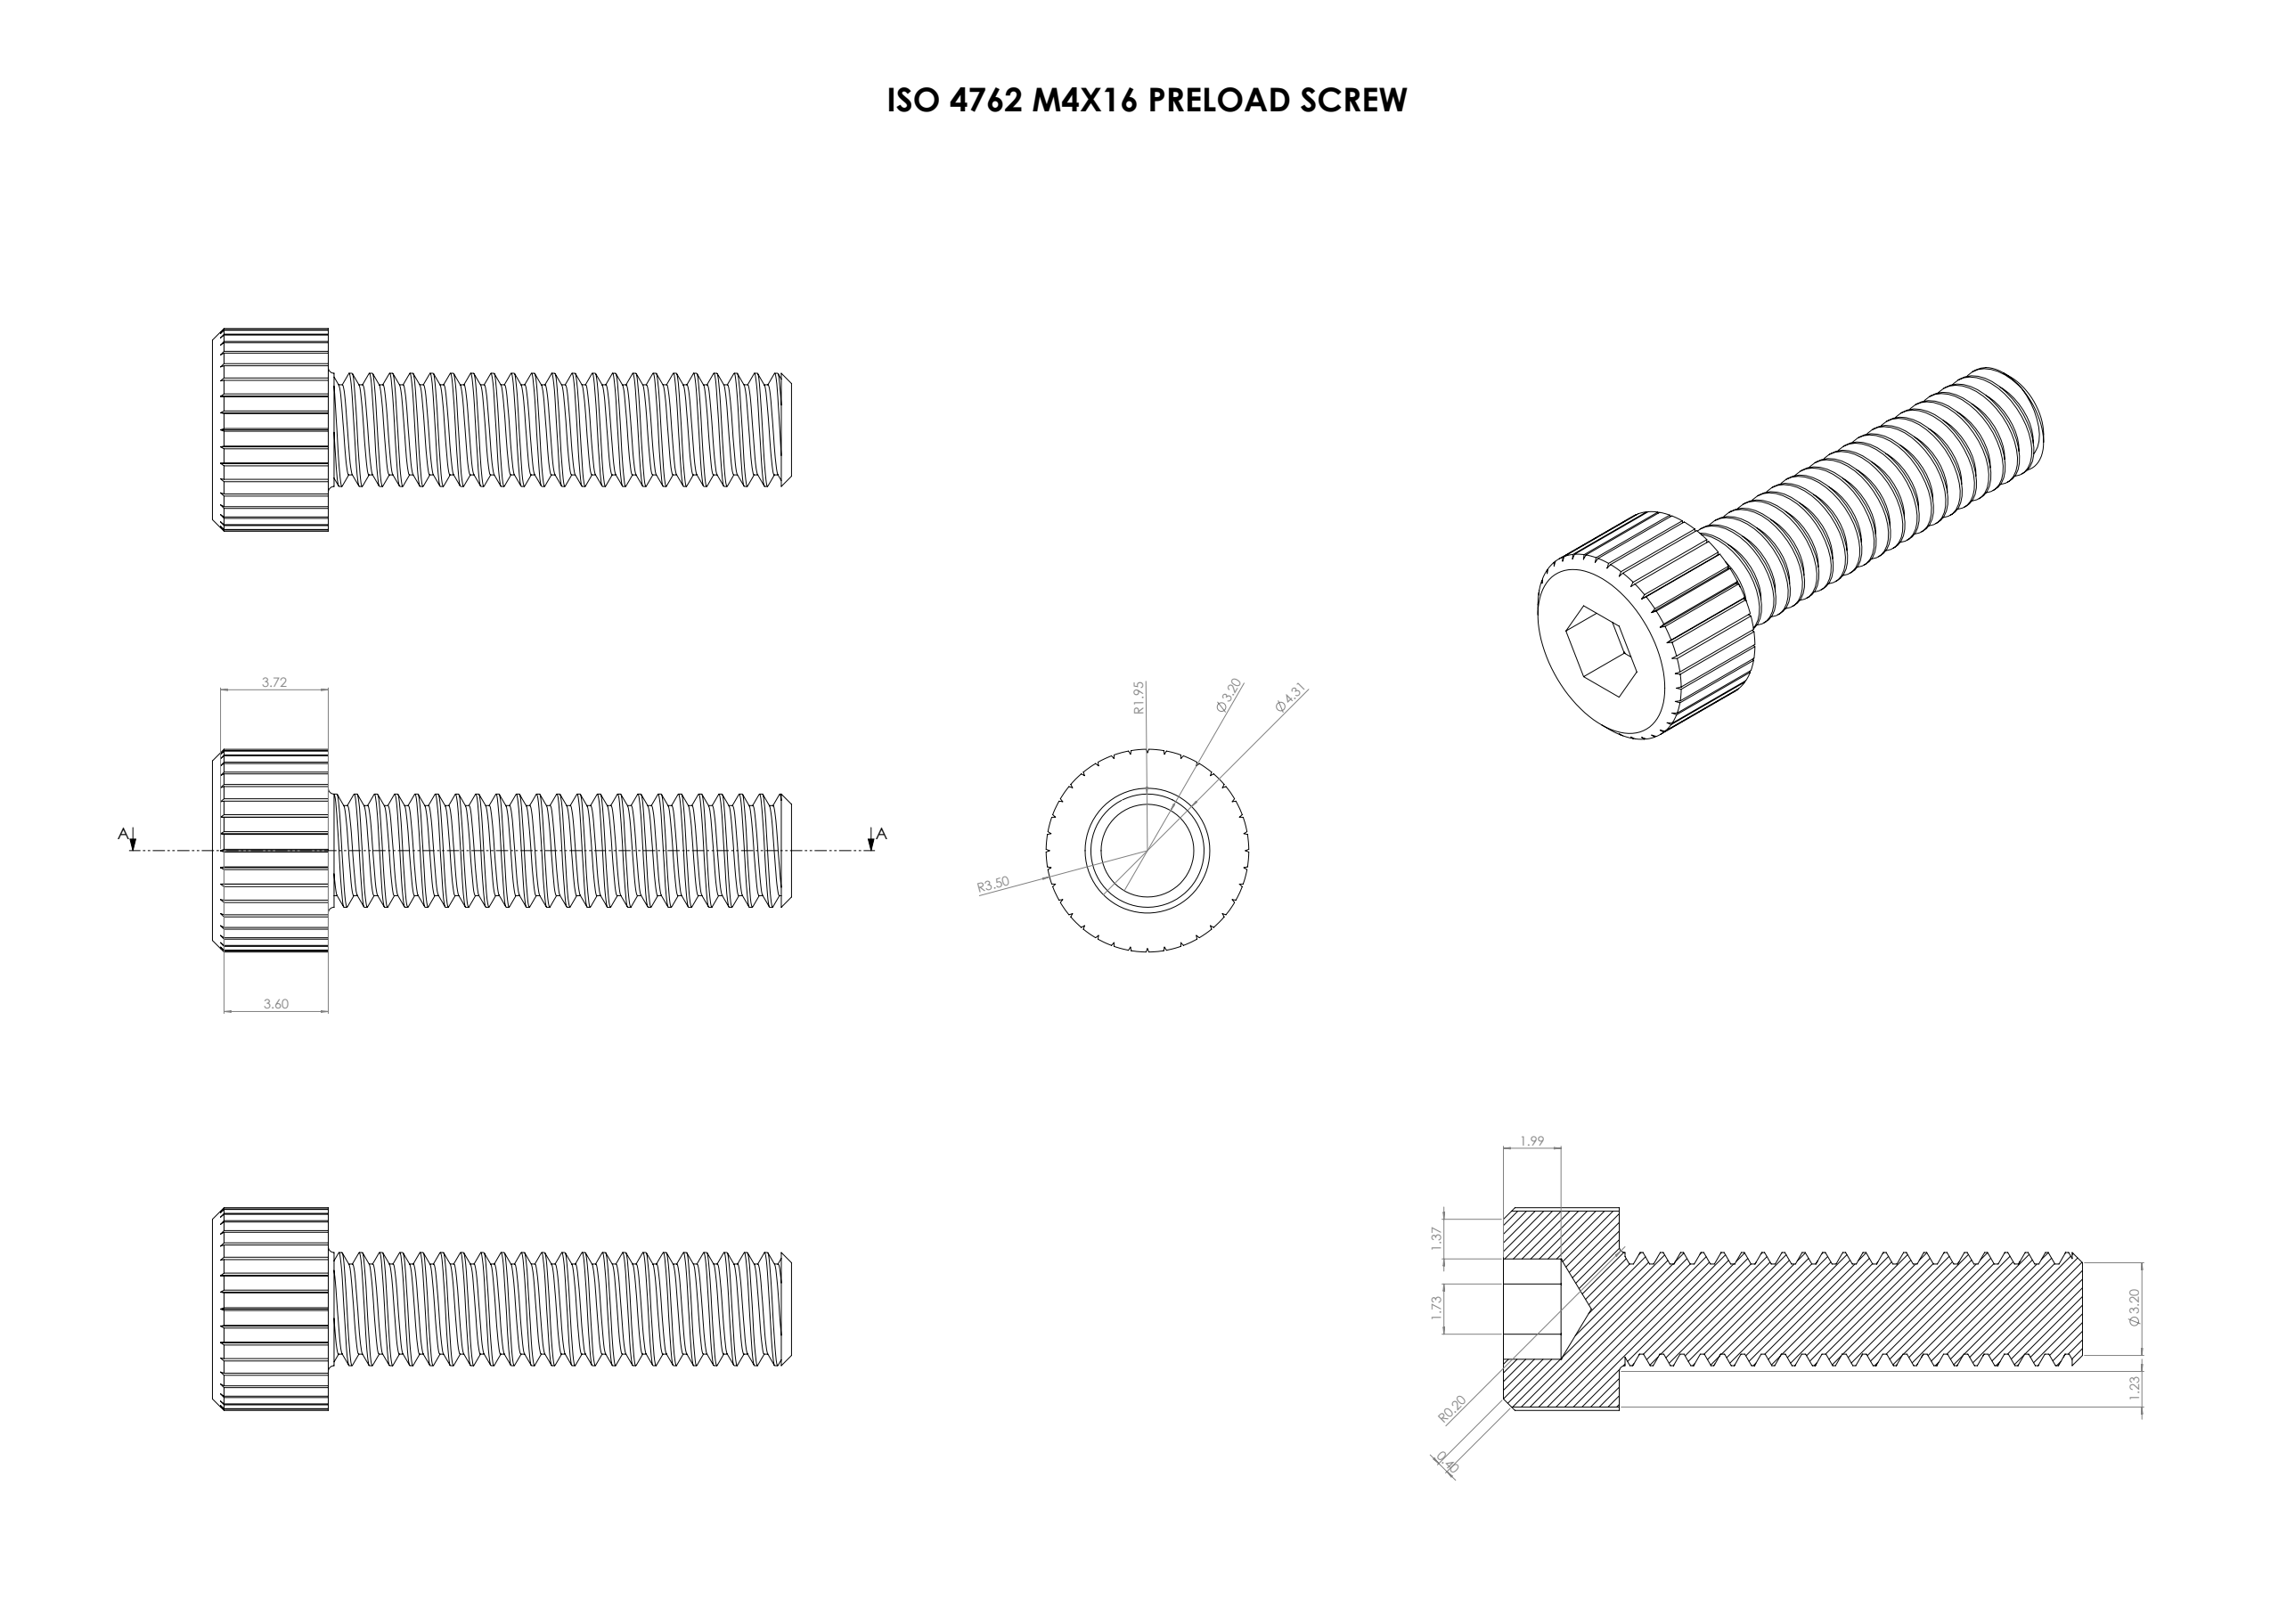
ISO-10303-21;
HEADER;
/* Generated by software containing ST-Developer
 * from STEP Tools, Inc. (www.steptools.com) 
 */

FILE_DESCRIPTION(
/* description */ (''),
/* implementation_level */ '2;1');

FILE_NAME(
/* name */ 
'11_ISO_4762_M4x16_Preload_Screw.step',
/* time_stamp */ '2026-10-20T10:06:23-07:00',
/* author */ (''),
/* organization */ (''),
/* preprocessor_version */ 'ST-DEVELOPER v20.2',
/* originating_system */ 'Autodesk Translation Framework v15.15.0.0',
/* authorisation */ '');

FILE_SCHEMA (('AUTOMOTIVE_DESIGN { 1 0 10303 214 3 1 1 }'));
ENDSEC;

DATA;
#10=MECHANICAL_DESIGN_GEOMETRIC_PRESENTATION_REPRESENTATION('',(#472),#38611);
#252=(
BOUNDED_CURVE()
B_SPLINE_CURVE(2,(#35550,#35551,#35552),.UNSPECIFIED.,.F.,.F.)
B_SPLINE_CURVE_WITH_KNOTS((3,3),(0.,0.00349669843186121),.UNSPECIFIED.)
CURVE()
GEOMETRIC_REPRESENTATION_ITEM()
RATIONAL_B_SPLINE_CURVE((1.,1.00004723091695,1.))
REPRESENTATION_ITEM('')
);
#253=(
BOUNDED_CURVE()
B_SPLINE_CURVE(2,(#35554,#35555,#35556),.UNSPECIFIED.,.F.,.F.)
B_SPLINE_CURVE_WITH_KNOTS((3,3),(0.,0.00349669843186122),.UNSPECIFIED.)
CURVE()
GEOMETRIC_REPRESENTATION_ITEM()
RATIONAL_B_SPLINE_CURVE((1.,1.00004723094136,1.))
REPRESENTATION_ITEM('')
);
#254=(
BOUNDED_CURVE()
B_SPLINE_CURVE(2,(#35559,#35560,#35561),.UNSPECIFIED.,.F.,.F.)
B_SPLINE_CURVE_WITH_KNOTS((3,3),(0.,0.00349669843186136),.UNSPECIFIED.)
CURVE()
GEOMETRIC_REPRESENTATION_ITEM()
RATIONAL_B_SPLINE_CURVE((1.,1.00004723092143,1.))
REPRESENTATION_ITEM('')
);
#255=(
BOUNDED_CURVE()
B_SPLINE_CURVE(2,(#35563,#35564,#35565),.UNSPECIFIED.,.F.,.F.)
B_SPLINE_CURVE_WITH_KNOTS((3,3),(0.,0.00349669843186135),.UNSPECIFIED.)
CURVE()
GEOMETRIC_REPRESENTATION_ITEM()
RATIONAL_B_SPLINE_CURVE((1.,1.00004723092493,1.))
REPRESENTATION_ITEM('')
);
#256=(
BOUNDED_CURVE()
B_SPLINE_CURVE(2,(#35568,#35569,#35570),.UNSPECIFIED.,.F.,.F.)
B_SPLINE_CURVE_WITH_KNOTS((3,3),(0.,0.00349669843186138),.UNSPECIFIED.)
CURVE()
GEOMETRIC_REPRESENTATION_ITEM()
RATIONAL_B_SPLINE_CURVE((1.,1.00004723092744,1.))
REPRESENTATION_ITEM('')
);
#257=(
BOUNDED_CURVE()
B_SPLINE_CURVE(2,(#35572,#35573,#35574),.UNSPECIFIED.,.F.,.F.)
B_SPLINE_CURVE_WITH_KNOTS((3,3),(0.,0.00349669843186141),.UNSPECIFIED.)
CURVE()
GEOMETRIC_REPRESENTATION_ITEM()
RATIONAL_B_SPLINE_CURVE((1.,1.00004723090855,1.))
REPRESENTATION_ITEM('')
);
#258=(
BOUNDED_CURVE()
B_SPLINE_CURVE(2,(#35577,#35578,#35579),.UNSPECIFIED.,.F.,.F.)
B_SPLINE_CURVE_WITH_KNOTS((3,3),(0.,0.0034966984318615),.UNSPECIFIED.)
CURVE()
GEOMETRIC_REPRESENTATION_ITEM()
RATIONAL_B_SPLINE_CURVE((1.,1.00004723094741,1.))
REPRESENTATION_ITEM('')
);
#259=(
BOUNDED_CURVE()
B_SPLINE_CURVE(2,(#35581,#35582,#35583),.UNSPECIFIED.,.F.,.F.)
B_SPLINE_CURVE_WITH_KNOTS((3,3),(0.,0.00349669843186142),.UNSPECIFIED.)
CURVE()
GEOMETRIC_REPRESENTATION_ITEM()
RATIONAL_B_SPLINE_CURVE((1.,1.00004723090666,1.))
REPRESENTATION_ITEM('')
);
#260=(
BOUNDED_CURVE()
B_SPLINE_CURVE(2,(#35586,#35587,#35588),.UNSPECIFIED.,.F.,.F.)
B_SPLINE_CURVE_WITH_KNOTS((3,3),(0.,0.00349669843186135),.UNSPECIFIED.)
CURVE()
GEOMETRIC_REPRESENTATION_ITEM()
RATIONAL_B_SPLINE_CURVE((1.,1.0000472309119,1.))
REPRESENTATION_ITEM('')
);
#261=(
BOUNDED_CURVE()
B_SPLINE_CURVE(2,(#35590,#35591,#35592),.UNSPECIFIED.,.F.,.F.)
B_SPLINE_CURVE_WITH_KNOTS((3,3),(0.,0.00349669843186137),.UNSPECIFIED.)
CURVE()
GEOMETRIC_REPRESENTATION_ITEM()
RATIONAL_B_SPLINE_CURVE((1.,1.00004723093721,1.))
REPRESENTATION_ITEM('')
);
#262=(
BOUNDED_CURVE()
B_SPLINE_CURVE(2,(#35595,#35596,#35597),.UNSPECIFIED.,.F.,.F.)
B_SPLINE_CURVE_WITH_KNOTS((3,3),(0.,0.00349669843186128),.UNSPECIFIED.)
CURVE()
GEOMETRIC_REPRESENTATION_ITEM()
RATIONAL_B_SPLINE_CURVE((1.,1.00004723093599,1.))
REPRESENTATION_ITEM('')
);
#263=(
BOUNDED_CURVE()
B_SPLINE_CURVE(2,(#35599,#35600,#35601),.UNSPECIFIED.,.F.,.F.)
B_SPLINE_CURVE_WITH_KNOTS((3,3),(0.,0.00349669843186128),.UNSPECIFIED.)
CURVE()
GEOMETRIC_REPRESENTATION_ITEM()
RATIONAL_B_SPLINE_CURVE((1.,1.00004723092625,1.))
REPRESENTATION_ITEM('')
);
#264=(
BOUNDED_CURVE()
B_SPLINE_CURVE(2,(#35672,#35673,#35674),.UNSPECIFIED.,.F.,.F.)
B_SPLINE_CURVE_WITH_KNOTS((3,3),(0.0420809670913651,0.0588848364681992),
 .UNSPECIFIED.)
CURVE()
GEOMETRIC_REPRESENTATION_ITEM()
RATIONAL_B_SPLINE_CURVE((1.00087707567824,1.00061365578614,1.))
REPRESENTATION_ITEM('')
);
#265=(
BOUNDED_CURVE()
B_SPLINE_CURVE(2,(#35679,#35680,#35681),.UNSPECIFIED.,.F.,.F.)
B_SPLINE_CURVE_WITH_KNOTS((3,3),(0.,0.0168038693768593),.UNSPECIFIED.)
CURVE()
GEOMETRIC_REPRESENTATION_ITEM()
RATIONAL_B_SPLINE_CURVE((1.,1.00061365578593,1.00087707567795))
REPRESENTATION_ITEM('')
);
#266=(
BOUNDED_CURVE()
B_SPLINE_CURVE(2,(#35686,#35687,#35688),.UNSPECIFIED.,.F.,.F.)
B_SPLINE_CURVE_WITH_KNOTS((3,3),(0.0420809670913399,0.0588848364681993),
 .UNSPECIFIED.)
CURVE()
GEOMETRIC_REPRESENTATION_ITEM()
RATIONAL_B_SPLINE_CURVE((1.00087707567746,1.00061365578559,1.))
REPRESENTATION_ITEM('')
);
#267=(
BOUNDED_CURVE()
B_SPLINE_CURVE(2,(#35693,#35694,#35695),.UNSPECIFIED.,.F.,.F.)
B_SPLINE_CURVE_WITH_KNOTS((3,3),(0.,0.0168038693768394),.UNSPECIFIED.)
CURVE()
GEOMETRIC_REPRESENTATION_ITEM()
RATIONAL_B_SPLINE_CURVE((1.,1.00061365578594,1.00087707567797))
REPRESENTATION_ITEM('')
);
#268=(
BOUNDED_CURVE()
B_SPLINE_CURVE(2,(#35700,#35701,#35702),.UNSPECIFIED.,.F.,.F.)
B_SPLINE_CURVE_WITH_KNOTS((3,3),(0.0420809670913626,0.0588848364681992),
 .UNSPECIFIED.)
CURVE()
GEOMETRIC_REPRESENTATION_ITEM()
RATIONAL_B_SPLINE_CURVE((1.00087707567775,1.00061365578579,1.))
REPRESENTATION_ITEM('')
);
#269=(
BOUNDED_CURVE()
B_SPLINE_CURVE(2,(#35707,#35708,#35709),.UNSPECIFIED.,.F.,.F.)
B_SPLINE_CURVE_WITH_KNOTS((3,3),(0.,0.0168038693768627),.UNSPECIFIED.)
CURVE()
GEOMETRIC_REPRESENTATION_ITEM()
RATIONAL_B_SPLINE_CURVE((1.,1.00061365578587,1.00087707567786))
REPRESENTATION_ITEM('')
);
#270=(
BOUNDED_CURVE()
B_SPLINE_CURVE(2,(#35714,#35715,#35716),.UNSPECIFIED.,.F.,.F.)
B_SPLINE_CURVE_WITH_KNOTS((3,3),(0.042080967091394,0.0588848364681993),
 .UNSPECIFIED.)
CURVE()
GEOMETRIC_REPRESENTATION_ITEM()
RATIONAL_B_SPLINE_CURVE((1.00087707567792,1.00061365578591,1.))
REPRESENTATION_ITEM('')
);
#271=(
BOUNDED_CURVE()
B_SPLINE_CURVE(2,(#35721,#35722,#35723),.UNSPECIFIED.,.F.,.F.)
B_SPLINE_CURVE_WITH_KNOTS((3,3),(0.,0.0168038693768566),.UNSPECIFIED.)
CURVE()
GEOMETRIC_REPRESENTATION_ITEM()
RATIONAL_B_SPLINE_CURVE((1.,1.00061365578555,1.0008770756774))
REPRESENTATION_ITEM('')
);
#272=(
BOUNDED_CURVE()
B_SPLINE_CURVE(2,(#35728,#35729,#35730),.UNSPECIFIED.,.F.,.F.)
B_SPLINE_CURVE_WITH_KNOTS((3,3),(0.0420809670913884,0.0588848364681993),
 .UNSPECIFIED.)
CURVE()
GEOMETRIC_REPRESENTATION_ITEM()
RATIONAL_B_SPLINE_CURVE((1.00087707567863,1.0006136557864,1.))
REPRESENTATION_ITEM('')
);
#273=(
BOUNDED_CURVE()
B_SPLINE_CURVE(2,(#35735,#35736,#35737),.UNSPECIFIED.,.F.,.F.)
B_SPLINE_CURVE_WITH_KNOTS((3,3),(0.,0.0168038693768499),.UNSPECIFIED.)
CURVE()
GEOMETRIC_REPRESENTATION_ITEM()
RATIONAL_B_SPLINE_CURVE((1.,1.00061365578631,1.00087707567849))
REPRESENTATION_ITEM('')
);
#274=(
BOUNDED_CURVE()
B_SPLINE_CURVE(2,(#35742,#35743,#35744),.UNSPECIFIED.,.F.,.F.)
B_SPLINE_CURVE_WITH_KNOTS((3,3),(0.0420809670913347,0.0588848364681992),
 .UNSPECIFIED.)
CURVE()
GEOMETRIC_REPRESENTATION_ITEM()
RATIONAL_B_SPLINE_CURVE((1.00087707567759,1.00061365578568,1.))
REPRESENTATION_ITEM('')
);
#275=(
BOUNDED_CURVE()
B_SPLINE_CURVE(2,(#35749,#35750,#35751),.UNSPECIFIED.,.F.,.F.)
B_SPLINE_CURVE_WITH_KNOTS((3,3),(0.,0.0168038693768258),.UNSPECIFIED.)
CURVE()
GEOMETRIC_REPRESENTATION_ITEM()
RATIONAL_B_SPLINE_CURVE((1.,1.00061365578592,1.00087707567793))
REPRESENTATION_ITEM('')
);
#276=(
BOUNDED_CURVE()
B_SPLINE_CURVE(2,(#35756,#35757,#35758),.UNSPECIFIED.,.F.,.F.)
B_SPLINE_CURVE_WITH_KNOTS((3,3),(0.0420809670913505,0.0588848364681993),
 .UNSPECIFIED.)
CURVE()
GEOMETRIC_REPRESENTATION_ITEM()
RATIONAL_B_SPLINE_CURVE((1.00087707567804,1.00061365578599,1.))
REPRESENTATION_ITEM('')
);
#277=(
BOUNDED_CURVE()
B_SPLINE_CURVE(2,(#35763,#35764,#35765),.UNSPECIFIED.,.F.,.F.)
B_SPLINE_CURVE_WITH_KNOTS((3,3),(0.,0.0168038693768362),.UNSPECIFIED.)
CURVE()
GEOMETRIC_REPRESENTATION_ITEM()
RATIONAL_B_SPLINE_CURVE((1.,1.00061365578568,1.00087707567759))
REPRESENTATION_ITEM('')
);
#278=(
BOUNDED_CURVE()
B_SPLINE_CURVE(2,(#35770,#35771,#35772),.UNSPECIFIED.,.F.,.F.)
B_SPLINE_CURVE_WITH_KNOTS((3,3),(0.0420809670913562,0.0588848364681992),
 .UNSPECIFIED.)
CURVE()
GEOMETRIC_REPRESENTATION_ITEM()
RATIONAL_B_SPLINE_CURVE((1.00087707567804,1.00061365578599,1.))
REPRESENTATION_ITEM('')
);
#279=(
BOUNDED_CURVE()
B_SPLINE_CURVE(2,(#35777,#35778,#35779),.UNSPECIFIED.,.F.,.F.)
B_SPLINE_CURVE_WITH_KNOTS((3,3),(0.,0.016803869376823),.UNSPECIFIED.)
CURVE()
GEOMETRIC_REPRESENTATION_ITEM()
RATIONAL_B_SPLINE_CURVE((1.,1.00061365578592,1.00087707567794))
REPRESENTATION_ITEM('')
);
#280=(
BOUNDED_CURVE()
B_SPLINE_CURVE(2,(#35784,#35785,#35786),.UNSPECIFIED.,.F.,.F.)
B_SPLINE_CURVE_WITH_KNOTS((3,3),(0.04208096709136,0.0588848364681992),
 .UNSPECIFIED.)
CURVE()
GEOMETRIC_REPRESENTATION_ITEM()
RATIONAL_B_SPLINE_CURVE((1.00087707567819,1.0006136557861,1.))
REPRESENTATION_ITEM('')
);
#281=(
BOUNDED_CURVE()
B_SPLINE_CURVE(2,(#35791,#35792,#35793),.UNSPECIFIED.,.F.,.F.)
B_SPLINE_CURVE_WITH_KNOTS((3,3),(0.,0.0168038693767949),.UNSPECIFIED.)
CURVE()
GEOMETRIC_REPRESENTATION_ITEM()
RATIONAL_B_SPLINE_CURVE((1.,1.00061365578653,1.00087707567881))
REPRESENTATION_ITEM('')
);
#282=(
BOUNDED_CURVE()
B_SPLINE_CURVE(2,(#35798,#35799,#35800),.UNSPECIFIED.,.F.,.F.)
B_SPLINE_CURVE_WITH_KNOTS((3,3),(0.0420809670913836,0.0588848364681992),
 .UNSPECIFIED.)
CURVE()
GEOMETRIC_REPRESENTATION_ITEM()
RATIONAL_B_SPLINE_CURVE((1.00087707567816,1.00061365578608,1.))
REPRESENTATION_ITEM('')
);
#283=(
BOUNDED_CURVE()
B_SPLINE_CURVE(2,(#35805,#35806,#35807),.UNSPECIFIED.,.F.,.F.)
B_SPLINE_CURVE_WITH_KNOTS((3,3),(0.,0.0168038693768179),.UNSPECIFIED.)
CURVE()
GEOMETRIC_REPRESENTATION_ITEM()
RATIONAL_B_SPLINE_CURVE((1.,1.00061365578613,1.00087707567823))
REPRESENTATION_ITEM('')
);
#284=(
BOUNDED_CURVE()
B_SPLINE_CURVE(2,(#35812,#35813,#35814),.UNSPECIFIED.,.F.,.F.)
B_SPLINE_CURVE_WITH_KNOTS((3,3),(0.0420809670913823,0.0588848364681992),
 .UNSPECIFIED.)
CURVE()
GEOMETRIC_REPRESENTATION_ITEM()
RATIONAL_B_SPLINE_CURVE((1.00087707567815,1.00061365578607,1.))
REPRESENTATION_ITEM('')
);
#285=(
BOUNDED_CURVE()
B_SPLINE_CURVE(2,(#35819,#35820,#35821),.UNSPECIFIED.,.F.,.F.)
B_SPLINE_CURVE_WITH_KNOTS((3,3),(0.,0.0168038693768011),.UNSPECIFIED.)
CURVE()
GEOMETRIC_REPRESENTATION_ITEM()
RATIONAL_B_SPLINE_CURVE((1.,1.00061365578643,1.00087707567867))
REPRESENTATION_ITEM('')
);
#286=(
BOUNDED_CURVE()
B_SPLINE_CURVE(2,(#35826,#35827,#35828),.UNSPECIFIED.,.F.,.F.)
B_SPLINE_CURVE_WITH_KNOTS((3,3),(0.0420809670914,0.0588848364681992),
 .UNSPECIFIED.)
CURVE()
GEOMETRIC_REPRESENTATION_ITEM()
RATIONAL_B_SPLINE_CURVE((1.00087707567851,1.00061365578632,1.))
REPRESENTATION_ITEM('')
);
#287=(
BOUNDED_CURVE()
B_SPLINE_CURVE(2,(#35833,#35834,#35835),.UNSPECIFIED.,.F.,.F.)
B_SPLINE_CURVE_WITH_KNOTS((3,3),(0.,0.016803869376813),.UNSPECIFIED.)
CURVE()
GEOMETRIC_REPRESENTATION_ITEM()
RATIONAL_B_SPLINE_CURVE((1.,1.00061365578622,1.00087707567836))
REPRESENTATION_ITEM('')
);
#288=(
BOUNDED_CURVE()
B_SPLINE_CURVE(2,(#35840,#35841,#35842),.UNSPECIFIED.,.F.,.F.)
B_SPLINE_CURVE_WITH_KNOTS((3,3),(0.0420809670913641,0.0588848364681993),
 .UNSPECIFIED.)
CURVE()
GEOMETRIC_REPRESENTATION_ITEM()
RATIONAL_B_SPLINE_CURVE((1.0008770756778,1.00061365578582,1.))
REPRESENTATION_ITEM('')
);
#289=(
BOUNDED_CURVE()
B_SPLINE_CURVE(2,(#35847,#35848,#35849),.UNSPECIFIED.,.F.,.F.)
B_SPLINE_CURVE_WITH_KNOTS((3,3),(0.,0.0168038693768258),.UNSPECIFIED.)
CURVE()
GEOMETRIC_REPRESENTATION_ITEM()
RATIONAL_B_SPLINE_CURVE((1.,1.00061365578608,1.00087707567816))
REPRESENTATION_ITEM('')
);
#290=(
BOUNDED_CURVE()
B_SPLINE_CURVE(2,(#35854,#35855,#35856),.UNSPECIFIED.,.F.,.F.)
B_SPLINE_CURVE_WITH_KNOTS((3,3),(0.0420809670913328,0.0588848364681992),
 .UNSPECIFIED.)
CURVE()
GEOMETRIC_REPRESENTATION_ITEM()
RATIONAL_B_SPLINE_CURVE((1.00087707567803,1.00061365578599,1.))
REPRESENTATION_ITEM('')
);
#291=(
BOUNDED_CURVE()
B_SPLINE_CURVE(2,(#35861,#35862,#35863),.UNSPECIFIED.,.F.,.F.)
B_SPLINE_CURVE_WITH_KNOTS((3,3),(0.,0.016803869376812),.UNSPECIFIED.)
CURVE()
GEOMETRIC_REPRESENTATION_ITEM()
RATIONAL_B_SPLINE_CURVE((1.,1.00061365578602,1.00087707567807))
REPRESENTATION_ITEM('')
);
#292=(
BOUNDED_CURVE()
B_SPLINE_CURVE(2,(#35868,#35869,#35870),.UNSPECIFIED.,.F.,.F.)
B_SPLINE_CURVE_WITH_KNOTS((3,3),(0.0420809670913778,0.0588848364681992),
 .UNSPECIFIED.)
CURVE()
GEOMETRIC_REPRESENTATION_ITEM()
RATIONAL_B_SPLINE_CURVE((1.0008770756785,1.00061365578631,1.))
REPRESENTATION_ITEM('')
);
#293=(
BOUNDED_CURVE()
B_SPLINE_CURVE(2,(#35875,#35876,#35877),.UNSPECIFIED.,.F.,.F.)
B_SPLINE_CURVE_WITH_KNOTS((3,3),(0.,0.0168038693768374),.UNSPECIFIED.)
CURVE()
GEOMETRIC_REPRESENTATION_ITEM()
RATIONAL_B_SPLINE_CURVE((1.,1.00061365578616,1.00087707567828))
REPRESENTATION_ITEM('')
);
#294=(
BOUNDED_CURVE()
B_SPLINE_CURVE(2,(#35882,#35883,#35884),.UNSPECIFIED.,.F.,.F.)
B_SPLINE_CURVE_WITH_KNOTS((3,3),(0.0420809670913638,0.0588848364681993),
 .UNSPECIFIED.)
CURVE()
GEOMETRIC_REPRESENTATION_ITEM()
RATIONAL_B_SPLINE_CURVE((1.00087707567787,1.00061365578588,1.))
REPRESENTATION_ITEM('')
);
#295=(
BOUNDED_CURVE()
B_SPLINE_CURVE(2,(#35889,#35890,#35891),.UNSPECIFIED.,.F.,.F.)
B_SPLINE_CURVE_WITH_KNOTS((3,3),(0.,0.0168038693768215),.UNSPECIFIED.)
CURVE()
GEOMETRIC_REPRESENTATION_ITEM()
RATIONAL_B_SPLINE_CURVE((1.,1.00061365578602,1.00087707567808))
REPRESENTATION_ITEM('')
);
#296=(
BOUNDED_CURVE()
B_SPLINE_CURVE(2,(#35896,#35897,#35898),.UNSPECIFIED.,.F.,.F.)
B_SPLINE_CURVE_WITH_KNOTS((3,3),(0.0420809670913305,0.0588848364681993),
 .UNSPECIFIED.)
CURVE()
GEOMETRIC_REPRESENTATION_ITEM()
RATIONAL_B_SPLINE_CURVE((1.00087707567765,1.00061365578572,1.))
REPRESENTATION_ITEM('')
);
#297=(
BOUNDED_CURVE()
B_SPLINE_CURVE(2,(#35903,#35904,#35905),.UNSPECIFIED.,.F.,.F.)
B_SPLINE_CURVE_WITH_KNOTS((3,3),(0.,0.0168038693768224),.UNSPECIFIED.)
CURVE()
GEOMETRIC_REPRESENTATION_ITEM()
RATIONAL_B_SPLINE_CURVE((1.,1.00061365578599,1.00087707567803))
REPRESENTATION_ITEM('')
);
#298=(
BOUNDED_CURVE()
B_SPLINE_CURVE(2,(#35910,#35911,#35912),.UNSPECIFIED.,.F.,.F.)
B_SPLINE_CURVE_WITH_KNOTS((3,3),(0.0420809670913736,0.0588848364681993),
 .UNSPECIFIED.)
CURVE()
GEOMETRIC_REPRESENTATION_ITEM()
RATIONAL_B_SPLINE_CURVE((1.00087707567727,1.00061365578546,1.))
REPRESENTATION_ITEM('')
);
#299=(
BOUNDED_CURVE()
B_SPLINE_CURVE(2,(#35917,#35918,#35919),.UNSPECIFIED.,.F.,.F.)
B_SPLINE_CURVE_WITH_KNOTS((3,3),(0.,0.0168038693768305),.UNSPECIFIED.)
CURVE()
GEOMETRIC_REPRESENTATION_ITEM()
RATIONAL_B_SPLINE_CURVE((1.,1.00061365578611,1.00087707567821))
REPRESENTATION_ITEM('')
);
#300=(
BOUNDED_CURVE()
B_SPLINE_CURVE(2,(#35924,#35925,#35926),.UNSPECIFIED.,.F.,.F.)
B_SPLINE_CURVE_WITH_KNOTS((3,3),(0.042080967091357,0.0588848364681993),
 .UNSPECIFIED.)
CURVE()
GEOMETRIC_REPRESENTATION_ITEM()
RATIONAL_B_SPLINE_CURVE((1.00087707567817,1.00061365578609,1.))
REPRESENTATION_ITEM('')
);
#301=(
BOUNDED_CURVE()
B_SPLINE_CURVE(2,(#35931,#35932,#35933),.UNSPECIFIED.,.F.,.F.)
B_SPLINE_CURVE_WITH_KNOTS((3,3),(0.,0.0168038693768215),.UNSPECIFIED.)
CURVE()
GEOMETRIC_REPRESENTATION_ITEM()
RATIONAL_B_SPLINE_CURVE((1.,1.00061365578616,1.00087707567828))
REPRESENTATION_ITEM('')
);
#302=(
BOUNDED_CURVE()
B_SPLINE_CURVE(2,(#35938,#35939,#35940),.UNSPECIFIED.,.F.,.F.)
B_SPLINE_CURVE_WITH_KNOTS((3,3),(0.04208096709137,0.0588848364681993),
 .UNSPECIFIED.)
CURVE()
GEOMETRIC_REPRESENTATION_ITEM()
RATIONAL_B_SPLINE_CURVE((1.00087707567792,1.00061365578591,1.))
REPRESENTATION_ITEM('')
);
#303=(
BOUNDED_CURVE()
B_SPLINE_CURVE(2,(#35945,#35946,#35947),.UNSPECIFIED.,.F.,.F.)
B_SPLINE_CURVE_WITH_KNOTS((3,3),(0.,0.0168038693768075),.UNSPECIFIED.)
CURVE()
GEOMETRIC_REPRESENTATION_ITEM()
RATIONAL_B_SPLINE_CURVE((1.,1.00061365578628,1.00087707567845))
REPRESENTATION_ITEM('')
);
#304=(
BOUNDED_CURVE()
B_SPLINE_CURVE(2,(#35952,#35953,#35954),.UNSPECIFIED.,.F.,.F.)
B_SPLINE_CURVE_WITH_KNOTS((3,3),(0.0420809670913788,0.0588848364681993),
 .UNSPECIFIED.)
CURVE()
GEOMETRIC_REPRESENTATION_ITEM()
RATIONAL_B_SPLINE_CURVE((1.00087707567806,1.00061365578601,1.))
REPRESENTATION_ITEM('')
);
#305=(
BOUNDED_CURVE()
B_SPLINE_CURVE(2,(#35959,#35960,#35961),.UNSPECIFIED.,.F.,.F.)
B_SPLINE_CURVE_WITH_KNOTS((3,3),(0.,0.0168038693768069),.UNSPECIFIED.)
CURVE()
GEOMETRIC_REPRESENTATION_ITEM()
RATIONAL_B_SPLINE_CURVE((1.,1.00061365578667,1.000877075679))
REPRESENTATION_ITEM('')
);
#306=(
BOUNDED_CURVE()
B_SPLINE_CURVE(2,(#35966,#35967,#35968),.UNSPECIFIED.,.F.,.F.)
B_SPLINE_CURVE_WITH_KNOTS((3,3),(0.0420809670913639,0.0588848364681993),
 .UNSPECIFIED.)
CURVE()
GEOMETRIC_REPRESENTATION_ITEM()
RATIONAL_B_SPLINE_CURVE((1.00087707567811,1.00061365578604,1.))
REPRESENTATION_ITEM('')
);
#307=(
BOUNDED_CURVE()
B_SPLINE_CURVE(2,(#35973,#35974,#35975),.UNSPECIFIED.,.F.,.F.)
B_SPLINE_CURVE_WITH_KNOTS((3,3),(0.,0.0168038693768441),.UNSPECIFIED.)
CURVE()
GEOMETRIC_REPRESENTATION_ITEM()
RATIONAL_B_SPLINE_CURVE((1.,1.00061365578625,1.0008770756784))
REPRESENTATION_ITEM('')
);
#308=(
BOUNDED_CURVE()
B_SPLINE_CURVE(2,(#35980,#35981,#35982),.UNSPECIFIED.,.F.,.F.)
B_SPLINE_CURVE_WITH_KNOTS((3,3),(0.0420809670913765,0.0588848364681993),
 .UNSPECIFIED.)
CURVE()
GEOMETRIC_REPRESENTATION_ITEM()
RATIONAL_B_SPLINE_CURVE((1.00087707567789,1.00061365578589,1.))
REPRESENTATION_ITEM('')
);
#309=(
BOUNDED_CURVE()
B_SPLINE_CURVE(2,(#35987,#35988,#35989),.UNSPECIFIED.,.F.,.F.)
B_SPLINE_CURVE_WITH_KNOTS((3,3),(0.,0.016803869376822),.UNSPECIFIED.)
CURVE()
GEOMETRIC_REPRESENTATION_ITEM()
RATIONAL_B_SPLINE_CURVE((1.,1.00061365578656,1.00087707567884))
REPRESENTATION_ITEM('')
);
#310=(
BOUNDED_CURVE()
B_SPLINE_CURVE(2,(#35994,#35995,#35996),.UNSPECIFIED.,.F.,.F.)
B_SPLINE_CURVE_WITH_KNOTS((3,3),(0.0420809670913437,0.0588848364681993),
 .UNSPECIFIED.)
CURVE()
GEOMETRIC_REPRESENTATION_ITEM()
RATIONAL_B_SPLINE_CURVE((1.00087707567775,1.00061365578579,1.))
REPRESENTATION_ITEM('')
);
#311=(
BOUNDED_CURVE()
B_SPLINE_CURVE(2,(#36001,#36002,#36003),.UNSPECIFIED.,.F.,.F.)
B_SPLINE_CURVE_WITH_KNOTS((3,3),(0.,0.0168038693768237),.UNSPECIFIED.)
CURVE()
GEOMETRIC_REPRESENTATION_ITEM()
RATIONAL_B_SPLINE_CURVE((1.,1.00061365578586,1.00087707567785))
REPRESENTATION_ITEM('')
);
#312=(
BOUNDED_CURVE()
B_SPLINE_CURVE(2,(#36008,#36009,#36010),.UNSPECIFIED.,.F.,.F.)
B_SPLINE_CURVE_WITH_KNOTS((3,3),(0.0420809670913633,0.0588848364681993),
 .UNSPECIFIED.)
CURVE()
GEOMETRIC_REPRESENTATION_ITEM()
RATIONAL_B_SPLINE_CURVE((1.00087707567797,1.00061365578594,1.))
REPRESENTATION_ITEM('')
);
#313=(
BOUNDED_CURVE()
B_SPLINE_CURVE(2,(#36015,#36016,#36017),.UNSPECIFIED.,.F.,.F.)
B_SPLINE_CURVE_WITH_KNOTS((3,3),(0.,0.0168038693768391),.UNSPECIFIED.)
CURVE()
GEOMETRIC_REPRESENTATION_ITEM()
RATIONAL_B_SPLINE_CURVE((1.,1.00061365578625,1.0008770756784))
REPRESENTATION_ITEM('')
);
#314=(
BOUNDED_CURVE()
B_SPLINE_CURVE(2,(#36022,#36023,#36024),.UNSPECIFIED.,.F.,.F.)
B_SPLINE_CURVE_WITH_KNOTS((3,3),(0.0420809670913792,0.0588848364681992),
 .UNSPECIFIED.)
CURVE()
GEOMETRIC_REPRESENTATION_ITEM()
RATIONAL_B_SPLINE_CURVE((1.00087707567848,1.0006136557863,1.))
REPRESENTATION_ITEM('')
);
#315=(
BOUNDED_CURVE()
B_SPLINE_CURVE(2,(#36029,#36030,#36031),.UNSPECIFIED.,.F.,.F.)
B_SPLINE_CURVE_WITH_KNOTS((3,3),(0.,0.0168038693768203),.UNSPECIFIED.)
CURVE()
GEOMETRIC_REPRESENTATION_ITEM()
RATIONAL_B_SPLINE_CURVE((1.,1.00061365578598,1.00087707567802))
REPRESENTATION_ITEM('')
);
#316=(
BOUNDED_CURVE()
B_SPLINE_CURVE(2,(#36036,#36037,#36038),.UNSPECIFIED.,.F.,.F.)
B_SPLINE_CURVE_WITH_KNOTS((3,3),(0.0420809670913809,0.0588848364681992),
 .UNSPECIFIED.)
CURVE()
GEOMETRIC_REPRESENTATION_ITEM()
RATIONAL_B_SPLINE_CURVE((1.00087707567876,1.0006136557865,1.))
REPRESENTATION_ITEM('')
);
#317=(
BOUNDED_CURVE()
B_SPLINE_CURVE(2,(#36043,#36044,#36045),.UNSPECIFIED.,.F.,.F.)
B_SPLINE_CURVE_WITH_KNOTS((3,3),(0.,0.016803869376822),.UNSPECIFIED.)
CURVE()
GEOMETRIC_REPRESENTATION_ITEM()
RATIONAL_B_SPLINE_CURVE((1.,1.00061365578629,1.00087707567847))
REPRESENTATION_ITEM('')
);
#318=(
BOUNDED_CURVE()
B_SPLINE_CURVE(2,(#36050,#36051,#36052),.UNSPECIFIED.,.F.,.F.)
B_SPLINE_CURVE_WITH_KNOTS((3,3),(0.0420809670913693,0.0588848364681992),
 .UNSPECIFIED.)
CURVE()
GEOMETRIC_REPRESENTATION_ITEM()
RATIONAL_B_SPLINE_CURVE((1.00087707567787,1.00061365578588,1.))
REPRESENTATION_ITEM('')
);
#319=(
BOUNDED_CURVE()
B_SPLINE_CURVE(2,(#36057,#36058,#36059),.UNSPECIFIED.,.F.,.F.)
B_SPLINE_CURVE_WITH_KNOTS((3,3),(0.,0.0168038693768241),.UNSPECIFIED.)
CURVE()
GEOMETRIC_REPRESENTATION_ITEM()
RATIONAL_B_SPLINE_CURVE((1.,1.00061365578674,1.00087707567911))
REPRESENTATION_ITEM('')
);
#320=(
BOUNDED_CURVE()
B_SPLINE_CURVE(2,(#36064,#36065,#36066),.UNSPECIFIED.,.F.,.F.)
B_SPLINE_CURVE_WITH_KNOTS((3,3),(0.0420809670913706,0.0588848364681992),
 .UNSPECIFIED.)
CURVE()
GEOMETRIC_REPRESENTATION_ITEM()
RATIONAL_B_SPLINE_CURVE((1.00087707567803,1.00061365578598,1.))
REPRESENTATION_ITEM('')
);
#321=(
BOUNDED_CURVE()
B_SPLINE_CURVE(2,(#36071,#36072,#36073),.UNSPECIFIED.,.F.,.F.)
B_SPLINE_CURVE_WITH_KNOTS((3,3),(0.,0.0168038693768352),.UNSPECIFIED.)
CURVE()
GEOMETRIC_REPRESENTATION_ITEM()
RATIONAL_B_SPLINE_CURVE((1.,1.00061365578544,1.00087707567725))
REPRESENTATION_ITEM('')
);
#322=(
BOUNDED_CURVE()
B_SPLINE_CURVE(2,(#36078,#36079,#36080),.UNSPECIFIED.,.F.,.F.)
B_SPLINE_CURVE_WITH_KNOTS((3,3),(0.0420809670913822,0.0588848364681993),
 .UNSPECIFIED.)
CURVE()
GEOMETRIC_REPRESENTATION_ITEM()
RATIONAL_B_SPLINE_CURVE((1.00087707567791,1.00061365578591,1.))
REPRESENTATION_ITEM('')
);
#323=(
BOUNDED_CURVE()
B_SPLINE_CURVE(2,(#36085,#36086,#36087),.UNSPECIFIED.,.F.,.F.)
B_SPLINE_CURVE_WITH_KNOTS((3,3),(0.,0.0168038693768391),.UNSPECIFIED.)
CURVE()
GEOMETRIC_REPRESENTATION_ITEM()
RATIONAL_B_SPLINE_CURVE((1.,1.00061365578625,1.0008770756784))
REPRESENTATION_ITEM('')
);
#324=(
BOUNDED_CURVE()
B_SPLINE_CURVE(2,(#36092,#36093,#36094),.UNSPECIFIED.,.F.,.F.)
B_SPLINE_CURVE_WITH_KNOTS((3,3),(0.0420809670913788,0.0588848364681992),
 .UNSPECIFIED.)
CURVE()
GEOMETRIC_REPRESENTATION_ITEM()
RATIONAL_B_SPLINE_CURVE((1.00087707567811,1.00061365578604,1.))
REPRESENTATION_ITEM('')
);
#325=(
BOUNDED_CURVE()
B_SPLINE_CURVE(2,(#36099,#36100,#36101),.UNSPECIFIED.,.F.,.F.)
B_SPLINE_CURVE_WITH_KNOTS((3,3),(0.,0.0168038693768716),.UNSPECIFIED.)
CURVE()
GEOMETRIC_REPRESENTATION_ITEM()
RATIONAL_B_SPLINE_CURVE((1.,1.00061365578607,1.00087707567815))
REPRESENTATION_ITEM('')
);
#326=(
BOUNDED_CURVE()
B_SPLINE_CURVE(2,(#36106,#36107,#36108),.UNSPECIFIED.,.F.,.F.)
B_SPLINE_CURVE_WITH_KNOTS((3,3),(0.0420809670913493,0.0588848364681993),
 .UNSPECIFIED.)
CURVE()
GEOMETRIC_REPRESENTATION_ITEM()
RATIONAL_B_SPLINE_CURVE((1.00087707567838,1.00061365578623,1.))
REPRESENTATION_ITEM('')
);
#327=(
BOUNDED_CURVE()
B_SPLINE_CURVE(2,(#36113,#36114,#36115),.UNSPECIFIED.,.F.,.F.)
B_SPLINE_CURVE_WITH_KNOTS((3,3),(0.,0.0168038693768289),.UNSPECIFIED.)
CURVE()
GEOMETRIC_REPRESENTATION_ITEM()
RATIONAL_B_SPLINE_CURVE((1.,1.00061365578616,1.00087707567828))
REPRESENTATION_ITEM('')
);
#328=(
BOUNDED_CURVE()
B_SPLINE_CURVE(2,(#36120,#36121,#36122),.UNSPECIFIED.,.F.,.F.)
B_SPLINE_CURVE_WITH_KNOTS((3,3),(0.0420809670913749,0.0588848364681992),
 .UNSPECIFIED.)
CURVE()
GEOMETRIC_REPRESENTATION_ITEM()
RATIONAL_B_SPLINE_CURVE((1.00087707567811,1.00061365578604,1.))
REPRESENTATION_ITEM('')
);
#329=(
BOUNDED_CURVE()
B_SPLINE_CURVE(2,(#36127,#36128,#36129),.UNSPECIFIED.,.F.,.F.)
B_SPLINE_CURVE_WITH_KNOTS((3,3),(0.,0.0168038693768264),.UNSPECIFIED.)
CURVE()
GEOMETRIC_REPRESENTATION_ITEM()
RATIONAL_B_SPLINE_CURVE((1.,1.00061365578613,1.00087707567823))
REPRESENTATION_ITEM('')
);
#330=(
BOUNDED_CURVE()
B_SPLINE_CURVE(2,(#36134,#36135,#36136),.UNSPECIFIED.,.F.,.F.)
B_SPLINE_CURVE_WITH_KNOTS((3,3),(0.0420809670913744,0.0588848364681992),
 .UNSPECIFIED.)
CURVE()
GEOMETRIC_REPRESENTATION_ITEM()
RATIONAL_B_SPLINE_CURVE((1.00087707567875,1.00061365578649,1.))
REPRESENTATION_ITEM('')
);
#331=(
BOUNDED_CURVE()
B_SPLINE_CURVE(2,(#36141,#36142,#36143),.UNSPECIFIED.,.F.,.F.)
B_SPLINE_CURVE_WITH_KNOTS((3,3),(0.,0.0168038693768507),.UNSPECIFIED.)
CURVE()
GEOMETRIC_REPRESENTATION_ITEM()
RATIONAL_B_SPLINE_CURVE((1.,1.00061365578591,1.00087707567792))
REPRESENTATION_ITEM('')
);
#332=(
BOUNDED_CURVE()
B_SPLINE_CURVE(2,(#36148,#36149,#36150),.UNSPECIFIED.,.F.,.F.)
B_SPLINE_CURVE_WITH_KNOTS((3,3),(0.0420809670913786,0.0588848364681993),
 .UNSPECIFIED.)
CURVE()
GEOMETRIC_REPRESENTATION_ITEM()
RATIONAL_B_SPLINE_CURVE((1.00087707567801,1.00061365578597,1.))
REPRESENTATION_ITEM('')
);
#333=(
BOUNDED_CURVE()
B_SPLINE_CURVE(2,(#36155,#36156,#36157),.UNSPECIFIED.,.F.,.F.)
B_SPLINE_CURVE_WITH_KNOTS((3,3),(0.,0.0168038693768258),.UNSPECIFIED.)
CURVE()
GEOMETRIC_REPRESENTATION_ITEM()
RATIONAL_B_SPLINE_CURVE((1.,1.00061365578592,1.00087707567793))
REPRESENTATION_ITEM('')
);
#334=(
BOUNDED_CURVE()
B_SPLINE_CURVE(2,(#36162,#36163,#36164),.UNSPECIFIED.,.F.,.F.)
B_SPLINE_CURVE_WITH_KNOTS((3,3),(0.0420809670913652,0.0588848364681993),
 .UNSPECIFIED.)
CURVE()
GEOMETRIC_REPRESENTATION_ITEM()
RATIONAL_B_SPLINE_CURVE((1.00087707567844,1.00061365578627,1.))
REPRESENTATION_ITEM('')
);
#335=(
BOUNDED_CURVE()
B_SPLINE_CURVE(2,(#36169,#36170,#36171),.UNSPECIFIED.,.F.,.F.)
B_SPLINE_CURVE_WITH_KNOTS((3,3),(0.,0.0168038693768152),.UNSPECIFIED.)
CURVE()
GEOMETRIC_REPRESENTATION_ITEM()
RATIONAL_B_SPLINE_CURVE((1.,1.00061365578615,1.00087707567826))
REPRESENTATION_ITEM('')
);
#444=SHAPE_REPRESENTATION_RELATIONSHIP('SRR','None',#38680,#458);
#458=ADVANCED_BREP_SHAPE_REPRESENTATION('',(#486),#38609);
#472=STYLED_ITEM('',(#38885),#486);
#486=MANIFOLD_SOLID_BREP('Screw',#16246);
#489=TOROIDAL_SURFACE('',#17387,0.2154,0.02);
#506=B_SPLINE_SURFACE_WITH_KNOTS('',3,3,((#33981,#33982,#33983,#33984,#33985,
#33986,#33987,#33988,#33989,#33990,#33991,#33992,#33993,#33994,#33995,#33996,
#33997,#33998,#33999,#34000,#34001,#34002,#34003,#34004,#34005,#34006,#34007,
#34008,#34009,#34010,#34011,#34012,#34013,#34014,#34015,#34016,#34017,#34018,
#34019,#34020,#34021,#34022,#34023,#34024,#34025,#34026,#34027,#34028,#34029,
#34030,#34031,#34032,#34033,#34034,#34035,#34036,#34037,#34038,#34039,#34040,
#34041,#34042,#34043,#34044,#34045,#34046,#34047,#34048,#34049,#34050,#34051,
#34052,#34053,#34054,#34055,#34056,#34057,#34058,#34059,#34060,#34061,#34062,
#34063,#34064,#34065,#34066,#34067,#34068,#34069,#34070,#34071,#34072,#34073,
#34074,#34075,#34076,#34077,#34078,#34079,#34080,#34081,#34082,#34083,#34084,
#34085,#34086,#34087,#34088,#34089,#34090,#34091,#34092,#34093,#34094,#34095,
#34096,#34097,#34098,#34099,#34100,#34101,#34102,#34103,#34104,#34105,#34106,
#34107,#34108,#34109,#34110,#34111,#34112,#34113,#34114,#34115,#34116,#34117,
#34118,#34119,#34120,#34121,#34122,#34123,#34124),(#34125,#34126,#34127,
#34128,#34129,#34130,#34131,#34132,#34133,#34134,#34135,#34136,#34137,#34138,
#34139,#34140,#34141,#34142,#34143,#34144,#34145,#34146,#34147,#34148,#34149,
#34150,#34151,#34152,#34153,#34154,#34155,#34156,#34157,#34158,#34159,#34160,
#34161,#34162,#34163,#34164,#34165,#34166,#34167,#34168,#34169,#34170,#34171,
#34172,#34173,#34174,#34175,#34176,#34177,#34178,#34179,#34180,#34181,#34182,
#34183,#34184,#34185,#34186,#34187,#34188,#34189,#34190,#34191,#34192,#34193,
#34194,#34195,#34196,#34197,#34198,#34199,#34200,#34201,#34202,#34203,#34204,
#34205,#34206,#34207,#34208,#34209,#34210,#34211,#34212,#34213,#34214,#34215,
#34216,#34217,#34218,#34219,#34220,#34221,#34222,#34223,#34224,#34225,#34226,
#34227,#34228,#34229,#34230,#34231,#34232,#34233,#34234,#34235,#34236,#34237,
#34238,#34239,#34240,#34241,#34242,#34243,#34244,#34245,#34246,#34247,#34248,
#34249,#34250,#34251,#34252,#34253,#34254,#34255,#34256,#34257,#34258,#34259,
#34260,#34261,#34262,#34263,#34264,#34265,#34266,#34267,#34268),(#34269,
#34270,#34271,#34272,#34273,#34274,#34275,#34276,#34277,#34278,#34279,#34280,
#34281,#34282,#34283,#34284,#34285,#34286,#34287,#34288,#34289,#34290,#34291,
#34292,#34293,#34294,#34295,#34296,#34297,#34298,#34299,#34300,#34301,#34302,
#34303,#34304,#34305,#34306,#34307,#34308,#34309,#34310,#34311,#34312,#34313,
#34314,#34315,#34316,#34317,#34318,#34319,#34320,#34321,#34322,#34323,#34324,
#34325,#34326,#34327,#34328,#34329,#34330,#34331,#34332,#34333,#34334,#34335,
#34336,#34337,#34338,#34339,#34340,#34341,#34342,#34343,#34344,#34345,#34346,
#34347,#34348,#34349,#34350,#34351,#34352,#34353,#34354,#34355,#34356,#34357,
#34358,#34359,#34360,#34361,#34362,#34363,#34364,#34365,#34366,#34367,#34368,
#34369,#34370,#34371,#34372,#34373,#34374,#34375,#34376,#34377,#34378,#34379,
#34380,#34381,#34382,#34383,#34384,#34385,#34386,#34387,#34388,#34389,#34390,
#34391,#34392,#34393,#34394,#34395,#34396,#34397,#34398,#34399,#34400,#34401,
#34402,#34403,#34404,#34405,#34406,#34407,#34408,#34409,#34410,#34411,#34412),
(#34413,#34414,#34415,#34416,#34417,#34418,#34419,#34420,#34421,#34422,
#34423,#34424,#34425,#34426,#34427,#34428,#34429,#34430,#34431,#34432,#34433,
#34434,#34435,#34436,#34437,#34438,#34439,#34440,#34441,#34442,#34443,#34444,
#34445,#34446,#34447,#34448,#34449,#34450,#34451,#34452,#34453,#34454,#34455,
#34456,#34457,#34458,#34459,#34460,#34461,#34462,#34463,#34464,#34465,#34466,
#34467,#34468,#34469,#34470,#34471,#34472,#34473,#34474,#34475,#34476,#34477,
#34478,#34479,#34480,#34481,#34482,#34483,#34484,#34485,#34486,#34487,#34488,
#34489,#34490,#34491,#34492,#34493,#34494,#34495,#34496,#34497,#34498,#34499,
#34500,#34501,#34502,#34503,#34504,#34505,#34506,#34507,#34508,#34509,#34510,
#34511,#34512,#34513,#34514,#34515,#34516,#34517,#34518,#34519,#34520,#34521,
#34522,#34523,#34524,#34525,#34526,#34527,#34528,#34529,#34530,#34531,#34532,
#34533,#34534,#34535,#34536,#34537,#34538,#34539,#34540,#34541,#34542,#34543,
#34544,#34545,#34546,#34547,#34548,#34549,#34550,#34551,#34552,#34553,#34554,
#34555,#34556)),.UNSPECIFIED.,.F.,.F.,.F.,(4,4),(4,1,1,1,1,1,1,1,1,1,1,
1,1,1,1,1,1,1,1,1,1,1,1,1,1,1,1,1,1,1,1,1,1,1,1,1,1,1,1,1,1,1,1,1,1,1,1,
1,1,1,1,1,1,1,1,1,1,1,1,1,1,1,1,1,1,1,1,1,1,1,1,1,1,1,1,1,1,1,1,1,1,1,1,
1,1,1,1,1,1,1,1,1,1,1,1,1,1,1,1,1,1,1,1,1,1,1,1,1,1,1,1,1,1,1,1,1,1,1,1,
1,1,1,1,1,1,1,1,1,1,1,1,1,1,1,1,1,1,1,1,1,1,4),(0.,0.0460148164544131),
(8.31058692273977,9.30851679455325,10.3064466663667,11.3043765381802,12.3023064099937,
13.3002362818072,14.2981661536207,15.2960960254341,16.2940258972476,17.2919557690611,
18.2898856408746,19.2878155126881,20.2857453845015,21.283675256315,22.2816051281285,
23.279534999942,24.2774648717555,25.2753947435689,26.2733246153824,27.2712544871959,
28.2691843590094,29.2671142308229,30.2650441026364,31.2629739744498,32.2609038462633,
33.2588337180768,34.2567635898903,35.2546934617038,36.2526233335172,37.2505532053307,
38.2484830771442,39.2464129489577,40.2443428207712,41.2422726925846,42.2402025643981,
43.2381324362116,44.2360623080251,45.2339921798386,46.231922051652,47.2298519234655,
48.227781795279,49.2257116670925,50.223641538906,51.2215714107194,52.2195012825329,
53.2174311543464,54.2153610261599,55.2132908979734,56.2112207697869,57.2091506416003,
58.2070805134138,59.2050103852273,60.2029402570408,61.2008701288543,62.1988000006677,
63.1967298724812,64.1946597442947,65.1925896161082,66.1905194879217,67.1884493597351,
68.1863792315486,69.1843091033621,70.1822389751756,71.1801688469891,72.1780987188026,
73.176028590616,74.1739584624295,75.171888334243,76.1698182060565,77.16774807787,
78.1656779496834,79.1636078214969,80.1615376933104,81.1594675651239,82.1573974369374,
83.1553273087509,84.1532571805643,85.1511870523778,86.1491169241913,87.1470467960048,
88.1449766678183,89.1429065396317,90.1408364114452,91.1387662832587,92.1366961550722,
93.1346260268857,94.1325558986991,95.1304857705126,96.1284156423261,97.1263455141396,
98.1242753859531,99.1222052577666,100.12013512958,101.118065001394,102.115994873207,
103.11392474502,104.111854616834,105.109784488647,106.107714360461,107.105644232274,
108.103574104088,109.101503975901,110.099433847715,111.097363719528,112.095293591342,
113.093223463155,114.091153334969,115.089083206782,116.087013078596,117.084942950409,
118.082872822223,119.080802694036,120.07873256585,121.076662437663,122.074592309477,
123.07252218129,124.070452053104,125.068381924917,126.066311796731,127.064241668544,
128.062171540357,129.060101412171,130.058031283984,131.055961155798,132.053891027611,
133.051820899425,134.049750771238,135.047680643052,136.045610514865,137.043540386679,
138.041470258492,139.039400130306,140.037330002119,141.035259873933,142.033189745746,
143.03111961756,144.029049489373,145.026979361187,146.024909233,147.022839104814,
148.020768976627,149.018698848441),.UNSPECIFIED.);
#507=B_SPLINE_SURFACE_WITH_KNOTS('',3,3,((#34705,#34706,#34707,#34708,#34709,
#34710,#34711,#34712,#34713,#34714,#34715,#34716,#34717,#34718,#34719,#34720,
#34721,#34722,#34723,#34724,#34725,#34726,#34727,#34728,#34729,#34730,#34731,
#34732,#34733,#34734,#34735,#34736,#34737,#34738,#34739,#34740,#34741,#34742,
#34743,#34744,#34745,#34746,#34747,#34748,#34749,#34750,#34751,#34752,#34753,
#34754,#34755,#34756,#34757,#34758,#34759,#34760,#34761,#34762,#34763,#34764,
#34765,#34766,#34767,#34768,#34769,#34770,#34771,#34772,#34773,#34774,#34775,
#34776,#34777,#34778,#34779,#34780,#34781,#34782,#34783,#34784,#34785,#34786,
#34787,#34788,#34789,#34790,#34791,#34792,#34793,#34794,#34795,#34796,#34797,
#34798,#34799,#34800,#34801,#34802,#34803,#34804,#34805,#34806,#34807,#34808,
#34809,#34810,#34811,#34812,#34813,#34814,#34815,#34816,#34817,#34818,#34819,
#34820,#34821,#34822,#34823,#34824,#34825,#34826,#34827,#34828,#34829,#34830,
#34831,#34832,#34833,#34834,#34835,#34836,#34837,#34838,#34839,#34840,#34841,
#34842,#34843,#34844,#34845,#34846,#34847,#34848),(#34849,#34850,#34851,
#34852,#34853,#34854,#34855,#34856,#34857,#34858,#34859,#34860,#34861,#34862,
#34863,#34864,#34865,#34866,#34867,#34868,#34869,#34870,#34871,#34872,#34873,
#34874,#34875,#34876,#34877,#34878,#34879,#34880,#34881,#34882,#34883,#34884,
#34885,#34886,#34887,#34888,#34889,#34890,#34891,#34892,#34893,#34894,#34895,
#34896,#34897,#34898,#34899,#34900,#34901,#34902,#34903,#34904,#34905,#34906,
#34907,#34908,#34909,#34910,#34911,#34912,#34913,#34914,#34915,#34916,#34917,
#34918,#34919,#34920,#34921,#34922,#34923,#34924,#34925,#34926,#34927,#34928,
#34929,#34930,#34931,#34932,#34933,#34934,#34935,#34936,#34937,#34938,#34939,
#34940,#34941,#34942,#34943,#34944,#34945,#34946,#34947,#34948,#34949,#34950,
#34951,#34952,#34953,#34954,#34955,#34956,#34957,#34958,#34959,#34960,#34961,
#34962,#34963,#34964,#34965,#34966,#34967,#34968,#34969,#34970,#34971,#34972,
#34973,#34974,#34975,#34976,#34977,#34978,#34979,#34980,#34981,#34982,#34983,
#34984,#34985,#34986,#34987,#34988,#34989,#34990,#34991,#34992),(#34993,
#34994,#34995,#34996,#34997,#34998,#34999,#35000,#35001,#35002,#35003,#35004,
#35005,#35006,#35007,#35008,#35009,#35010,#35011,#35012,#35013,#35014,#35015,
#35016,#35017,#35018,#35019,#35020,#35021,#35022,#35023,#35024,#35025,#35026,
#35027,#35028,#35029,#35030,#35031,#35032,#35033,#35034,#35035,#35036,#35037,
#35038,#35039,#35040,#35041,#35042,#35043,#35044,#35045,#35046,#35047,#35048,
#35049,#35050,#35051,#35052,#35053,#35054,#35055,#35056,#35057,#35058,#35059,
#35060,#35061,#35062,#35063,#35064,#35065,#35066,#35067,#35068,#35069,#35070,
#35071,#35072,#35073,#35074,#35075,#35076,#35077,#35078,#35079,#35080,#35081,
#35082,#35083,#35084,#35085,#35086,#35087,#35088,#35089,#35090,#35091,#35092,
#35093,#35094,#35095,#35096,#35097,#35098,#35099,#35100,#35101,#35102,#35103,
#35104,#35105,#35106,#35107,#35108,#35109,#35110,#35111,#35112,#35113,#35114,
#35115,#35116,#35117,#35118,#35119,#35120,#35121,#35122,#35123,#35124,#35125,
#35126,#35127,#35128,#35129,#35130,#35131,#35132,#35133,#35134,#35135,#35136),
(#35137,#35138,#35139,#35140,#35141,#35142,#35143,#35144,#35145,#35146,
#35147,#35148,#35149,#35150,#35151,#35152,#35153,#35154,#35155,#35156,#35157,
#35158,#35159,#35160,#35161,#35162,#35163,#35164,#35165,#35166,#35167,#35168,
#35169,#35170,#35171,#35172,#35173,#35174,#35175,#35176,#35177,#35178,#35179,
#35180,#35181,#35182,#35183,#35184,#35185,#35186,#35187,#35188,#35189,#35190,
#35191,#35192,#35193,#35194,#35195,#35196,#35197,#35198,#35199,#35200,#35201,
#35202,#35203,#35204,#35205,#35206,#35207,#35208,#35209,#35210,#35211,#35212,
#35213,#35214,#35215,#35216,#35217,#35218,#35219,#35220,#35221,#35222,#35223,
#35224,#35225,#35226,#35227,#35228,#35229,#35230,#35231,#35232,#35233,#35234,
#35235,#35236,#35237,#35238,#35239,#35240,#35241,#35242,#35243,#35244,#35245,
#35246,#35247,#35248,#35249,#35250,#35251,#35252,#35253,#35254,#35255,#35256,
#35257,#35258,#35259,#35260,#35261,#35262,#35263,#35264,#35265,#35266,#35267,
#35268,#35269,#35270,#35271,#35272,#35273,#35274,#35275,#35276,#35277,#35278,
#35279,#35280)),.UNSPECIFIED.,.F.,.F.,.F.,(4,4),(4,1,1,1,1,1,1,1,1,1,1,
1,1,1,1,1,1,1,1,1,1,1,1,1,1,1,1,1,1,1,1,1,1,1,1,1,1,1,1,1,1,1,1,1,1,1,1,
1,1,1,1,1,1,1,1,1,1,1,1,1,1,1,1,1,1,1,1,1,1,1,1,1,1,1,1,1,1,1,1,1,1,1,1,
1,1,1,1,1,1,1,1,1,1,1,1,1,1,1,1,1,1,1,1,1,1,1,1,1,1,1,1,1,1,1,1,1,1,1,1,
1,1,1,1,1,1,1,1,1,1,1,1,1,1,1,1,1,1,1,1,1,1,4),(0.,0.0460148164544131),
(11.6154215191106,12.6133513909241,13.6112812627376,14.6092111345511,15.6071410063646,
16.605070878178,17.6030007499915,18.600930621805,19.5988604936185,20.596790365432,
21.5947202372454,22.5926501090589,23.5905799808724,24.5885098526859,25.5864397244994,
26.5843695963128,27.5822994681263,28.5802293399398,29.5781592117533,30.5760890835668,
31.5740189553803,32.5719488271937,33.5698786990072,34.5678085708207,35.5657384426342,
36.5636683144477,37.5615981862611,38.5595280580746,39.5574579298881,40.5553878017016,
41.5533176735151,42.5512475453285,43.549177417142,44.5471072889555,45.545037160769,
46.5429670325825,47.540896904396,48.5388267762094,49.5367566480229,50.5346865198364,
51.5326163916499,52.5305462634634,53.5284761352768,54.5264060070903,55.5243358789038,
56.5222657507173,57.5201956225308,58.5181254943442,59.5160553661577,60.5139852379712,
61.5119151097847,62.5098449815982,63.5077748534116,64.5057047252251,65.5036345970386,
66.5015644688521,67.4994943406656,68.497424212479,69.4953540842925,70.493283956106,
71.4912138279195,72.489143699733,73.4870735715464,74.4850034433599,75.4829333151734,
76.4808631869869,77.4787930588004,78.4767229306139,79.4746528024273,80.4725826742408,
81.4705125460543,82.4684424178678,83.4663722896813,84.4643021614947,85.4622320333082,
86.4601619051217,87.4580917769352,88.4560216487487,89.4539515205621,90.4518813923756,
91.4498112641891,92.4477411360026,93.4456710078161,94.4436008796296,95.441530751443,
96.4394606232565,97.43739049507,98.4353203668835,99.433250238697,100.43118011051,
101.429109982324,102.427039854137,103.424969725951,104.422899597764,105.420829469578,
106.418759341391,107.416689213205,108.414619085018,109.412548956832,110.410478828645,
111.408408700459,112.406338572272,113.404268444086,114.402198315899,115.400128187713,
116.398058059526,117.39598793134,118.393917803153,119.391847674967,120.38977754678,
121.387707418594,122.385637290407,123.383567162221,124.381497034034,125.379426905847,
126.377356777661,127.375286649474,128.373216521288,129.371146393101,130.369076264915,
131.367006136728,132.364936008542,133.362865880355,134.360795752169,135.358725623982,
136.356655495796,137.354585367609,138.352515239423,139.350445111236,140.34837498305,
141.346304854863,142.344234726677,143.34216459849,144.340094470304,145.338024342117,
146.335954213931,147.333884085744,148.331813957558,149.329743829371,150.327673701184,
151.325603572998,152.323533444811),.UNSPECIFIED.);
#729=B_SPLINE_CURVE_WITH_KNOTS('',3,(#32274,#32275,#32276,#32277,#32278,
#32279,#32280,#32281,#32282,#32283),.UNSPECIFIED.,.F.,.F.,(4,3,3,4),(-4.09254174883829,
-3.99171948725392,-2.99378961544044,-2.06514013327807),.UNSPECIFIED.);
#730=B_SPLINE_CURVE_WITH_KNOTS('',3,(#32286,#32287,#32288,#32289,#32290,
#32291,#32292),.UNSPECIFIED.,.F.,.F.,(4,3,4),(0.,0.997929871813473,1.11419103802947),
 .UNSPECIFIED.);
#731=B_SPLINE_CURVE_WITH_KNOTS('',3,(#32297,#32298,#32299,#32300,#32301,
#32302,#32303,#32304,#32305,#32306,#32307,#32308,#32309,#32310,#32311,#32312,
#32313,#32314,#32315,#32316,#32317,#32318),.UNSPECIFIED.,.F.,.F.,(4,3,3,
3,3,3,3,4),(-10.3757270560179,-9.97929871813481,-8.98136884632133,-7.98343897450785,
-6.98550910269437,-5.98757923088089,-4.98964935906741,-4.09254174883829),
 .UNSPECIFIED.);
#732=B_SPLINE_CURVE_WITH_KNOTS('',3,(#32319,#32320,#32321,#32322,#32323,
#32324,#32325,#32326,#32327,#32328,#32329,#32330,#32331,#32332,#32333,#32334,
#32335,#32336,#32337,#32338,#32339,#32340),.UNSPECIFIED.,.F.,.F.,(4,3,3,
3,3,3,3,4),(1.11419103802947,1.99585974362696,2.99378961544044,3.99171948725392,
4.9896493590674,5.98757923088088,6.98550910269437,7.39737634520906),
 .UNSPECIFIED.);
#733=B_SPLINE_CURVE_WITH_KNOTS('',3,(#32345,#32346,#32347,#32348,#32349,
#32350,#32351,#32352,#32353,#32354,#32355,#32356,#32357,#32358,#32359,#32360,
#32361,#32362,#32363,#32364,#32365,#32366),.UNSPECIFIED.,.F.,.F.,(4,3,3,
3,3,3,3,4),(-16.6589123631975,-15.9668779490157,-14.9689480772022,-13.9710182053887,
-12.9730883335753,-11.9751584617618,-10.9772285899483,-10.3757270560179),
 .UNSPECIFIED.);
#734=B_SPLINE_CURVE_WITH_KNOTS('',3,(#32367,#32368,#32369,#32370,#32371,
#32372,#32373,#32374,#32375,#32376,#32377,#32378,#32379,#32380,#32381,#32382,
#32383,#32384,#32385,#32386,#32387,#32388),.UNSPECIFIED.,.F.,.F.,(4,3,3,
3,3,3,3,4),(7.39737634520906,7.98343897450785,8.98136884632133,9.97929871813481,
10.9772285899483,11.9751584617618,12.9730883335753,13.6805616523886),
 .UNSPECIFIED.);
#735=B_SPLINE_CURVE_WITH_KNOTS('',3,(#32393,#32394,#32395,#32396,#32397,
#32398,#32399,#32400,#32401,#32402,#32403,#32404,#32405,#32406,#32407,#32408,
#32409,#32410,#32411,#32412,#32413,#32414),.UNSPECIFIED.,.F.,.F.,(4,3,3,
3,3,3,3,4),(-22.942097670377,-21.9544571798966,-20.9565273080831,-19.9585974362696,
-18.9606675644561,-17.9627376926427,-16.9648078208292,-16.6589123631975),
 .UNSPECIFIED.);
#736=B_SPLINE_CURVE_WITH_KNOTS('',3,(#32415,#32416,#32417,#32418,#32419,
#32420,#32421,#32422,#32423,#32424,#32425,#32426,#32427,#32428,#32429,#32430,
#32431,#32432,#32433,#32434,#32435,#32436,#32437,#32438,#32439),
 .UNSPECIFIED.,.F.,.F.,(4,3,3,3,3,3,3,3,4),(13.6805616523886,13.9710182053887,
14.9689480772022,15.9668779490157,16.9648078208292,17.9627376926427,18.9606675644561,
19.9585974362696,19.9637469595682),.UNSPECIFIED.);
#737=B_SPLINE_CURVE_WITH_KNOTS('',3,(#32444,#32445,#32446,#32447,#32448,
#32449,#32450,#32451,#32452,#32453,#32454,#32455,#32456,#32457,#32458,#32459,
#32460,#32461,#32462,#32463,#32464,#32465,#32466,#32467,#32468),
 .UNSPECIFIED.,.F.,.F.,(4,3,3,3,3,3,3,3,4),(-29.2252829775566,-28.9399662825909,
-27.9420364107775,-26.944106538964,-25.9461766671505,-24.948246795337,-23.9503169235235,
-22.9523870517101,-22.942097670377),.UNSPECIFIED.);
#738=B_SPLINE_CURVE_WITH_KNOTS('',3,(#32469,#32470,#32471,#32472,#32473,
#32474,#32475,#32476,#32477,#32478,#32479,#32480,#32481,#32482,#32483,#32484,
#32485,#32486,#32487,#32488,#32489,#32490),.UNSPECIFIED.,.F.,.F.,(4,3,3,
3,3,3,3,4),(19.9637469595682,20.9565273080831,21.9544571798966,22.9523870517101,
23.9503169235235,24.948246795337,25.9461766671505,26.2469322667478),
 .UNSPECIFIED.);
#739=B_SPLINE_CURVE_WITH_KNOTS('',3,(#32495,#32496,#32497,#32498,#32499,
#32500,#32501,#32502,#32503,#32504,#32505,#32506,#32507,#32508,#32509,#32510,
#32511,#32512,#32513,#32514,#32515,#32516),.UNSPECIFIED.,.F.,.F.,(4,3,3,
3,3,3,3,4),(-35.5084682847362,-34.9275455134718,-33.9296156416584,-32.9316857698449,
-31.9337558980314,-30.9358260262179,-29.9378961544044,-29.2252829775566),
 .UNSPECIFIED.);
#740=B_SPLINE_CURVE_WITH_KNOTS('',3,(#32517,#32518,#32519,#32520,#32521,
#32522,#32523,#32524,#32525,#32526,#32527,#32528,#32529,#32530,#32531,#32532,
#32533,#32534,#32535,#32536,#32537,#32538),.UNSPECIFIED.,.F.,.F.,(4,3,3,
3,3,3,3,4),(26.2469322667478,26.944106538964,27.9420364107775,28.9399662825909,
29.9378961544044,30.9358260262179,31.9337558980314,32.5301175739274),
 .UNSPECIFIED.);
#741=B_SPLINE_CURVE_WITH_KNOTS('',3,(#32543,#32544,#32545,#32546,#32547,
#32548,#32549,#32550,#32551,#32552,#32553,#32554,#32555,#32556,#32557,#32558,
#32559,#32560,#32561,#32562,#32563,#32564),.UNSPECIFIED.,.F.,.F.,(4,3,3,
3,3,3,3,4),(-41.7916535919158,-40.9151247443527,-39.9171948725392,-38.9192650007258,
-37.9213351289123,-36.9234052570988,-35.9254753852853,-35.5084682847362),
 .UNSPECIFIED.);
#742=B_SPLINE_CURVE_WITH_KNOTS('',3,(#32565,#32566,#32567,#32568,#32569,
#32570,#32571,#32572,#32573,#32574,#32575,#32576,#32577,#32578,#32579,#32580,
#32581,#32582,#32583,#32584,#32585,#32586),.UNSPECIFIED.,.F.,.F.,(4,3,3,
3,3,3,3,4),(32.5301175739274,32.9316857698449,33.9296156416584,34.9275455134718,
35.9254753852853,36.9234052570988,37.9213351289123,38.813302881107),
 .UNSPECIFIED.);
#743=B_SPLINE_CURVE_WITH_KNOTS('',3,(#32591,#32592,#32593,#32594,#32595,
#32596,#32597,#32598,#32599,#32600,#32601,#32602,#32603,#32604,#32605,#32606,
#32607,#32608,#32609,#32610,#32611,#32612,#32613,#32614,#32615),
 .UNSPECIFIED.,.F.,.F.,(4,3,3,3,3,3,3,3,4),(-48.0748388990954,-47.9006338470471,
-46.9027039752336,-45.9047741034201,-44.9068442316067,-43.9089143597932,
-42.9109844879797,-41.9130546161662,-41.7916535919158),.UNSPECIFIED.);
#744=B_SPLINE_CURVE_WITH_KNOTS('',3,(#32616,#32617,#32618,#32619,#32620,
#32621,#32622,#32623,#32624,#32625,#32626,#32627,#32628,#32629,#32630,#32631,
#32632,#32633,#32634,#32635,#32636,#32637,#32638,#32639,#32640),
 .UNSPECIFIED.,.F.,.F.,(4,3,3,3,3,3,3,3,4),(38.813302881107,38.9192650007258,
39.9171948725392,40.9151247443527,41.9130546161662,42.9109844879797,43.9089143597932,
44.9068442316066,45.0964881882866),.UNSPECIFIED.);
#745=B_SPLINE_CURVE_WITH_KNOTS('',3,(#32645,#32646,#32647,#32648,#32649,
#32650,#32651,#32652,#32653,#32654,#32655,#32656,#32657,#32658,#32659,#32660,
#32661,#32662,#32663,#32664,#32665,#32666),.UNSPECIFIED.,.F.,.F.,(4,3,3,
3,3,3,3,4),(-54.358024206275,-53.888213077928,-52.8902832061145,-51.892353334301,
-50.8944234624875,-49.8964935906741,-48.8985637188606,-48.0748388990954),
 .UNSPECIFIED.);
#746=B_SPLINE_CURVE_WITH_KNOTS('',3,(#32667,#32668,#32669,#32670,#32671,
#32672,#32673,#32674,#32675,#32676,#32677,#32678,#32679,#32680,#32681,#32682,
#32683,#32684,#32685,#32686,#32687,#32688),.UNSPECIFIED.,.F.,.F.,(4,3,3,
3,3,3,3,4),(45.0964881882866,45.9047741034201,46.9027039752336,47.9006338470471,
48.8985637188606,49.8964935906741,50.8944234624875,51.3796734954662),
 .UNSPECIFIED.);
#747=B_SPLINE_CURVE_WITH_KNOTS('',3,(#32693,#32694,#32695,#32696,#32697,
#32698,#32699,#32700,#32701,#32702,#32703,#32704,#32705,#32706,#32707,#32708,
#32709,#32710,#32711,#32712,#32713,#32714),.UNSPECIFIED.,.F.,.F.,(4,3,3,
3,3,3,3,4),(-60.6412095134546,-59.8757923088089,-58.8778624369954,-57.8799325651819,
-56.8820026933684,-55.8840728215549,-54.8861429497415,-54.358024206275),
 .UNSPECIFIED.);
#748=B_SPLINE_CURVE_WITH_KNOTS('',3,(#32715,#32716,#32717,#32718,#32719,
#32720,#32721,#32722,#32723,#32724,#32725,#32726,#32727,#32728,#32729,#32730,
#32731,#32732,#32733,#32734,#32735,#32736),.UNSPECIFIED.,.F.,.F.,(4,3,3,
3,3,3,3,4),(51.3796734954662,51.892353334301,52.8902832061145,53.888213077928,
54.8861429497415,55.8840728215549,56.8820026933684,57.6628588026458),
 .UNSPECIFIED.);
#749=B_SPLINE_CURVE_WITH_KNOTS('',3,(#32741,#32742,#32743,#32744,#32745,
#32746,#32747,#32748,#32749,#32750,#32751,#32752,#32753,#32754,#32755,#32756,
#32757,#32758,#32759,#32760,#32761,#32762,#32763,#32764,#32765),
 .UNSPECIFIED.,.F.,.F.,(4,3,3,3,3,3,3,3,4),(-66.9243948206342,-66.8613014115032,
-65.8633715396898,-64.8654416678763,-63.8675117960628,-62.8695819242493,
-61.8716520524358,-60.8737221806224,-60.6412095134546),.UNSPECIFIED.);
#750=B_SPLINE_CURVE_WITH_KNOTS('',3,(#32766,#32767,#32768,#32769,#32770,
#32771,#32772,#32773,#32774,#32775,#32776,#32777,#32778,#32779,#32780,#32781,
#32782,#32783,#32784,#32785,#32786,#32787,#32788,#32789,#32790),
 .UNSPECIFIED.,.F.,.F.,(4,3,3,3,3,3,3,3,4),(57.6628588026458,57.8799325651819,
58.8778624369954,59.8757923088089,60.8737221806224,61.8716520524358,62.8695819242493,
63.8675117960628,63.9460441098254),.UNSPECIFIED.);
#751=B_SPLINE_CURVE_WITH_KNOTS('',3,(#32795,#32796,#32797,#32798,#32799,
#32800,#32801,#32802,#32803,#32804,#32805,#32806,#32807,#32808,#32809,#32810,
#32811,#32812,#32813,#32814,#32815,#32816),.UNSPECIFIED.,.F.,.F.,(4,3,3,
3,3,3,3,4),(-73.2075801278138,-72.8488806423841,-71.8509507705706,-70.8530208987571,
-69.8550910269437,-68.8571611551302,-67.8592312833167,-66.9243948206342),
 .UNSPECIFIED.);
#752=B_SPLINE_CURVE_WITH_KNOTS('',3,(#32817,#32818,#32819,#32820,#32821,
#32822,#32823,#32824,#32825,#32826,#32827,#32828,#32829,#32830,#32831,#32832,
#32833,#32834,#32835,#32836,#32837,#32838),.UNSPECIFIED.,.F.,.F.,(4,3,3,
3,3,3,3,4),(63.9460441098254,64.8654416678763,65.8633715396898,66.8613014115032,
67.8592312833167,68.8571611551302,69.8550910269437,70.229229417005),
 .UNSPECIFIED.);
#753=B_SPLINE_CURVE_WITH_KNOTS('',3,(#32843,#32844,#32845,#32846,#32847,
#32848,#32849,#32850,#32851,#32852,#32853,#32854,#32855,#32856,#32857,#32858,
#32859,#32860,#32861,#32862,#32863,#32864),.UNSPECIFIED.,.F.,.F.,(4,3,3,
3,3,3,3,4),(-79.4907654349934,-78.836459873265,-77.8385300014515,-76.840600129638,
-75.8426702578246,-74.8447403860111,-73.8468105141976,-73.2075801278138),
 .UNSPECIFIED.);
#754=B_SPLINE_CURVE_WITH_KNOTS('',3,(#32865,#32866,#32867,#32868,#32869,
#32870,#32871,#32872,#32873,#32874,#32875,#32876,#32877,#32878,#32879,#32880,
#32881,#32882,#32883,#32884,#32885,#32886),.UNSPECIFIED.,.F.,.F.,(4,3,3,
3,3,3,3,4),(70.229229417005,70.8530208987571,71.8509507705706,72.8488806423841,
73.8468105141976,74.8447403860111,75.8426702578246,76.5124147241846),
 .UNSPECIFIED.);
#755=B_SPLINE_CURVE_WITH_KNOTS('',3,(#32891,#32892,#32893,#32894,#32895,
#32896,#32897,#32898,#32899,#32900,#32901,#32902,#32903,#32904,#32905,#32906,
#32907,#32908,#32909,#32910,#32911,#32912),.UNSPECIFIED.,.F.,.F.,(4,3,3,
3,3,3,3,4),(-85.773950742173,-84.8240391041459,-83.8261092323324,-82.8281793605189,
-81.8302494887054,-80.832319616892,-79.8343897450785,-79.4907654349934),
 .UNSPECIFIED.);
#756=B_SPLINE_CURVE_WITH_KNOTS('',3,(#32913,#32914,#32915,#32916,#32917,
#32918,#32919,#32920,#32921,#32922,#32923,#32924,#32925,#32926,#32927,#32928,
#32929,#32930,#32931,#32932,#32933,#32934),.UNSPECIFIED.,.F.,.F.,(4,3,3,
3,3,3,3,4),(76.5124147241846,76.840600129638,77.8385300014515,78.836459873265,
79.8343897450785,80.832319616892,81.8302494887054,82.7956000313641),
 .UNSPECIFIED.);
#757=B_SPLINE_CURVE_WITH_KNOTS('',3,(#32939,#32940,#32941,#32942,#32943,
#32944,#32945,#32946,#32947,#32948,#32949,#32950,#32951,#32952,#32953,#32954,
#32955,#32956,#32957,#32958,#32959,#32960,#32961,#32962,#32963),
 .UNSPECIFIED.,.F.,.F.,(4,3,3,3,3,3,3,3,4),(-92.0571360493526,-91.8095482068402,
-90.8116183350268,-89.8136884632133,-88.8157585913998,-87.8178287195863,
-86.8198988477728,-85.8219689759594,-85.773950742173),.UNSPECIFIED.);
#758=B_SPLINE_CURVE_WITH_KNOTS('',3,(#32964,#32965,#32966,#32967,#32968,
#32969,#32970,#32971,#32972,#32973,#32974,#32975,#32976,#32977,#32978,#32979,
#32980,#32981,#32982,#32983,#32984,#32985,#32986,#32987,#32988),
 .UNSPECIFIED.,.F.,.F.,(4,3,3,3,3,3,3,3,4),(82.7956000313641,82.8281793605189,
83.8261092323324,84.8240391041459,85.8219689759594,86.8198988477728,87.8178287195863,
88.8157585913998,89.0787853385437),.UNSPECIFIED.);
#759=B_SPLINE_CURVE_WITH_KNOTS('',3,(#32993,#32994,#32995,#32996,#32997,
#32998,#32999,#33000,#33001,#33002,#33003,#33004,#33005,#33006,#33007,#33008,
#33009,#33010,#33011,#33012,#33013,#33014),.UNSPECIFIED.,.F.,.F.,(4,3,3,
3,3,3,3,4),(-98.3403213565322,-97.7971274377211,-96.7991975659076,-95.8012676940942,
-94.8033378222807,-93.8054079504672,-92.8074780786537,-92.0571360493526),
 .UNSPECIFIED.);
#760=B_SPLINE_CURVE_WITH_KNOTS('',3,(#33015,#33016,#33017,#33018,#33019,
#33020,#33021,#33022,#33023,#33024,#33025,#33026,#33027,#33028,#33029,#33030,
#33031,#33032,#33033,#33034,#33035,#33036),.UNSPECIFIED.,.F.,.F.,(4,3,3,
3,3,3,3,4),(89.0787853385437,89.8136884632133,90.8116183350268,91.8095482068402,
92.8074780786537,93.8054079504672,94.8033378222807,95.3619706457233),
 .UNSPECIFIED.);
#761=B_SPLINE_CURVE_WITH_KNOTS('',3,(#33041,#33042,#33043,#33044,#33045,
#33046,#33047,#33048,#33049,#33050,#33051,#33052,#33053,#33054,#33055,#33056,
#33057,#33058,#33059,#33060,#33061,#33062),.UNSPECIFIED.,.F.,.F.,(4,3,3,
3,3,3,3,4),(-104.623506663712,-103.784706668602,-102.786776796789,-101.788846924975,
-100.790917053162,-99.7929871813481,-98.7950573095346,-98.3403213565322),
 .UNSPECIFIED.);
#762=B_SPLINE_CURVE_WITH_KNOTS('',3,(#33063,#33064,#33065,#33066,#33067,
#33068,#33069,#33070,#33071,#33072,#33073,#33074,#33075,#33076,#33077,#33078,
#33079,#33080,#33081,#33082,#33083,#33084),.UNSPECIFIED.,.F.,.F.,(4,3,3,
3,3,3,3,4),(95.3619706457233,95.8012676940942,96.7991975659077,97.7971274377211,
98.7950573095346,99.7929871813481,100.790917053162,101.645155952903),
 .UNSPECIFIED.);
#763=B_SPLINE_CURVE_WITH_KNOTS('',3,(#33089,#33090,#33091,#33092,#33093,
#33094,#33095,#33096,#33097,#33098,#33099,#33100,#33101,#33102,#33103,#33104,
#33105,#33106,#33107,#33108,#33109,#33110,#33111,#33112,#33113),
 .UNSPECIFIED.,.F.,.F.,(4,3,3,3,3,3,3,3,4),(-110.906691970891,-110.770215771296,
-109.772285899483,-108.774356027669,-107.776426155856,-106.778496284042,
-105.780566412229,-104.782636540416,-104.623506663712),.UNSPECIFIED.);
#764=B_SPLINE_CURVE_WITH_KNOTS('',3,(#33114,#33115,#33116,#33117,#33118,
#33119,#33120,#33121,#33122,#33123,#33124,#33125,#33126,#33127,#33128,#33129,
#33130,#33131,#33132,#33133,#33134,#33135,#33136,#33137,#33138),
 .UNSPECIFIED.,.F.,.F.,(4,3,3,3,3,3,3,3,4),(101.645155952903,101.788846924975,
102.786776796789,103.784706668602,104.782636540416,105.780566412229,106.778496284042,
107.776426155856,107.928341260083),.UNSPECIFIED.);
#765=B_SPLINE_CURVE_WITH_KNOTS('',3,(#33143,#33144,#33145,#33146,#33147,
#33148,#33149,#33150,#33151,#33152,#33153,#33154,#33155,#33156,#33157,#33158,
#33159,#33160,#33161,#33162,#33163,#33164),.UNSPECIFIED.,.F.,.F.,(4,3,3,
3,3,3,3,4),(-117.189877278071,-116.757795002177,-115.759865130364,-114.76193525855,
-113.764005386737,-112.766075514923,-111.76814564311,-110.906691970891),
 .UNSPECIFIED.);
#766=B_SPLINE_CURVE_WITH_KNOTS('',3,(#33165,#33166,#33167,#33168,#33169,
#33170,#33171,#33172,#33173,#33174,#33175,#33176,#33177,#33178,#33179,#33180,
#33181,#33182,#33183,#33184,#33185,#33186),.UNSPECIFIED.,.F.,.F.,(4,3,3,
3,3,3,3,4),(107.928341260083,108.774356027669,109.772285899483,110.770215771296,
111.76814564311,112.766075514923,113.764005386737,114.211526567262),
 .UNSPECIFIED.);
#767=B_SPLINE_CURVE_WITH_KNOTS('',3,(#33191,#33192,#33193,#33194,#33195,
#33196,#33197,#33198,#33199,#33200,#33201,#33202,#33203,#33204,#33205,#33206,
#33207,#33208,#33209,#33210,#33211,#33212),.UNSPECIFIED.,.F.,.F.,(4,3,3,
3,3,3,3,4),(-123.473062585251,-122.745374233058,-121.747444361245,-120.749514489431,
-119.751584617618,-118.753654745804,-117.755724873991,-117.189877278071),
 .UNSPECIFIED.);
#768=B_SPLINE_CURVE_WITH_KNOTS('',3,(#33213,#33214,#33215,#33216,#33217,
#33218,#33219,#33220,#33221,#33222,#33223,#33224,#33225,#33226,#33227,#33228,
#33229,#33230,#33231,#33232,#33233,#33234),.UNSPECIFIED.,.F.,.F.,(4,3,3,
3,3,3,3,4),(114.211526567262,114.76193525855,115.759865130364,116.757795002177,
117.755724873991,118.753654745804,119.751584617618,120.494711874442),
 .UNSPECIFIED.);
#769=B_SPLINE_CURVE_WITH_KNOTS('',3,(#33239,#33240,#33241,#33242,#33243,
#33244,#33245,#33246,#33247,#33248,#33249,#33250,#33251,#33252,#33253,#33254,
#33255,#33256,#33257,#33258,#33259,#33260,#33261,#33262,#33263),
 .UNSPECIFIED.,.F.,.F.,(4,3,3,3,3,3,3,3,4),(-129.75624789243,-129.730883335753,
-128.732953463939,-127.735023592126,-126.737093720312,-125.739163848499,
-124.741233976685,-123.743304104872,-123.473062585251),.UNSPECIFIED.);
#770=B_SPLINE_CURVE_WITH_KNOTS('',3,(#33264,#33265,#33266,#33267,#33268,
#33269,#33270,#33271,#33272,#33273,#33274,#33275,#33276,#33277,#33278,#33279,
#33280,#33281,#33282,#33283,#33284,#33285,#33286,#33287,#33288),
 .UNSPECIFIED.,.F.,.F.,(4,3,3,3,3,3,3,3,4),(120.494711874442,120.749514489431,
121.747444361245,122.745374233058,123.743304104872,124.741233976685,125.739163848499,
126.737093720312,126.777897181621),.UNSPECIFIED.);
#771=B_SPLINE_CURVE_WITH_KNOTS('',3,(#33293,#33294,#33295,#33296,#33297,
#33298,#33299,#33300,#33301,#33302,#33303,#33304,#33305,#33306,#33307,#33308,
#33309,#33310,#33311,#33312,#33313,#33314),.UNSPECIFIED.,.F.,.F.,(4,3,3,
3,3,3,3,4),(-136.03943319961,-135.718462566633,-134.72053269482,-133.722602823006,
-132.724672951193,-131.72674307938,-130.728813207566,-129.75624789243),
 .UNSPECIFIED.);
#772=B_SPLINE_CURVE_WITH_KNOTS('',3,(#33315,#33316,#33317,#33318,#33319,
#33320,#33321,#33322,#33323,#33324,#33325,#33326,#33327,#33328,#33329,#33330,
#33331,#33332,#33333,#33334,#33335,#33336),.UNSPECIFIED.,.F.,.F.,(4,3,3,
3,3,3,3,4),(126.777897181621,127.735023592126,128.732953463939,129.730883335753,
130.728813207566,131.72674307938,132.724672951193,133.061082488801),
 .UNSPECIFIED.);
#773=B_SPLINE_CURVE_WITH_KNOTS('',3,(#33342,#33343,#33344,#33345,#33346,
#33347),.UNSPECIFIED.,.F.,.F.,(4,1,1,4),(147.65485471872,148.331813957558,
149.329743829371,150.258393311533),.UNSPECIFIED.);
#774=B_SPLINE_CURVE_WITH_KNOTS('',3,(#33350,#33351,#33352,#33353,#33354),
 .UNSPECIFIED.,.F.,.F.,(4,1,4),(147.65485471872,148.020768976627,149.018698848441),
 .UNSPECIFIED.);
#775=B_SPLINE_CURVE_WITH_KNOTS('',3,(#33359,#33360,#33361,#33362,#33363,
#33364,#33365,#33366,#33367,#33368),.UNSPECIFIED.,.F.,.F.,(4,1,1,1,1,1,
1,4),(141.371669411541,142.344234726677,143.34216459849,144.340094470304,
145.338024342117,146.335954213931,147.333884085744,147.65485471872),
 .UNSPECIFIED.);
#776=B_SPLINE_CURVE_WITH_KNOTS('',3,(#33369,#33370,#33371,#33372,#33373,
#33374,#33375,#33376,#33377,#33378),.UNSPECIFIED.,.F.,.F.,(4,1,1,1,1,1,
1,4),(141.371669411541,142.033189745746,143.03111961756,144.029049489373,
145.026979361187,146.024909233,147.022839104814,147.65485471872),
 .UNSPECIFIED.);
#777=B_SPLINE_CURVE_WITH_KNOTS('',3,(#33383,#33384,#33385,#33386,#33387,
#33388,#33389,#33390,#33391,#33392,#33393),.UNSPECIFIED.,.F.,.F.,(4,1,1,
1,1,1,1,1,4),(135.088484104361,135.358725623982,136.356655495796,137.354585367609,
138.352515239423,139.350445111236,140.34837498305,141.346304854863,141.371669411541),
 .UNSPECIFIED.);
#778=B_SPLINE_CURVE_WITH_KNOTS('',3,(#33394,#33395,#33396,#33397,#33398,
#33399,#33400,#33401,#33402,#33403),.UNSPECIFIED.,.F.,.F.,(4,1,1,1,1,1,
1,4),(135.088484104361,136.045610514865,137.043540386679,138.041470258492,
139.039400130306,140.037330002119,141.035259873933,141.371669411541),
 .UNSPECIFIED.);
#779=B_SPLINE_CURVE_WITH_KNOTS('',3,(#33408,#33409,#33410,#33411,#33412,
#33413,#33414,#33415,#33416,#33417),.UNSPECIFIED.,.F.,.F.,(4,1,1,1,1,1,
1,4),(128.805298797182,129.371146393101,130.369076264915,131.367006136728,
132.364936008542,133.362865880355,134.360795752169,135.088484104361),
 .UNSPECIFIED.);
#780=B_SPLINE_CURVE_WITH_KNOTS('',3,(#33418,#33419,#33420,#33421,#33422,
#33423,#33424,#33425,#33426,#33427,#33428),.UNSPECIFIED.,.F.,.F.,(4,1,1,
1,1,1,1,1,4),(128.805298797182,129.060101412171,130.058031283984,131.055961155798,
132.053891027611,133.051820899425,134.049750771238,135.047680643052,135.088484104361),
 .UNSPECIFIED.);
#781=B_SPLINE_CURVE_WITH_KNOTS('',3,(#33433,#33434,#33435,#33436,#33437,
#33438,#33439,#33440,#33441,#33442),.UNSPECIFIED.,.F.,.F.,(4,1,1,1,1,1,
1,4),(122.522113490002,123.383567162221,124.381497034034,125.379426905847,
126.377356777661,127.375286649474,128.373216521288,128.805298797182),
 .UNSPECIFIED.);
#782=B_SPLINE_CURVE_WITH_KNOTS('',3,(#33443,#33444,#33445,#33446,#33447,
#33448,#33449,#33450,#33451,#33452),.UNSPECIFIED.,.F.,.F.,(4,1,1,1,1,1,
1,4),(122.522113490002,123.07252218129,124.070452053104,125.068381924917,
126.066311796731,127.064241668544,128.062171540357,128.805298797182),
 .UNSPECIFIED.);
#783=B_SPLINE_CURVE_WITH_KNOTS('',3,(#33457,#33458,#33459,#33460,#33461,
#33462,#33463,#33464,#33465,#33466,#33467),.UNSPECIFIED.,.F.,.F.,(4,1,1,
1,1,1,1,1,4),(116.238928182822,116.398058059526,117.39598793134,118.393917803153,
119.391847674967,120.38977754678,121.387707418594,122.385637290407,122.522113490002),
 .UNSPECIFIED.);
#784=B_SPLINE_CURVE_WITH_KNOTS('',3,(#33468,#33469,#33470,#33471,#33472,
#33473,#33474,#33475,#33476,#33477),.UNSPECIFIED.,.F.,.F.,(4,1,1,1,1,1,
1,4),(116.238928182822,117.084942950409,118.082872822223,119.080802694036,
120.07873256585,121.076662437663,122.074592309477,122.522113490002),
 .UNSPECIFIED.);
#785=B_SPLINE_CURVE_WITH_KNOTS('',3,(#33482,#33483,#33484,#33485,#33486,
#33487,#33488,#33489,#33490,#33491),.UNSPECIFIED.,.F.,.F.,(4,1,1,1,1,1,
1,4),(109.955742875643,110.410478828645,111.408408700459,112.406338572272,
113.404268444086,114.402198315899,115.400128187713,116.238928182822),
 .UNSPECIFIED.);
#786=B_SPLINE_CURVE_WITH_KNOTS('',3,(#33492,#33493,#33494,#33495,#33496,
#33497,#33498,#33499,#33500,#33501,#33502),.UNSPECIFIED.,.F.,.F.,(4,1,1,
1,1,1,1,1,4),(109.955742875643,110.099433847715,111.097363719528,112.095293591342,
113.093223463155,114.091153334969,115.089083206782,116.087013078596,116.238928182822),
 .UNSPECIFIED.);
#787=B_SPLINE_CURVE_WITH_KNOTS('',3,(#33507,#33508,#33509,#33510,#33511,
#33512,#33513,#33514,#33515,#33516),.UNSPECIFIED.,.F.,.F.,(4,1,1,1,1,1,
1,4),(103.672557568463,104.422899597764,105.420829469578,106.418759341391,
107.416689213205,108.414619085018,109.412548956832,109.955742875643),
 .UNSPECIFIED.);
#788=B_SPLINE_CURVE_WITH_KNOTS('',3,(#33517,#33518,#33519,#33520,#33521,
#33522,#33523,#33524,#33525,#33526),.UNSPECIFIED.,.F.,.F.,(4,1,1,1,1,1,
1,4),(103.672557568463,104.111854616834,105.109784488647,106.107714360461,
107.105644232274,108.103574104088,109.101503975901,109.955742875643),
 .UNSPECIFIED.);
#789=B_SPLINE_CURVE_WITH_KNOTS('',3,(#33531,#33532,#33533,#33534,#33535,
#33536,#33537,#33538,#33539,#33540,#33541),.UNSPECIFIED.,.F.,.F.,(4,1,1,
1,1,1,1,1,4),(97.3893722612836,97.43739049507,98.4353203668835,99.433250238697,
100.43118011051,101.429109982324,102.427039854137,103.424969725951,103.672557568463),
 .UNSPECIFIED.);
#790=B_SPLINE_CURVE_WITH_KNOTS('',3,(#33542,#33543,#33544,#33545,#33546,
#33547,#33548,#33549,#33550,#33551),.UNSPECIFIED.,.F.,.F.,(4,1,1,1,1,1,
1,4),(97.3893722612836,98.1242753859531,99.1222052577666,100.12013512958,
101.118065001394,102.115994873207,103.11392474502,103.672557568463),
 .UNSPECIFIED.);
#791=B_SPLINE_CURVE_WITH_KNOTS('',3,(#33556,#33557,#33558,#33559,#33560,
#33561,#33562,#33563,#33564,#33565),.UNSPECIFIED.,.F.,.F.,(4,1,1,1,1,1,
1,4),(91.106186954104,91.4498112641891,92.4477411360026,93.4456710078161,
94.4436008796296,95.441530751443,96.4394606232565,97.3893722612836),
 .UNSPECIFIED.);
#792=B_SPLINE_CURVE_WITH_KNOTS('',3,(#33566,#33567,#33568,#33569,#33570,
#33571,#33572,#33573,#33574,#33575,#33576),.UNSPECIFIED.,.F.,.F.,(4,1,1,
1,1,1,1,1,4),(91.106186954104,91.1387662832587,92.1366961550722,93.1346260268857,
94.1325558986991,95.1304857705126,96.1284156423261,97.1263455141396,97.3893722612836),
 .UNSPECIFIED.);
#793=B_SPLINE_CURVE_WITH_KNOTS('',3,(#33581,#33582,#33583,#33584,#33585,
#33586,#33587,#33588,#33589,#33590),.UNSPECIFIED.,.F.,.F.,(4,1,1,1,1,1,
1,4),(84.8230016469244,85.4622320333082,86.4601619051217,87.4580917769352,
88.4560216487487,89.4539515205621,90.4518813923756,91.106186954104),
 .UNSPECIFIED.);
#794=B_SPLINE_CURVE_WITH_KNOTS('',3,(#33591,#33592,#33593,#33594,#33595,
#33596,#33597,#33598,#33599,#33600),.UNSPECIFIED.,.F.,.F.,(4,1,1,1,1,1,
1,4),(84.8230016469244,85.1511870523778,86.1491169241913,87.1470467960048,
88.1449766678183,89.1429065396317,90.1408364114452,91.106186954104),
 .UNSPECIFIED.);
#795=B_SPLINE_CURVE_WITH_KNOTS('',3,(#33605,#33606,#33607,#33608,#33609,
#33610,#33611,#33612,#33613,#33614),.UNSPECIFIED.,.F.,.F.,(4,1,1,1,1,1,
1,4),(78.5398163397449,79.4746528024273,80.4725826742408,81.4705125460543,
82.4684424178678,83.4663722896813,84.4643021614947,84.8230016469244),
 .UNSPECIFIED.);
#796=B_SPLINE_CURVE_WITH_KNOTS('',3,(#33615,#33616,#33617,#33618,#33619,
#33620,#33621,#33622,#33623,#33624),.UNSPECIFIED.,.F.,.F.,(4,1,1,1,1,1,
1,4),(78.5398163397449,79.1636078214969,80.1615376933104,81.1594675651239,
82.1573974369374,83.1553273087509,84.1532571805643,84.8230016469244),
 .UNSPECIFIED.);
#797=B_SPLINE_CURVE_WITH_KNOTS('',3,(#33629,#33630,#33631,#33632,#33633,
#33634,#33635,#33636,#33637,#33638,#33639),.UNSPECIFIED.,.F.,.F.,(4,1,1,
1,1,1,1,1,4),(72.2566310325653,72.489143699733,73.4870735715464,74.4850034433599,
75.4829333151734,76.4808631869869,77.4787930588004,78.4767229306139,78.5398163397449),
 .UNSPECIFIED.);
#798=B_SPLINE_CURVE_WITH_KNOTS('',3,(#33640,#33641,#33642,#33643,#33644,
#33645,#33646,#33647,#33648,#33649),.UNSPECIFIED.,.F.,.F.,(4,1,1,1,1,1,
1,4),(72.2566310325653,73.176028590616,74.1739584624295,75.171888334243,
76.1698182060565,77.16774807787,78.1656779496834,78.5398163397449),
 .UNSPECIFIED.);
#799=B_SPLINE_CURVE_WITH_KNOTS('',3,(#33654,#33655,#33656,#33657,#33658,
#33659,#33660,#33661,#33662,#33663),.UNSPECIFIED.,.F.,.F.,(4,1,1,1,1,1,
1,4),(65.9734457253856,66.5015644688521,67.4994943406656,68.497424212479,
69.4953540842925,70.493283956106,71.4912138279195,72.2566310325653),
 .UNSPECIFIED.);
#800=B_SPLINE_CURVE_WITH_KNOTS('',3,(#33664,#33665,#33666,#33667,#33668,
#33669,#33670,#33671,#33672,#33673,#33674),.UNSPECIFIED.,.F.,.F.,(4,1,1,
1,1,1,1,1,4),(65.9734457253856,66.1905194879217,67.1884493597351,68.1863792315486,
69.1843091033621,70.1822389751756,71.1801688469891,72.1780987188026,72.2566310325653),
 .UNSPECIFIED.);
#801=B_SPLINE_CURVE_WITH_KNOTS('',3,(#33679,#33680,#33681,#33682,#33683,
#33684,#33685,#33686,#33687,#33688),.UNSPECIFIED.,.F.,.F.,(4,1,1,1,1,1,
1,4),(59.6902604182061,60.5139852379712,61.5119151097847,62.5098449815982,
63.5077748534116,64.5057047252251,65.5036345970386,65.9734457253856),
 .UNSPECIFIED.);
#802=B_SPLINE_CURVE_WITH_KNOTS('',3,(#33689,#33690,#33691,#33692,#33693,
#33694,#33695,#33696,#33697,#33698),.UNSPECIFIED.,.F.,.F.,(4,1,1,1,1,1,
1,4),(59.6902604182061,60.2029402570408,61.2008701288543,62.1988000006677,
63.1967298724812,64.1946597442947,65.1925896161082,65.9734457253856),
 .UNSPECIFIED.);
#803=B_SPLINE_CURVE_WITH_KNOTS('',3,(#33703,#33704,#33705,#33706,#33707,
#33708,#33709,#33710,#33711,#33712,#33713),.UNSPECIFIED.,.F.,.F.,(4,1,1,
1,1,1,1,1,4),(53.4070751110265,53.5284761352768,54.5264060070903,55.5243358789038,
56.5222657507173,57.5201956225308,58.5181254943442,59.5160553661577,59.6902604182061),
 .UNSPECIFIED.);
#804=B_SPLINE_CURVE_WITH_KNOTS('',3,(#33714,#33715,#33716,#33717,#33718,
#33719,#33720,#33721,#33722,#33723),.UNSPECIFIED.,.F.,.F.,(4,1,1,1,1,1,
1,4),(53.4070751110265,54.2153610261599,55.2132908979734,56.2112207697869,
57.2091506416003,58.2070805134138,59.2050103852273,59.6902604182061),
 .UNSPECIFIED.);
#805=B_SPLINE_CURVE_WITH_KNOTS('',3,(#33728,#33729,#33730,#33731,#33732,
#33733,#33734,#33735,#33736,#33737),.UNSPECIFIED.,.F.,.F.,(4,1,1,1,1,1,
1,4),(47.1238898038469,47.540896904396,48.5388267762094,49.5367566480229,
50.5346865198364,51.5326163916499,52.5305462634634,53.4070751110265),
 .UNSPECIFIED.);
#806=B_SPLINE_CURVE_WITH_KNOTS('',3,(#33738,#33739,#33740,#33741,#33742,
#33743,#33744,#33745,#33746,#33747,#33748),.UNSPECIFIED.,.F.,.F.,(4,1,1,
1,1,1,1,1,4),(47.1238898038469,47.2298519234655,48.227781795279,49.2257116670925,
50.223641538906,51.2215714107194,52.2195012825329,53.2174311543464,53.4070751110265),
 .UNSPECIFIED.);
#807=B_SPLINE_CURVE_WITH_KNOTS('',3,(#33753,#33754,#33755,#33756,#33757,
#33758,#33759,#33760,#33761,#33762),.UNSPECIFIED.,.F.,.F.,(4,1,1,1,1,1,
1,4),(40.8407044966673,41.5533176735151,42.5512475453285,43.549177417142,
44.5471072889555,45.545037160769,46.5429670325825,47.1238898038469),
 .UNSPECIFIED.);
#808=B_SPLINE_CURVE_WITH_KNOTS('',3,(#33763,#33764,#33765,#33766,#33767,
#33768,#33769,#33770,#33771,#33772),.UNSPECIFIED.,.F.,.F.,(4,1,1,1,1,1,
1,4),(40.8407044966673,41.2422726925846,42.2402025643981,43.2381324362116,
44.2360623080251,45.2339921798386,46.231922051652,47.1238898038469),
 .UNSPECIFIED.);
#809=B_SPLINE_CURVE_WITH_KNOTS('',3,(#33777,#33778,#33779,#33780,#33781,
#33782,#33783,#33784,#33785,#33786,#33787),.UNSPECIFIED.,.F.,.F.,(4,1,1,
1,1,1,1,1,4),(34.5575191894877,34.5678085708207,35.5657384426342,36.5636683144477,
37.5615981862611,38.5595280580746,39.5574579298881,40.5553878017016,40.8407044966673),
 .UNSPECIFIED.);
#810=B_SPLINE_CURVE_WITH_KNOTS('',3,(#33788,#33789,#33790,#33791,#33792,
#33793,#33794,#33795,#33796,#33797),.UNSPECIFIED.,.F.,.F.,(4,1,1,1,1,1,
1,4),(34.5575191894877,35.2546934617038,36.2526233335172,37.2505532053307,
38.2484830771442,39.2464129489577,40.2443428207712,40.8407044966673),
 .UNSPECIFIED.);
#811=B_SPLINE_CURVE_WITH_KNOTS('',3,(#33802,#33803,#33804,#33805,#33806,
#33807,#33808,#33809,#33810,#33811),.UNSPECIFIED.,.F.,.F.,(4,1,1,1,1,1,
1,4),(28.2743338823081,28.5802293399398,29.5781592117533,30.5760890835668,
31.5740189553803,32.5719488271937,33.5698786990072,34.5575191894877),
 .UNSPECIFIED.);
#812=B_SPLINE_CURVE_WITH_KNOTS('',3,(#33812,#33813,#33814,#33815,#33816,
#33817,#33818,#33819,#33820,#33821),.UNSPECIFIED.,.F.,.F.,(4,1,1,1,1,1,
1,4),(28.2743338823081,29.2671142308229,30.2650441026364,31.2629739744498,
32.2609038462633,33.2588337180768,34.2567635898903,34.5575191894877),
 .UNSPECIFIED.);
#813=B_SPLINE_CURVE_WITH_KNOTS('',3,(#33826,#33827,#33828,#33829,#33830,
#33831,#33832,#33833,#33834,#33835),.UNSPECIFIED.,.F.,.F.,(4,1,1,1,1,1,
1,4),(21.9911485751285,22.5926501090589,23.5905799808724,24.5885098526859,
25.5864397244994,26.5843695963128,27.5822994681263,28.2743338823081),
 .UNSPECIFIED.);
#814=B_SPLINE_CURVE_WITH_KNOTS('',3,(#33836,#33837,#33838,#33839,#33840,
#33841,#33842,#33843,#33844,#33845,#33846),.UNSPECIFIED.,.F.,.F.,(4,1,1,
1,1,1,1,1,4),(21.9911485751285,22.2816051281285,23.279534999942,24.2774648717555,
25.2753947435689,26.2733246153824,27.2712544871959,28.2691843590094,28.2743338823081),
 .UNSPECIFIED.);
#815=B_SPLINE_CURVE_WITH_KNOTS('',3,(#33851,#33852,#33853,#33854,#33855,
#33856,#33857,#33858,#33859,#33860),.UNSPECIFIED.,.F.,.F.,(4,1,1,1,1,1,
1,4),(15.7079632679489,16.605070878178,17.6030007499915,18.600930621805,
19.5988604936185,20.596790365432,21.5947202372454,21.9911485751285),
 .UNSPECIFIED.);
#816=B_SPLINE_CURVE_WITH_KNOTS('',3,(#33861,#33862,#33863,#33864,#33865,
#33866,#33867,#33868,#33869,#33870),.UNSPECIFIED.,.F.,.F.,(4,1,1,1,1,1,
1,4),(15.7079632679489,16.2940258972476,17.2919557690611,18.2898856408746,
19.2878155126881,20.2857453845015,21.283675256315,21.9911485751285),
 .UNSPECIFIED.);
#817=B_SPLINE_CURVE_WITH_KNOTS('',3,(#33873,#33874,#33875,#33876,#33877,
#33878,#33879,#33880,#33881,#33882,#33883,#33884,#33885,#33886,#33887,#33888,
#33889,#33890,#33891,#33892,#33893,#33894,#33895,#33896,#33897,#33898,#33899,
#33900,#33901,#33902,#33903,#33904,#33905,#33906,#33907,#33908,#33909,#33910,
#33911,#33912,#33913,#33914,#33915,#33916,#33917,#33918,#33919,#33920,#33921,
#33922,#33923,#33924),.UNSPECIFIED.,.F.,.F.,(4,3,3,3,3,3,3,3,3,3,3,3,3,
3,3,3,3,4),(-0.366397579005835,-0.355436711127808,-0.328765885113455,-0.316053385254379,
-0.292504079879806,-0.280231653992808,-0.245255630742482,-0.21857122152355,
-0.207922214642856,-0.187195667096964,-0.163796208709843,-0.149553713974392,
-0.138748641693171,-0.104061481269878,-0.0827650289191262,-0.0667799803750929,
-0.0282862380303849,0.),.UNSPECIFIED.);
#818=B_SPLINE_CURVE_WITH_KNOTS('',3,(#33929,#33930,#33931,#33932,#33933,
#33934,#33935,#33936,#33937,#33938,#33939,#33940,#33941,#33942,#33943,#33944,
#33945,#33946,#33947,#33948,#33949,#33950,#33951,#33952,#33953,#33954,#33955,
#33956,#33957,#33958,#33959,#33960,#33961,#33962,#33963,#33964,#33965,#33966,
#33967,#33968,#33969,#33970,#33971,#33972,#33973,#33974,#33975,#33976,#33977,
#33978,#33979,#33980),.UNSPECIFIED.,.F.,.F.,(4,3,3,3,3,3,3,3,3,3,3,3,3,
3,3,3,3,4),(-0.364629307890686,-0.351116863859227,-0.324664676768481,-0.311283134135643,
-0.274452551481962,-0.262271743112635,-0.225606031128057,-0.200971540009699,
-0.186293214263739,-0.166278288083988,-0.130542983888158,-0.11937084036021,
-0.0895281302701574,-0.0729763635778195,-0.0626462517339964,-0.0518843227274219,
-0.0196324840529713,0.),.UNSPECIFIED.);
#819=B_SPLINE_CURVE_WITH_KNOTS('',3,(#34557,#34558,#34559,#34560,#34561,
#34562,#34563,#34564,#34565,#34566,#34567,#34568,#34569,#34570,#34571,#34572,
#34573,#34574,#34575),.UNSPECIFIED.,.F.,.F.,(4,3,3,3,3,3,4),(133.061082488801,
133.722602823006,134.72053269482,135.718462566633,136.716392438447,137.71432231026,
138.642971792423),.UNSPECIFIED.);
#820=B_SPLINE_CURVE_WITH_KNOTS('',3,(#34577,#34578,#34579,#34580,#34581,
#34582,#34583,#34584,#34585,#34586,#34587,#34588,#34589,#34590,#34591,#34592,
#34593,#34594,#34595,#34596,#34597,#34598,#34599,#34600,#34601,#34602,#34603,
#34604,#34605,#34606,#34607,#34608,#34609,#34610,#34611,#34612,#34613,#34614,
#34615,#34616,#34617,#34618,#34619,#34620,#34621,#34622,#34623,#34624,#34625,
#34626,#34627,#34628),.UNSPECIFIED.,.F.,.F.,(4,3,3,3,3,3,3,3,3,3,3,3,3,
3,3,3,3,4),(-0.366397579005848,-0.355436711127817,-0.328765885668864,-0.316053387324444,
-0.292503977462896,-0.2802316187117,-0.245255597344971,-0.218571154973266,
-0.207922184331738,-0.187195667096965,-0.163796208709844,-0.149553707012105,
-0.138748635975912,-0.104061476981934,-0.0827650184680586,-0.066779980749083,
-0.0282862336556402,0.),.UNSPECIFIED.);
#821=B_SPLINE_CURVE_WITH_KNOTS('',3,(#34629,#34630,#34631,#34632,#34633,
#34634,#34635,#34636,#34637),.UNSPECIFIED.,.F.,.F.,(4,1,1,1,1,1,4),(10.3757270560179,
11.3043765381802,12.3023064099937,13.3002362818072,14.2981661536207,15.2960960254341,
15.7079632679489),.UNSPECIFIED.);
#822=B_SPLINE_CURVE_WITH_KNOTS('',3,(#34643,#34644,#34645,#34646,#34647,
#34648,#34649,#34650,#34651,#34652,#34653,#34654,#34655,#34656,#34657,#34658,
#34659,#34660,#34661,#34662,#34663,#34664,#34665,#34666,#34667,#34668,#34669,
#34670,#34671,#34672,#34673,#34674,#34675,#34676,#34677,#34678,#34679,#34680,
#34681,#34682,#34683,#34684,#34685,#34686,#34687,#34688,#34689,#34690,#34691,
#34692,#34693,#34694),.UNSPECIFIED.,.F.,.F.,(4,3,3,3,3,3,3,3,3,3,3,3,3,
3,3,3,3,4),(-0.364629307890667,-0.351116863859215,-0.324664673225363,-0.311283119253959,
-0.274452522062154,-0.262271701636058,-0.22560598629008,-0.200971428165319,
-0.186293220294034,-0.166278288083978,-0.130542982670707,-0.119370841196389,
-0.0895281308972919,-0.0729763658959894,-0.0626462592378975,-0.0518843246587979,
-0.0196325022123193,0.),.UNSPECIFIED.);
#823=B_SPLINE_CURVE_WITH_KNOTS('',3,(#34697,#34698,#34699,#34700,#34701,
#34702,#34703,#34704),.UNSPECIFIED.,.F.,.F.,(4,1,1,1,1,4),(11.6154215191106,
12.6133513909241,13.6112812627376,14.6092111345511,15.6071410063646,15.7079632679489),
 .UNSPECIFIED.);
#824=B_SPLINE_CURVE_WITH_KNOTS('',3,(#35281,#35282,#35283,#35284,#35285,
#35286,#35287,#35288,#35289,#35290,#35291,#35292,#35293,#35294,#35295,#35296),
 .UNSPECIFIED.,.F.,.F.,(4,3,3,3,3,4),(-140.708111925701,-139.710182053887,
-138.712252182074,-137.71432231026,-136.716392438447,-136.03943319961),
 .UNSPECIFIED.);
#1029=CYLINDRICAL_SURFACE('',#17333,0.1954);
#1030=CYLINDRICAL_SURFACE('',#17335,0.1954);
#1031=CYLINDRICAL_SURFACE('',#17336,0.1954);
#1032=CYLINDRICAL_SURFACE('',#17337,0.1954);
#1033=CYLINDRICAL_SURFACE('',#17338,0.1954);
#1034=CYLINDRICAL_SURFACE('',#17339,0.1954);
#1035=CYLINDRICAL_SURFACE('',#17340,0.1954);
#1036=CYLINDRICAL_SURFACE('',#17341,0.1954);
#1037=CYLINDRICAL_SURFACE('',#17342,0.1954);
#1038=CYLINDRICAL_SURFACE('',#17343,0.1954);
#1039=CYLINDRICAL_SURFACE('',#17344,0.1954);
#1040=CYLINDRICAL_SURFACE('',#17345,0.1954);
#1041=CYLINDRICAL_SURFACE('',#17346,0.1954);
#1042=CYLINDRICAL_SURFACE('',#17347,0.1954);
#1043=CYLINDRICAL_SURFACE('',#17348,0.1954);
#1044=CYLINDRICAL_SURFACE('',#17349,0.1954);
#1045=CYLINDRICAL_SURFACE('',#17350,0.1954);
#1046=CYLINDRICAL_SURFACE('',#17351,0.1954);
#1047=CYLINDRICAL_SURFACE('',#17352,0.1954);
#1048=CYLINDRICAL_SURFACE('',#17353,0.1954);
#1049=CYLINDRICAL_SURFACE('',#17354,0.1954);
#1050=CYLINDRICAL_SURFACE('',#17355,0.1954);
#1051=CYLINDRICAL_SURFACE('',#17356,0.15555);
#1052=CYLINDRICAL_SURFACE('',#17358,0.15555);
#1053=CYLINDRICAL_SURFACE('',#17359,0.15555);
#1054=CYLINDRICAL_SURFACE('',#17360,0.15555);
#1055=CYLINDRICAL_SURFACE('',#17361,0.15555);
#1056=CYLINDRICAL_SURFACE('',#17362,0.15555);
#1057=CYLINDRICAL_SURFACE('',#17363,0.15555);
#1058=CYLINDRICAL_SURFACE('',#17364,0.15555);
#1059=CYLINDRICAL_SURFACE('',#17365,0.15555);
#1060=CYLINDRICAL_SURFACE('',#17366,0.15555);
#1061=CYLINDRICAL_SURFACE('',#17367,0.15555);
#1062=CYLINDRICAL_SURFACE('',#17368,0.15555);
#1063=CYLINDRICAL_SURFACE('',#17369,0.15555);
#1064=CYLINDRICAL_SURFACE('',#17370,0.15555);
#1065=CYLINDRICAL_SURFACE('',#17371,0.15555);
#1066=CYLINDRICAL_SURFACE('',#17372,0.15555);
#1067=CYLINDRICAL_SURFACE('',#17373,0.15555);
#1068=CYLINDRICAL_SURFACE('',#17374,0.15555);
#1069=CYLINDRICAL_SURFACE('',#17375,0.15555);
#1070=CYLINDRICAL_SURFACE('',#17376,0.15555);
#1071=CYLINDRICAL_SURFACE('',#17377,0.15555);
#1072=CYLINDRICAL_SURFACE('',#17378,0.15555);
#1073=CYLINDRICAL_SURFACE('',#17386,0.15555);
#1074=CYLINDRICAL_SURFACE('',#17391,0.1954);
#1075=CYLINDRICAL_SURFACE('',#17545,0.35);
#1076=CYLINDRICAL_SURFACE('',#17547,0.35);
#1077=CYLINDRICAL_SURFACE('',#17549,0.35);
#1078=CYLINDRICAL_SURFACE('',#17551,0.35);
#1079=CYLINDRICAL_SURFACE('',#17553,0.35);
#1080=CYLINDRICAL_SURFACE('',#17555,0.35);
#1081=CYLINDRICAL_SURFACE('',#17557,0.35);
#1082=CYLINDRICAL_SURFACE('',#17559,0.35);
#1083=CYLINDRICAL_SURFACE('',#17561,0.35);
#1084=CYLINDRICAL_SURFACE('',#17563,0.35);
#1085=CYLINDRICAL_SURFACE('',#17565,0.35);
#1086=CYLINDRICAL_SURFACE('',#17567,0.35);
#1087=CYLINDRICAL_SURFACE('',#17569,0.35);
#1088=CYLINDRICAL_SURFACE('',#17571,0.35);
#1089=CYLINDRICAL_SURFACE('',#17573,0.35);
#1090=CYLINDRICAL_SURFACE('',#17575,0.35);
#1091=CYLINDRICAL_SURFACE('',#17577,0.35);
#1092=CYLINDRICAL_SURFACE('',#17579,0.35);
#1093=CYLINDRICAL_SURFACE('',#17581,0.35);
#1094=CYLINDRICAL_SURFACE('',#17583,0.35);
#1095=CYLINDRICAL_SURFACE('',#17585,0.35);
#1096=CYLINDRICAL_SURFACE('',#17587,0.35);
#1097=CYLINDRICAL_SURFACE('',#17589,0.35);
#1098=CYLINDRICAL_SURFACE('',#17591,0.35);
#1099=CYLINDRICAL_SURFACE('',#17593,0.35);
#1100=CYLINDRICAL_SURFACE('',#17595,0.35);
#1101=CYLINDRICAL_SURFACE('',#17597,0.35);
#1102=CYLINDRICAL_SURFACE('',#17599,0.35);
#1103=CYLINDRICAL_SURFACE('',#17601,0.35);
#1104=CYLINDRICAL_SURFACE('',#17603,0.35);
#1105=CYLINDRICAL_SURFACE('',#17605,0.35);
#1106=CYLINDRICAL_SURFACE('',#17607,0.35);
#1107=CYLINDRICAL_SURFACE('',#17609,0.35);
#1108=CYLINDRICAL_SURFACE('',#17611,0.35);
#1109=CYLINDRICAL_SURFACE('',#17613,0.35);
#1110=CYLINDRICAL_SURFACE('',#17615,0.35);
#1202=FACE_BOUND('',#3403,.T.);
#1203=FACE_BOUND('',#3547,.T.);
#1518=CIRCLE('',#17334,0.1954);
#1519=CIRCLE('',#17357,0.15555);
#1520=CIRCLE('',#17380,0.1954);
#1521=CIRCLE('',#17381,0.1954);
#1522=CIRCLE('',#17383,0.1954);
#1523=CIRCLE('',#17384,0.1954);
#1524=CIRCLE('',#17385,0.15555);
#1525=CIRCLE('',#17388,0.02);
#1526=CIRCLE('',#17389,0.2154);
#1527=CIRCLE('',#17390,0.1954);
#1528=CIRCLE('',#17393,0.35);
#1529=CIRCLE('',#17394,0.35);
#1530=CIRCLE('',#17395,0.35);
#1531=CIRCLE('',#17396,0.35);
#1532=CIRCLE('',#17397,0.35);
#1533=CIRCLE('',#17398,0.35);
#1534=CIRCLE('',#17399,0.35);
#1535=CIRCLE('',#17400,0.35);
#1536=CIRCLE('',#17401,0.35);
#1537=CIRCLE('',#17402,0.35);
#1538=CIRCLE('',#17403,0.35);
#1539=CIRCLE('',#17404,0.35);
#1540=CIRCLE('',#17405,0.35);
#1541=CIRCLE('',#17406,0.35);
#1542=CIRCLE('',#17407,0.35);
#1543=CIRCLE('',#17408,0.35);
#1544=CIRCLE('',#17409,0.35);
#1545=CIRCLE('',#17410,0.35);
#1546=CIRCLE('',#17411,0.35);
#1547=CIRCLE('',#17412,0.35);
#1548=CIRCLE('',#17413,0.35);
#1549=CIRCLE('',#17414,0.35);
#1550=CIRCLE('',#17415,0.35);
#1551=CIRCLE('',#17416,0.35);
#1552=CIRCLE('',#17417,0.35);
#1553=CIRCLE('',#17418,0.35);
#1554=CIRCLE('',#17419,0.35);
#1555=CIRCLE('',#17420,0.35);
#1556=CIRCLE('',#17421,0.35);
#1557=CIRCLE('',#17422,0.35);
#1558=CIRCLE('',#17423,0.35);
#1559=CIRCLE('',#17424,0.35);
#1560=CIRCLE('',#17425,0.35);
#1561=CIRCLE('',#17426,0.35);
#1562=CIRCLE('',#17427,0.35);
#1563=CIRCLE('',#17428,0.35);
#1564=CIRCLE('',#17430,0.173205080756888);
#1565=CIRCLE('',#17432,0.173205080756888);
#1566=CIRCLE('',#17434,0.173205080756888);
#1567=CIRCLE('',#17436,0.173205080756888);
#1568=CIRCLE('',#17438,0.173205080756888);
#1569=CIRCLE('',#17440,0.173205080756888);
#1570=CIRCLE('',#17442,0.171554298747513);
#1571=CIRCLE('',#17443,0.171554298747513);
#1572=CIRCLE('',#17444,0.171554298747513);
#1573=CIRCLE('',#17445,0.171554298747513);
#1574=CIRCLE('',#17446,0.171554298747513);
#1575=CIRCLE('',#17447,0.171554298747513);
#1576=CIRCLE('',#17448,0.171554298747513);
#1577=CIRCLE('',#17546,0.35);
#1578=CIRCLE('',#17548,0.35);
#1579=CIRCLE('',#17550,0.35);
#1580=CIRCLE('',#17552,0.35);
#1581=CIRCLE('',#17554,0.35);
#1582=CIRCLE('',#17556,0.35);
#1583=CIRCLE('',#17558,0.35);
#1584=CIRCLE('',#17560,0.35);
#1585=CIRCLE('',#17562,0.35);
#1586=CIRCLE('',#17564,0.35);
#1587=CIRCLE('',#17566,0.35);
#1588=CIRCLE('',#17568,0.35);
#1589=CIRCLE('',#17570,0.35);
#1590=CIRCLE('',#17572,0.35);
#1591=CIRCLE('',#17574,0.35);
#1592=CIRCLE('',#17576,0.35);
#1593=CIRCLE('',#17578,0.35);
#1594=CIRCLE('',#17580,0.35);
#1595=CIRCLE('',#17582,0.35);
#1596=CIRCLE('',#17584,0.35);
#1597=CIRCLE('',#17586,0.35);
#1598=CIRCLE('',#17588,0.35);
#1599=CIRCLE('',#17590,0.35);
#1600=CIRCLE('',#17592,0.35);
#1601=CIRCLE('',#17594,0.35);
#1602=CIRCLE('',#17596,0.35);
#1603=CIRCLE('',#17598,0.35);
#1604=CIRCLE('',#17600,0.35);
#1605=CIRCLE('',#17602,0.35);
#1606=CIRCLE('',#17604,0.35);
#1607=CIRCLE('',#17606,0.35);
#1608=CIRCLE('',#17608,0.35);
#1609=CIRCLE('',#17610,0.35);
#1610=CIRCLE('',#17612,0.35);
#1611=CIRCLE('',#17614,0.35);
#1612=CIRCLE('',#17616,0.35);
#1613=CIRCLE('',#17618,0.16);
#1614=CIRCLE('',#17621,0.31);
#1768=CONICAL_SURFACE('',#17441,0.0866025403784439,1.02614241494116);
#1769=CONICAL_SURFACE('',#17619,0.18,0.785398163397448);
#1770=CONICAL_SURFACE('',#17620,0.33,0.785398163397448);
#2391=FACE_OUTER_BOUND('',#3351,.T.);
#2392=FACE_OUTER_BOUND('',#3352,.T.);
#2393=FACE_OUTER_BOUND('',#3353,.T.);
#2394=FACE_OUTER_BOUND('',#3354,.T.);
#2395=FACE_OUTER_BOUND('',#3355,.T.);
#2396=FACE_OUTER_BOUND('',#3356,.T.);
#2397=FACE_OUTER_BOUND('',#3357,.T.);
#2398=FACE_OUTER_BOUND('',#3358,.T.);
#2399=FACE_OUTER_BOUND('',#3359,.T.);
#2400=FACE_OUTER_BOUND('',#3360,.T.);
#2401=FACE_OUTER_BOUND('',#3361,.T.);
#2402=FACE_OUTER_BOUND('',#3362,.T.);
#2403=FACE_OUTER_BOUND('',#3363,.T.);
#2404=FACE_OUTER_BOUND('',#3364,.T.);
#2405=FACE_OUTER_BOUND('',#3365,.T.);
#2406=FACE_OUTER_BOUND('',#3366,.T.);
#2407=FACE_OUTER_BOUND('',#3367,.T.);
#2408=FACE_OUTER_BOUND('',#3368,.T.);
#2409=FACE_OUTER_BOUND('',#3369,.T.);
#2410=FACE_OUTER_BOUND('',#3370,.T.);
#2411=FACE_OUTER_BOUND('',#3371,.T.);
#2412=FACE_OUTER_BOUND('',#3372,.T.);
#2413=FACE_OUTER_BOUND('',#3373,.T.);
#2414=FACE_OUTER_BOUND('',#3374,.T.);
#2415=FACE_OUTER_BOUND('',#3375,.T.);
#2416=FACE_OUTER_BOUND('',#3376,.T.);
#2417=FACE_OUTER_BOUND('',#3377,.T.);
#2418=FACE_OUTER_BOUND('',#3378,.T.);
#2419=FACE_OUTER_BOUND('',#3379,.T.);
#2420=FACE_OUTER_BOUND('',#3380,.T.);
#2421=FACE_OUTER_BOUND('',#3381,.T.);
#2422=FACE_OUTER_BOUND('',#3382,.T.);
#2423=FACE_OUTER_BOUND('',#3383,.T.);
#2424=FACE_OUTER_BOUND('',#3384,.T.);
#2425=FACE_OUTER_BOUND('',#3385,.T.);
#2426=FACE_OUTER_BOUND('',#3386,.T.);
#2427=FACE_OUTER_BOUND('',#3387,.T.);
#2428=FACE_OUTER_BOUND('',#3388,.T.);
#2429=FACE_OUTER_BOUND('',#3389,.T.);
#2430=FACE_OUTER_BOUND('',#3390,.T.);
#2431=FACE_OUTER_BOUND('',#3391,.T.);
#2432=FACE_OUTER_BOUND('',#3392,.T.);
#2433=FACE_OUTER_BOUND('',#3393,.T.);
#2434=FACE_OUTER_BOUND('',#3394,.T.);
#2435=FACE_OUTER_BOUND('',#3395,.T.);
#2436=FACE_OUTER_BOUND('',#3396,.T.);
#2437=FACE_OUTER_BOUND('',#3397,.T.);
#2438=FACE_OUTER_BOUND('',#3398,.T.);
#2439=FACE_OUTER_BOUND('',#3399,.T.);
#2440=FACE_OUTER_BOUND('',#3400,.T.);
#2441=FACE_OUTER_BOUND('',#3401,.T.);
#2442=FACE_OUTER_BOUND('',#3402,.T.);
#2443=FACE_OUTER_BOUND('',#3404,.T.);
#2444=FACE_OUTER_BOUND('',#3405,.T.);
#2445=FACE_OUTER_BOUND('',#3406,.T.);
#2446=FACE_OUTER_BOUND('',#3407,.T.);
#2447=FACE_OUTER_BOUND('',#3408,.T.);
#2448=FACE_OUTER_BOUND('',#3409,.T.);
#2449=FACE_OUTER_BOUND('',#3410,.T.);
#2450=FACE_OUTER_BOUND('',#3411,.T.);
#2451=FACE_OUTER_BOUND('',#3412,.T.);
#2452=FACE_OUTER_BOUND('',#3413,.T.);
#2453=FACE_OUTER_BOUND('',#3414,.T.);
#2454=FACE_OUTER_BOUND('',#3415,.T.);
#2455=FACE_OUTER_BOUND('',#3416,.T.);
#2456=FACE_OUTER_BOUND('',#3417,.T.);
#2457=FACE_OUTER_BOUND('',#3418,.T.);
#2458=FACE_OUTER_BOUND('',#3419,.T.);
#2459=FACE_OUTER_BOUND('',#3420,.T.);
#2460=FACE_OUTER_BOUND('',#3421,.T.);
#2461=FACE_OUTER_BOUND('',#3422,.T.);
#2462=FACE_OUTER_BOUND('',#3423,.T.);
#2463=FACE_OUTER_BOUND('',#3424,.T.);
#2464=FACE_OUTER_BOUND('',#3425,.T.);
#2465=FACE_OUTER_BOUND('',#3426,.T.);
#2466=FACE_OUTER_BOUND('',#3427,.T.);
#2467=FACE_OUTER_BOUND('',#3428,.T.);
#2468=FACE_OUTER_BOUND('',#3429,.T.);
#2469=FACE_OUTER_BOUND('',#3430,.T.);
#2470=FACE_OUTER_BOUND('',#3431,.T.);
#2471=FACE_OUTER_BOUND('',#3432,.T.);
#2472=FACE_OUTER_BOUND('',#3433,.T.);
#2473=FACE_OUTER_BOUND('',#3434,.T.);
#2474=FACE_OUTER_BOUND('',#3435,.T.);
#2475=FACE_OUTER_BOUND('',#3436,.T.);
#2476=FACE_OUTER_BOUND('',#3437,.T.);
#2477=FACE_OUTER_BOUND('',#3438,.T.);
#2478=FACE_OUTER_BOUND('',#3439,.T.);
#2479=FACE_OUTER_BOUND('',#3440,.T.);
#2480=FACE_OUTER_BOUND('',#3441,.T.);
#2481=FACE_OUTER_BOUND('',#3442,.T.);
#2482=FACE_OUTER_BOUND('',#3443,.T.);
#2483=FACE_OUTER_BOUND('',#3444,.T.);
#2484=FACE_OUTER_BOUND('',#3445,.T.);
#2485=FACE_OUTER_BOUND('',#3446,.T.);
#2486=FACE_OUTER_BOUND('',#3447,.T.);
#2487=FACE_OUTER_BOUND('',#3448,.T.);
#2488=FACE_OUTER_BOUND('',#3449,.T.);
#2489=FACE_OUTER_BOUND('',#3450,.T.);
#2490=FACE_OUTER_BOUND('',#3451,.T.);
#2491=FACE_OUTER_BOUND('',#3452,.T.);
#2492=FACE_OUTER_BOUND('',#3453,.T.);
#2493=FACE_OUTER_BOUND('',#3454,.T.);
#2494=FACE_OUTER_BOUND('',#3455,.T.);
#2495=FACE_OUTER_BOUND('',#3456,.T.);
#2496=FACE_OUTER_BOUND('',#3457,.T.);
#2497=FACE_OUTER_BOUND('',#3458,.T.);
#2498=FACE_OUTER_BOUND('',#3459,.T.);
#2499=FACE_OUTER_BOUND('',#3460,.T.);
#2500=FACE_OUTER_BOUND('',#3461,.T.);
#2501=FACE_OUTER_BOUND('',#3462,.T.);
#2502=FACE_OUTER_BOUND('',#3463,.T.);
#2503=FACE_OUTER_BOUND('',#3464,.T.);
#2504=FACE_OUTER_BOUND('',#3465,.T.);
#2505=FACE_OUTER_BOUND('',#3466,.T.);
#2506=FACE_OUTER_BOUND('',#3467,.T.);
#2507=FACE_OUTER_BOUND('',#3468,.T.);
#2508=FACE_OUTER_BOUND('',#3469,.T.);
#2509=FACE_OUTER_BOUND('',#3470,.T.);
#2510=FACE_OUTER_BOUND('',#3471,.T.);
#2511=FACE_OUTER_BOUND('',#3472,.T.);
#2512=FACE_OUTER_BOUND('',#3473,.T.);
#2513=FACE_OUTER_BOUND('',#3474,.T.);
#2514=FACE_OUTER_BOUND('',#3475,.T.);
#2515=FACE_OUTER_BOUND('',#3476,.T.);
#2516=FACE_OUTER_BOUND('',#3477,.T.);
#2517=FACE_OUTER_BOUND('',#3478,.T.);
#2518=FACE_OUTER_BOUND('',#3479,.T.);
#2519=FACE_OUTER_BOUND('',#3480,.T.);
#2520=FACE_OUTER_BOUND('',#3481,.T.);
#2521=FACE_OUTER_BOUND('',#3482,.T.);
#2522=FACE_OUTER_BOUND('',#3483,.T.);
#2523=FACE_OUTER_BOUND('',#3484,.T.);
#2524=FACE_OUTER_BOUND('',#3485,.T.);
#2525=FACE_OUTER_BOUND('',#3486,.T.);
#2526=FACE_OUTER_BOUND('',#3487,.T.);
#2527=FACE_OUTER_BOUND('',#3488,.T.);
#2528=FACE_OUTER_BOUND('',#3489,.T.);
#2529=FACE_OUTER_BOUND('',#3490,.T.);
#2530=FACE_OUTER_BOUND('',#3491,.T.);
#2531=FACE_OUTER_BOUND('',#3492,.T.);
#2532=FACE_OUTER_BOUND('',#3493,.T.);
#2533=FACE_OUTER_BOUND('',#3494,.T.);
#2534=FACE_OUTER_BOUND('',#3495,.T.);
#2535=FACE_OUTER_BOUND('',#3496,.T.);
#2536=FACE_OUTER_BOUND('',#3497,.T.);
#2537=FACE_OUTER_BOUND('',#3498,.T.);
#2538=FACE_OUTER_BOUND('',#3499,.T.);
#2539=FACE_OUTER_BOUND('',#3500,.T.);
#2540=FACE_OUTER_BOUND('',#3501,.T.);
#2541=FACE_OUTER_BOUND('',#3502,.T.);
#2542=FACE_OUTER_BOUND('',#3503,.T.);
#2543=FACE_OUTER_BOUND('',#3504,.T.);
#2544=FACE_OUTER_BOUND('',#3505,.T.);
#2545=FACE_OUTER_BOUND('',#3506,.T.);
#2546=FACE_OUTER_BOUND('',#3507,.T.);
#2547=FACE_OUTER_BOUND('',#3508,.T.);
#2548=FACE_OUTER_BOUND('',#3509,.T.);
#2549=FACE_OUTER_BOUND('',#3510,.T.);
#2550=FACE_OUTER_BOUND('',#3511,.T.);
#2551=FACE_OUTER_BOUND('',#3512,.T.);
#2552=FACE_OUTER_BOUND('',#3513,.T.);
#2553=FACE_OUTER_BOUND('',#3514,.T.);
#2554=FACE_OUTER_BOUND('',#3515,.T.);
#2555=FACE_OUTER_BOUND('',#3516,.T.);
#2556=FACE_OUTER_BOUND('',#3517,.T.);
#2557=FACE_OUTER_BOUND('',#3518,.T.);
#2558=FACE_OUTER_BOUND('',#3519,.T.);
#2559=FACE_OUTER_BOUND('',#3520,.T.);
#2560=FACE_OUTER_BOUND('',#3521,.T.);
#2561=FACE_OUTER_BOUND('',#3522,.T.);
#2562=FACE_OUTER_BOUND('',#3523,.T.);
#2563=FACE_OUTER_BOUND('',#3524,.T.);
#2564=FACE_OUTER_BOUND('',#3525,.T.);
#2565=FACE_OUTER_BOUND('',#3526,.T.);
#2566=FACE_OUTER_BOUND('',#3527,.T.);
#2567=FACE_OUTER_BOUND('',#3528,.T.);
#2568=FACE_OUTER_BOUND('',#3529,.T.);
#2569=FACE_OUTER_BOUND('',#3530,.T.);
#2570=FACE_OUTER_BOUND('',#3531,.T.);
#2571=FACE_OUTER_BOUND('',#3532,.T.);
#2572=FACE_OUTER_BOUND('',#3533,.T.);
#2573=FACE_OUTER_BOUND('',#3534,.T.);
#2574=FACE_OUTER_BOUND('',#3535,.T.);
#2575=FACE_OUTER_BOUND('',#3536,.T.);
#2576=FACE_OUTER_BOUND('',#3537,.T.);
#2577=FACE_OUTER_BOUND('',#3538,.T.);
#2578=FACE_OUTER_BOUND('',#3539,.T.);
#2579=FACE_OUTER_BOUND('',#3540,.T.);
#2580=FACE_OUTER_BOUND('',#3541,.T.);
#2581=FACE_OUTER_BOUND('',#3542,.T.);
#2582=FACE_OUTER_BOUND('',#3543,.T.);
#2583=FACE_OUTER_BOUND('',#3544,.T.);
#2584=FACE_OUTER_BOUND('',#3545,.T.);
#2585=FACE_OUTER_BOUND('',#3546,.T.);
#3351=EDGE_LOOP('',(#13123,#13124,#13125,#13126));
#3352=EDGE_LOOP('',(#13127,#13128,#13129,#13130));
#3353=EDGE_LOOP('',(#13131,#13132,#13133,#13134));
#3354=EDGE_LOOP('',(#13135,#13136,#13137,#13138));
#3355=EDGE_LOOP('',(#13139,#13140,#13141,#13142));
#3356=EDGE_LOOP('',(#13143,#13144,#13145,#13146));
#3357=EDGE_LOOP('',(#13147,#13148,#13149,#13150));
#3358=EDGE_LOOP('',(#13151,#13152,#13153,#13154));
#3359=EDGE_LOOP('',(#13155,#13156,#13157,#13158));
#3360=EDGE_LOOP('',(#13159,#13160,#13161,#13162));
#3361=EDGE_LOOP('',(#13163,#13164,#13165,#13166));
#3362=EDGE_LOOP('',(#13167,#13168,#13169,#13170));
#3363=EDGE_LOOP('',(#13171,#13172,#13173,#13174));
#3364=EDGE_LOOP('',(#13175,#13176,#13177,#13178));
#3365=EDGE_LOOP('',(#13179,#13180,#13181,#13182));
#3366=EDGE_LOOP('',(#13183,#13184,#13185,#13186));
#3367=EDGE_LOOP('',(#13187,#13188,#13189,#13190));
#3368=EDGE_LOOP('',(#13191,#13192,#13193,#13194));
#3369=EDGE_LOOP('',(#13195,#13196,#13197,#13198));
#3370=EDGE_LOOP('',(#13199,#13200,#13201,#13202));
#3371=EDGE_LOOP('',(#13203,#13204,#13205,#13206));
#3372=EDGE_LOOP('',(#13207,#13208,#13209,#13210));
#3373=EDGE_LOOP('',(#13211,#13212,#13213,#13214));
#3374=EDGE_LOOP('',(#13215,#13216,#13217,#13218));
#3375=EDGE_LOOP('',(#13219,#13220,#13221,#13222));
#3376=EDGE_LOOP('',(#13223,#13224,#13225,#13226));
#3377=EDGE_LOOP('',(#13227,#13228,#13229,#13230));
#3378=EDGE_LOOP('',(#13231,#13232,#13233,#13234));
#3379=EDGE_LOOP('',(#13235,#13236,#13237,#13238));
#3380=EDGE_LOOP('',(#13239,#13240,#13241,#13242));
#3381=EDGE_LOOP('',(#13243,#13244,#13245,#13246));
#3382=EDGE_LOOP('',(#13247,#13248,#13249,#13250));
#3383=EDGE_LOOP('',(#13251,#13252,#13253,#13254));
#3384=EDGE_LOOP('',(#13255,#13256,#13257,#13258));
#3385=EDGE_LOOP('',(#13259,#13260,#13261,#13262));
#3386=EDGE_LOOP('',(#13263,#13264,#13265,#13266));
#3387=EDGE_LOOP('',(#13267,#13268,#13269,#13270));
#3388=EDGE_LOOP('',(#13271,#13272,#13273,#13274));
#3389=EDGE_LOOP('',(#13275,#13276,#13277,#13278));
#3390=EDGE_LOOP('',(#13279,#13280,#13281,#13282));
#3391=EDGE_LOOP('',(#13283,#13284,#13285,#13286));
#3392=EDGE_LOOP('',(#13287,#13288,#13289,#13290));
#3393=EDGE_LOOP('',(#13291,#13292,#13293,#13294));
#3394=EDGE_LOOP('',(#13295,#13296,#13297,#13298));
#3395=EDGE_LOOP('',(#13299,#13300,#13301,#13302,#13303));
#3396=EDGE_LOOP('',(#13304,#13305,#13306,#13307,#13308,#13309,#13310,#13311,
#13312,#13313,#13314,#13315,#13316,#13317,#13318,#13319,#13320,#13321,#13322,
#13323,#13324,#13325,#13326,#13327,#13328,#13329,#13330,#13331,#13332,#13333,
#13334,#13335,#13336,#13337,#13338,#13339,#13340,#13341,#13342,#13343,#13344,
#13345,#13346,#13347,#13348,#13349,#13350,#13351));
#3397=EDGE_LOOP('',(#13352,#13353,#13354,#13355,#13356));
#3398=EDGE_LOOP('',(#13357,#13358,#13359,#13360));
#3399=EDGE_LOOP('',(#13361,#13362,#13363,#13364,#13365,#13366,#13367,#13368,
#13369,#13370,#13371,#13372,#13373,#13374,#13375,#13376,#13377,#13378,#13379,
#13380,#13381,#13382,#13383,#13384,#13385,#13386,#13387,#13388,#13389,#13390,
#13391,#13392,#13393,#13394,#13395,#13396,#13397,#13398,#13399,#13400,#13401,
#13402,#13403,#13404,#13405,#13406,#13407,#13408));
#3400=EDGE_LOOP('',(#13409,#13410,#13411,#13412,#13413,#13414));
#3401=EDGE_LOOP('',(#13415,#13416,#13417,#13418));
#3402=EDGE_LOOP('',(#13419,#13420,#13421,#13422,#13423,#13424,#13425,#13426,
#13427,#13428,#13429,#13430,#13431,#13432,#13433,#13434,#13435,#13436,#13437,
#13438,#13439,#13440,#13441,#13442,#13443,#13444,#13445,#13446,#13447,#13448,
#13449,#13450,#13451,#13452,#13453,#13454,#13455,#13456,#13457,#13458,#13459,
#13460,#13461,#13462,#13463,#13464,#13465,#13466,#13467,#13468,#13469,#13470,
#13471,#13472,#13473,#13474,#13475,#13476,#13477,#13478,#13479,#13480,#13481,
#13482,#13483,#13484,#13485,#13486,#13487,#13488,#13489,#13490,#13491,#13492,
#13493,#13494,#13495,#13496,#13497,#13498,#13499,#13500,#13501,#13502,#13503,
#13504,#13505,#13506,#13507,#13508,#13509,#13510,#13511,#13512,#13513,#13514,
#13515,#13516,#13517,#13518,#13519,#13520,#13521,#13522,#13523,#13524,#13525,
#13526));
#3403=EDGE_LOOP('',(#13527));
#3404=EDGE_LOOP('',(#13528,#13529));
#3405=EDGE_LOOP('',(#13530,#13531));
#3406=EDGE_LOOP('',(#13532,#13533));
#3407=EDGE_LOOP('',(#13534,#13535));
#3408=EDGE_LOOP('',(#13536,#13537));
#3409=EDGE_LOOP('',(#13538,#13539));
#3410=EDGE_LOOP('',(#13540,#13541,#13542,#13543,#13544,#13545,#13546,#13547,
#13548,#13549,#13550,#13551,#13552,#13553,#13554,#13555,#13556,#13557,#13558,
#13559,#13560,#13561,#13562,#13563,#13564,#13565,#13566));
#3411=EDGE_LOOP('',(#13567,#13568,#13569,#13570));
#3412=EDGE_LOOP('',(#13571,#13572,#13573));
#3413=EDGE_LOOP('',(#13574,#13575,#13576,#13577));
#3414=EDGE_LOOP('',(#13578,#13579,#13580));
#3415=EDGE_LOOP('',(#13581,#13582,#13583));
#3416=EDGE_LOOP('',(#13584,#13585,#13586,#13587));
#3417=EDGE_LOOP('',(#13588,#13589,#13590));
#3418=EDGE_LOOP('',(#13591,#13592,#13593,#13594));
#3419=EDGE_LOOP('',(#13595,#13596,#13597));
#3420=EDGE_LOOP('',(#13598,#13599,#13600));
#3421=EDGE_LOOP('',(#13601,#13602,#13603));
#3422=EDGE_LOOP('',(#13604,#13605,#13606));
#3423=EDGE_LOOP('',(#13607,#13608,#13609));
#3424=EDGE_LOOP('',(#13610,#13611,#13612));
#3425=EDGE_LOOP('',(#13613,#13614,#13615));
#3426=EDGE_LOOP('',(#13616,#13617,#13618,#13619));
#3427=EDGE_LOOP('',(#13620,#13621,#13622,#13623));
#3428=EDGE_LOOP('',(#13624,#13625,#13626));
#3429=EDGE_LOOP('',(#13627,#13628,#13629));
#3430=EDGE_LOOP('',(#13630,#13631,#13632));
#3431=EDGE_LOOP('',(#13633,#13634,#13635,#13636));
#3432=EDGE_LOOP('',(#13637,#13638,#13639));
#3433=EDGE_LOOP('',(#13640,#13641,#13642));
#3434=EDGE_LOOP('',(#13643,#13644,#13645));
#3435=EDGE_LOOP('',(#13646,#13647,#13648,#13649));
#3436=EDGE_LOOP('',(#13650,#13651,#13652,#13653));
#3437=EDGE_LOOP('',(#13654,#13655,#13656,#13657));
#3438=EDGE_LOOP('',(#13658,#13659,#13660,#13661));
#3439=EDGE_LOOP('',(#13662,#13663,#13664,#13665));
#3440=EDGE_LOOP('',(#13666,#13667,#13668,#13669));
#3441=EDGE_LOOP('',(#13670,#13671,#13672,#13673));
#3442=EDGE_LOOP('',(#13674,#13675,#13676,#13677));
#3443=EDGE_LOOP('',(#13678,#13679,#13680,#13681));
#3444=EDGE_LOOP('',(#13682,#13683,#13684,#13685));
#3445=EDGE_LOOP('',(#13686,#13687,#13688,#13689));
#3446=EDGE_LOOP('',(#13690,#13691,#13692,#13693));
#3447=EDGE_LOOP('',(#13694,#13695,#13696,#13697));
#3448=EDGE_LOOP('',(#13698,#13699,#13700,#13701));
#3449=EDGE_LOOP('',(#13702,#13703,#13704,#13705));
#3450=EDGE_LOOP('',(#13706,#13707,#13708,#13709));
#3451=EDGE_LOOP('',(#13710,#13711,#13712,#13713));
#3452=EDGE_LOOP('',(#13714,#13715,#13716,#13717));
#3453=EDGE_LOOP('',(#13718,#13719,#13720,#13721));
#3454=EDGE_LOOP('',(#13722,#13723,#13724,#13725));
#3455=EDGE_LOOP('',(#13726,#13727,#13728,#13729));
#3456=EDGE_LOOP('',(#13730,#13731,#13732,#13733));
#3457=EDGE_LOOP('',(#13734,#13735,#13736,#13737));
#3458=EDGE_LOOP('',(#13738,#13739,#13740,#13741));
#3459=EDGE_LOOP('',(#13742,#13743,#13744,#13745));
#3460=EDGE_LOOP('',(#13746,#13747,#13748,#13749));
#3461=EDGE_LOOP('',(#13750,#13751,#13752,#13753));
#3462=EDGE_LOOP('',(#13754,#13755,#13756,#13757));
#3463=EDGE_LOOP('',(#13758,#13759,#13760,#13761));
#3464=EDGE_LOOP('',(#13762,#13763,#13764,#13765));
#3465=EDGE_LOOP('',(#13766,#13767,#13768,#13769));
#3466=EDGE_LOOP('',(#13770,#13771,#13772,#13773));
#3467=EDGE_LOOP('',(#13774,#13775,#13776,#13777));
#3468=EDGE_LOOP('',(#13778,#13779,#13780,#13781));
#3469=EDGE_LOOP('',(#13782,#13783,#13784,#13785));
#3470=EDGE_LOOP('',(#13786,#13787,#13788,#13789));
#3471=EDGE_LOOP('',(#13790,#13791,#13792,#13793));
#3472=EDGE_LOOP('',(#13794,#13795,#13796,#13797));
#3473=EDGE_LOOP('',(#13798,#13799,#13800,#13801));
#3474=EDGE_LOOP('',(#13802,#13803,#13804,#13805));
#3475=EDGE_LOOP('',(#13806,#13807,#13808,#13809));
#3476=EDGE_LOOP('',(#13810,#13811,#13812,#13813));
#3477=EDGE_LOOP('',(#13814,#13815,#13816,#13817));
#3478=EDGE_LOOP('',(#13818,#13819,#13820,#13821));
#3479=EDGE_LOOP('',(#13822,#13823,#13824,#13825));
#3480=EDGE_LOOP('',(#13826,#13827,#13828,#13829));
#3481=EDGE_LOOP('',(#13830,#13831,#13832,#13833));
#3482=EDGE_LOOP('',(#13834,#13835,#13836,#13837));
#3483=EDGE_LOOP('',(#13838,#13839,#13840,#13841));
#3484=EDGE_LOOP('',(#13842,#13843,#13844,#13845));
#3485=EDGE_LOOP('',(#13846,#13847,#13848,#13849));
#3486=EDGE_LOOP('',(#13850,#13851,#13852,#13853));
#3487=EDGE_LOOP('',(#13854,#13855,#13856,#13857));
#3488=EDGE_LOOP('',(#13858,#13859,#13860,#13861));
#3489=EDGE_LOOP('',(#13862,#13863,#13864,#13865));
#3490=EDGE_LOOP('',(#13866,#13867,#13868,#13869));
#3491=EDGE_LOOP('',(#13870,#13871,#13872,#13873));
#3492=EDGE_LOOP('',(#13874,#13875,#13876,#13877));
#3493=EDGE_LOOP('',(#13878,#13879,#13880,#13881));
#3494=EDGE_LOOP('',(#13882,#13883,#13884,#13885));
#3495=EDGE_LOOP('',(#13886,#13887,#13888,#13889));
#3496=EDGE_LOOP('',(#13890,#13891,#13892,#13893));
#3497=EDGE_LOOP('',(#13894,#13895,#13896,#13897));
#3498=EDGE_LOOP('',(#13898,#13899,#13900,#13901));
#3499=EDGE_LOOP('',(#13902,#13903,#13904,#13905));
#3500=EDGE_LOOP('',(#13906,#13907,#13908,#13909));
#3501=EDGE_LOOP('',(#13910,#13911,#13912,#13913));
#3502=EDGE_LOOP('',(#13914,#13915,#13916,#13917));
#3503=EDGE_LOOP('',(#13918,#13919,#13920,#13921));
#3504=EDGE_LOOP('',(#13922,#13923,#13924,#13925));
#3505=EDGE_LOOP('',(#13926,#13927,#13928,#13929));
#3506=EDGE_LOOP('',(#13930,#13931,#13932,#13933));
#3507=EDGE_LOOP('',(#13934,#13935,#13936,#13937));
#3508=EDGE_LOOP('',(#13938,#13939,#13940,#13941));
#3509=EDGE_LOOP('',(#13942,#13943,#13944,#13945));
#3510=EDGE_LOOP('',(#13946,#13947,#13948,#13949));
#3511=EDGE_LOOP('',(#13950,#13951,#13952,#13953));
#3512=EDGE_LOOP('',(#13954,#13955,#13956,#13957));
#3513=EDGE_LOOP('',(#13958,#13959,#13960,#13961));
#3514=EDGE_LOOP('',(#13962,#13963,#13964,#13965));
#3515=EDGE_LOOP('',(#13966,#13967,#13968,#13969));
#3516=EDGE_LOOP('',(#13970,#13971,#13972,#13973));
#3517=EDGE_LOOP('',(#13974,#13975,#13976,#13977));
#3518=EDGE_LOOP('',(#13978,#13979,#13980,#13981));
#3519=EDGE_LOOP('',(#13982,#13983,#13984,#13985));
#3520=EDGE_LOOP('',(#13986,#13987,#13988,#13989));
#3521=EDGE_LOOP('',(#13990,#13991,#13992,#13993));
#3522=EDGE_LOOP('',(#13994,#13995,#13996,#13997));
#3523=EDGE_LOOP('',(#13998,#13999,#14000,#14001));
#3524=EDGE_LOOP('',(#14002,#14003,#14004,#14005));
#3525=EDGE_LOOP('',(#14006,#14007,#14008,#14009));
#3526=EDGE_LOOP('',(#14010,#14011,#14012,#14013));
#3527=EDGE_LOOP('',(#14014,#14015,#14016,#14017));
#3528=EDGE_LOOP('',(#14018,#14019,#14020,#14021));
#3529=EDGE_LOOP('',(#14022,#14023,#14024,#14025));
#3530=EDGE_LOOP('',(#14026,#14027,#14028,#14029));
#3531=EDGE_LOOP('',(#14030,#14031,#14032,#14033));
#3532=EDGE_LOOP('',(#14034,#14035,#14036,#14037));
#3533=EDGE_LOOP('',(#14038,#14039,#14040,#14041));
#3534=EDGE_LOOP('',(#14042,#14043,#14044,#14045));
#3535=EDGE_LOOP('',(#14046,#14047,#14048,#14049));
#3536=EDGE_LOOP('',(#14050,#14051,#14052,#14053));
#3537=EDGE_LOOP('',(#14054,#14055,#14056,#14057));
#3538=EDGE_LOOP('',(#14058,#14059,#14060,#14061));
#3539=EDGE_LOOP('',(#14062,#14063,#14064,#14065));
#3540=EDGE_LOOP('',(#14066,#14067,#14068,#14069));
#3541=EDGE_LOOP('',(#14070,#14071,#14072,#14073));
#3542=EDGE_LOOP('',(#14074,#14075,#14076,#14077));
#3543=EDGE_LOOP('',(#14078));
#3544=EDGE_LOOP('',(#14079,#14080,#14081,#14082,#14083,#14084));
#3545=EDGE_LOOP('',(#14085,#14086,#14087,#14088,#14089,#14090,#14091,#14092,
#14093,#14094,#14095,#14096,#14097,#14098,#14099,#14100,#14101,#14102,#14103,
#14104,#14105,#14106,#14107,#14108,#14109,#14110,#14111,#14112,#14113,#14114,
#14115,#14116,#14117,#14118,#14119,#14120,#14121,#14122,#14123,#14124,#14125,
#14126,#14127,#14128,#14129,#14130,#14131,#14132,#14133,#14134,#14135,#14136,
#14137,#14138,#14139,#14140,#14141,#14142,#14143,#14144,#14145,#14146,#14147,
#14148,#14149,#14150,#14151,#14152,#14153,#14154,#14155,#14156,#14157,#14158,
#14159,#14160,#14161,#14162,#14163,#14164,#14165,#14166,#14167,#14168,#14169,
#14170,#14171,#14172,#14173,#14174,#14175,#14176,#14177,#14178,#14179,#14180,
#14181,#14182,#14183,#14184,#14185,#14186,#14187,#14188,#14189,#14190,#14191,
#14192,#14193,#14194,#14195));
#3546=EDGE_LOOP('',(#14196));
#3547=EDGE_LOOP('',(#14197,#14198,#14199,#14200,#14201,#14202));
#4518=LINE('',#32272,#5742);
#4519=LINE('',#32296,#5743);
#4520=LINE('',#32344,#5744);
#4521=LINE('',#32392,#5745);
#4522=LINE('',#32443,#5746);
#4523=LINE('',#32494,#5747);
#4524=LINE('',#32542,#5748);
#4525=LINE('',#32590,#5749);
#4526=LINE('',#32644,#5750);
#4527=LINE('',#32692,#5751);
#4528=LINE('',#32740,#5752);
#4529=LINE('',#32794,#5753);
#4530=LINE('',#32842,#5754);
#4531=LINE('',#32890,#5755);
#4532=LINE('',#32938,#5756);
#4533=LINE('',#32992,#5757);
#4534=LINE('',#33040,#5758);
#4535=LINE('',#33088,#5759);
#4536=LINE('',#33142,#5760);
#4537=LINE('',#33190,#5761);
#4538=LINE('',#33238,#5762);
#4539=LINE('',#33292,#5763);
#4540=LINE('',#33340,#5764);
#4541=LINE('',#33358,#5765);
#4542=LINE('',#33382,#5766);
#4543=LINE('',#33407,#5767);
#4544=LINE('',#33432,#5768);
#4545=LINE('',#33456,#5769);
#4546=LINE('',#33481,#5770);
#4547=LINE('',#33506,#5771);
#4548=LINE('',#33530,#5772);
#4549=LINE('',#33555,#5773);
#4550=LINE('',#33580,#5774);
#4551=LINE('',#33604,#5775);
#4552=LINE('',#33628,#5776);
#4553=LINE('',#33653,#5777);
#4554=LINE('',#33678,#5778);
#4555=LINE('',#33702,#5779);
#4556=LINE('',#33727,#5780);
#4557=LINE('',#33752,#5781);
#4558=LINE('',#33776,#5782);
#4559=LINE('',#33801,#5783);
#4560=LINE('',#33825,#5784);
#4561=LINE('',#33850,#5785);
#4562=LINE('',#35306,#5786);
#4563=LINE('',#35308,#5787);
#4564=LINE('',#35312,#5788);
#4565=LINE('',#35314,#5789);
#4566=LINE('',#35318,#5790);
#4567=LINE('',#35320,#5791);
#4568=LINE('',#35324,#5792);
#4569=LINE('',#35326,#5793);
#4570=LINE('',#35330,#5794);
#4571=LINE('',#35332,#5795);
#4572=LINE('',#35336,#5796);
#4573=LINE('',#35338,#5797);
#4574=LINE('',#35342,#5798);
#4575=LINE('',#35344,#5799);
#4576=LINE('',#35348,#5800);
#4577=LINE('',#35350,#5801);
#4578=LINE('',#35354,#5802);
#4579=LINE('',#35356,#5803);
#4580=LINE('',#35360,#5804);
#4581=LINE('',#35362,#5805);
#4582=LINE('',#35366,#5806);
#4583=LINE('',#35368,#5807);
#4584=LINE('',#35372,#5808);
#4585=LINE('',#35374,#5809);
#4586=LINE('',#35378,#5810);
#4587=LINE('',#35380,#5811);
#4588=LINE('',#35384,#5812);
#4589=LINE('',#35386,#5813);
#4590=LINE('',#35390,#5814);
#4591=LINE('',#35392,#5815);
#4592=LINE('',#35396,#5816);
#4593=LINE('',#35398,#5817);
#4594=LINE('',#35402,#5818);
#4595=LINE('',#35404,#5819);
#4596=LINE('',#35408,#5820);
#4597=LINE('',#35410,#5821);
#4598=LINE('',#35414,#5822);
#4599=LINE('',#35416,#5823);
#4600=LINE('',#35420,#5824);
#4601=LINE('',#35422,#5825);
#4602=LINE('',#35426,#5826);
#4603=LINE('',#35428,#5827);
#4604=LINE('',#35432,#5828);
#4605=LINE('',#35434,#5829);
#4606=LINE('',#35438,#5830);
#4607=LINE('',#35440,#5831);
#4608=LINE('',#35444,#5832);
#4609=LINE('',#35446,#5833);
#4610=LINE('',#35450,#5834);
#4611=LINE('',#35452,#5835);
#4612=LINE('',#35456,#5836);
#4613=LINE('',#35458,#5837);
#4614=LINE('',#35462,#5838);
#4615=LINE('',#35464,#5839);
#4616=LINE('',#35468,#5840);
#4617=LINE('',#35470,#5841);
#4618=LINE('',#35474,#5842);
#4619=LINE('',#35476,#5843);
#4620=LINE('',#35480,#5844);
#4621=LINE('',#35482,#5845);
#4622=LINE('',#35486,#5846);
#4623=LINE('',#35488,#5847);
#4624=LINE('',#35492,#5848);
#4625=LINE('',#35494,#5849);
#4626=LINE('',#35498,#5850);
#4627=LINE('',#35500,#5851);
#4628=LINE('',#35504,#5852);
#4629=LINE('',#35506,#5853);
#4630=LINE('',#35510,#5854);
#4631=LINE('',#35512,#5855);
#4632=LINE('',#35516,#5856);
#4633=LINE('',#35518,#5857);
#4634=LINE('',#35523,#5858);
#4635=LINE('',#35527,#5859);
#4636=LINE('',#35531,#5860);
#4637=LINE('',#35535,#5861);
#4638=LINE('',#35539,#5862);
#4639=LINE('',#35542,#5863);
#4640=LINE('',#35547,#5864);
#4641=LINE('',#35605,#5865);
#4642=LINE('',#35607,#5866);
#4643=LINE('',#35608,#5867);
#4644=LINE('',#35611,#5868);
#4645=LINE('',#35612,#5869);
#4646=LINE('',#35615,#5870);
#4647=LINE('',#35616,#5871);
#4648=LINE('',#35619,#5872);
#4649=LINE('',#35620,#5873);
#4650=LINE('',#35623,#5874);
#4651=LINE('',#35624,#5875);
#4652=LINE('',#35627,#5876);
#4653=LINE('',#35628,#5877);
#4654=LINE('',#35631,#5878);
#4655=LINE('',#35632,#5879);
#4656=LINE('',#35635,#5880);
#4657=LINE('',#35636,#5881);
#4658=LINE('',#35639,#5882);
#4659=LINE('',#35640,#5883);
#4660=LINE('',#35642,#5884);
#4661=LINE('',#35644,#5885);
#4662=LINE('',#35647,#5886);
#4663=LINE('',#35650,#5887);
#4664=LINE('',#35651,#5888);
#4665=LINE('',#35653,#5889);
#4666=LINE('',#35655,#5890);
#4667=LINE('',#35658,#5891);
#4668=LINE('',#35659,#5892);
#4669=LINE('',#35661,#5893);
#4670=LINE('',#35665,#5894);
#4671=LINE('',#35675,#5895);
#4672=LINE('',#35676,#5896);
#4673=LINE('',#35682,#5897);
#4674=LINE('',#35689,#5898);
#4675=LINE('',#35690,#5899);
#4676=LINE('',#35696,#5900);
#4677=LINE('',#35703,#5901);
#4678=LINE('',#35704,#5902);
#4679=LINE('',#35710,#5903);
#4680=LINE('',#35717,#5904);
#4681=LINE('',#35718,#5905);
#4682=LINE('',#35724,#5906);
#4683=LINE('',#35731,#5907);
#4684=LINE('',#35732,#5908);
#4685=LINE('',#35738,#5909);
#4686=LINE('',#35745,#5910);
#4687=LINE('',#35746,#5911);
#4688=LINE('',#35752,#5912);
#4689=LINE('',#35759,#5913);
#4690=LINE('',#35760,#5914);
#4691=LINE('',#35766,#5915);
#4692=LINE('',#35773,#5916);
#4693=LINE('',#35774,#5917);
#4694=LINE('',#35780,#5918);
#4695=LINE('',#35787,#5919);
#4696=LINE('',#35788,#5920);
#4697=LINE('',#35794,#5921);
#4698=LINE('',#35801,#5922);
#4699=LINE('',#35802,#5923);
#4700=LINE('',#35808,#5924);
#4701=LINE('',#35815,#5925);
#4702=LINE('',#35816,#5926);
#4703=LINE('',#35822,#5927);
#4704=LINE('',#35829,#5928);
#4705=LINE('',#35830,#5929);
#4706=LINE('',#35836,#5930);
#4707=LINE('',#35843,#5931);
#4708=LINE('',#35844,#5932);
#4709=LINE('',#35850,#5933);
#4710=LINE('',#35857,#5934);
#4711=LINE('',#35858,#5935);
#4712=LINE('',#35864,#5936);
#4713=LINE('',#35871,#5937);
#4714=LINE('',#35872,#5938);
#4715=LINE('',#35878,#5939);
#4716=LINE('',#35885,#5940);
#4717=LINE('',#35886,#5941);
#4718=LINE('',#35892,#5942);
#4719=LINE('',#35899,#5943);
#4720=LINE('',#35900,#5944);
#4721=LINE('',#35906,#5945);
#4722=LINE('',#35913,#5946);
#4723=LINE('',#35914,#5947);
#4724=LINE('',#35920,#5948);
#4725=LINE('',#35927,#5949);
#4726=LINE('',#35928,#5950);
#4727=LINE('',#35934,#5951);
#4728=LINE('',#35941,#5952);
#4729=LINE('',#35942,#5953);
#4730=LINE('',#35948,#5954);
#4731=LINE('',#35955,#5955);
#4732=LINE('',#35956,#5956);
#4733=LINE('',#35962,#5957);
#4734=LINE('',#35969,#5958);
#4735=LINE('',#35970,#5959);
#4736=LINE('',#35976,#5960);
#4737=LINE('',#35983,#5961);
#4738=LINE('',#35984,#5962);
#4739=LINE('',#35990,#5963);
#4740=LINE('',#35997,#5964);
#4741=LINE('',#35998,#5965);
#4742=LINE('',#36004,#5966);
#4743=LINE('',#36011,#5967);
#4744=LINE('',#36012,#5968);
#4745=LINE('',#36018,#5969);
#4746=LINE('',#36025,#5970);
#4747=LINE('',#36026,#5971);
#4748=LINE('',#36032,#5972);
#4749=LINE('',#36039,#5973);
#4750=LINE('',#36040,#5974);
#4751=LINE('',#36046,#5975);
#4752=LINE('',#36053,#5976);
#4753=LINE('',#36054,#5977);
#4754=LINE('',#36060,#5978);
#4755=LINE('',#36067,#5979);
#4756=LINE('',#36068,#5980);
#4757=LINE('',#36074,#5981);
#4758=LINE('',#36081,#5982);
#4759=LINE('',#36082,#5983);
#4760=LINE('',#36088,#5984);
#4761=LINE('',#36095,#5985);
#4762=LINE('',#36096,#5986);
#4763=LINE('',#36102,#5987);
#4764=LINE('',#36109,#5988);
#4765=LINE('',#36110,#5989);
#4766=LINE('',#36116,#5990);
#4767=LINE('',#36123,#5991);
#4768=LINE('',#36124,#5992);
#4769=LINE('',#36130,#5993);
#4770=LINE('',#36137,#5994);
#4771=LINE('',#36138,#5995);
#4772=LINE('',#36144,#5996);
#4773=LINE('',#36151,#5997);
#4774=LINE('',#36152,#5998);
#4775=LINE('',#36158,#5999);
#4776=LINE('',#36165,#6000);
#4777=LINE('',#36166,#6001);
#4778=LINE('',#36172,#6002);
#4779=LINE('',#36249,#6003);
#4780=LINE('',#36253,#6004);
#5742=VECTOR('',#20531,0.2);
#5743=VECTOR('',#20536,0.2);
#5744=VECTOR('',#20539,0.2);
#5745=VECTOR('',#20542,0.2);
#5746=VECTOR('',#20545,0.2);
#5747=VECTOR('',#20548,0.2);
#5748=VECTOR('',#20551,0.2);
#5749=VECTOR('',#20554,0.2);
#5750=VECTOR('',#20557,0.2);
#5751=VECTOR('',#20560,0.2);
#5752=VECTOR('',#20563,0.2);
#5753=VECTOR('',#20566,0.2);
#5754=VECTOR('',#20569,0.2);
#5755=VECTOR('',#20572,0.2);
#5756=VECTOR('',#20575,0.2);
#5757=VECTOR('',#20578,0.2);
#5758=VECTOR('',#20581,0.2);
#5759=VECTOR('',#20584,0.2);
#5760=VECTOR('',#20587,0.2);
#5761=VECTOR('',#20590,0.2);
#5762=VECTOR('',#20593,0.2);
#5763=VECTOR('',#20596,0.2);
#5764=VECTOR('',#20599,0.15555);
#5765=VECTOR('',#20604,0.15555);
#5766=VECTOR('',#20607,0.15555);
#5767=VECTOR('',#20610,0.15555);
#5768=VECTOR('',#20613,0.15555);
#5769=VECTOR('',#20616,0.15555);
#5770=VECTOR('',#20619,0.15555);
#5771=VECTOR('',#20622,0.15555);
#5772=VECTOR('',#20625,0.15555);
#5773=VECTOR('',#20628,0.15555);
#5774=VECTOR('',#20631,0.15555);
#5775=VECTOR('',#20634,0.15555);
#5776=VECTOR('',#20637,0.15555);
#5777=VECTOR('',#20640,0.15555);
#5778=VECTOR('',#20643,0.15555);
#5779=VECTOR('',#20646,0.15555);
#5780=VECTOR('',#20649,0.15555);
#5781=VECTOR('',#20652,0.15555);
#5782=VECTOR('',#20655,0.15555);
#5783=VECTOR('',#20658,0.15555);
#5784=VECTOR('',#20661,0.15555);
#5785=VECTOR('',#20664,0.15555);
#5786=VECTOR('',#20693,1.);
#5787=VECTOR('',#20694,1.);
#5788=VECTOR('',#20697,1.);
#5789=VECTOR('',#20698,1.);
#5790=VECTOR('',#20701,1.);
#5791=VECTOR('',#20702,1.);
#5792=VECTOR('',#20705,1.);
#5793=VECTOR('',#20706,1.);
#5794=VECTOR('',#20709,1.);
#5795=VECTOR('',#20710,1.);
#5796=VECTOR('',#20713,1.);
#5797=VECTOR('',#20714,1.);
#5798=VECTOR('',#20717,1.);
#5799=VECTOR('',#20718,1.);
#5800=VECTOR('',#20721,1.);
#5801=VECTOR('',#20722,1.);
#5802=VECTOR('',#20725,1.);
#5803=VECTOR('',#20726,1.);
#5804=VECTOR('',#20729,1.);
#5805=VECTOR('',#20730,1.);
#5806=VECTOR('',#20733,1.);
#5807=VECTOR('',#20734,1.);
#5808=VECTOR('',#20737,1.);
#5809=VECTOR('',#20738,1.);
#5810=VECTOR('',#20741,1.);
#5811=VECTOR('',#20742,1.);
#5812=VECTOR('',#20745,1.);
#5813=VECTOR('',#20746,1.);
#5814=VECTOR('',#20749,1.);
#5815=VECTOR('',#20750,1.);
#5816=VECTOR('',#20753,1.);
#5817=VECTOR('',#20754,1.);
#5818=VECTOR('',#20757,1.);
#5819=VECTOR('',#20758,1.);
#5820=VECTOR('',#20761,1.);
#5821=VECTOR('',#20762,1.);
#5822=VECTOR('',#20765,1.);
#5823=VECTOR('',#20766,1.);
#5824=VECTOR('',#20769,1.);
#5825=VECTOR('',#20770,1.);
#5826=VECTOR('',#20773,1.);
#5827=VECTOR('',#20774,1.);
#5828=VECTOR('',#20777,1.);
#5829=VECTOR('',#20778,1.);
#5830=VECTOR('',#20781,1.);
#5831=VECTOR('',#20782,1.);
#5832=VECTOR('',#20785,1.);
#5833=VECTOR('',#20786,1.);
#5834=VECTOR('',#20789,1.);
#5835=VECTOR('',#20790,1.);
#5836=VECTOR('',#20793,1.);
#5837=VECTOR('',#20794,1.);
#5838=VECTOR('',#20797,1.);
#5839=VECTOR('',#20798,1.);
#5840=VECTOR('',#20801,1.);
#5841=VECTOR('',#20802,1.);
#5842=VECTOR('',#20805,1.);
#5843=VECTOR('',#20806,1.);
#5844=VECTOR('',#20809,1.);
#5845=VECTOR('',#20810,1.);
#5846=VECTOR('',#20813,1.);
#5847=VECTOR('',#20814,1.);
#5848=VECTOR('',#20817,1.);
#5849=VECTOR('',#20818,1.);
#5850=VECTOR('',#20821,1.);
#5851=VECTOR('',#20822,1.);
#5852=VECTOR('',#20825,1.);
#5853=VECTOR('',#20826,1.);
#5854=VECTOR('',#20829,1.);
#5855=VECTOR('',#20830,1.);
#5856=VECTOR('',#20833,1.);
#5857=VECTOR('',#20834,1.);
#5858=VECTOR('',#20839,1.);
#5859=VECTOR('',#20844,1.);
#5860=VECTOR('',#20849,1.);
#5861=VECTOR('',#20854,1.);
#5862=VECTOR('',#20859,1.);
#5863=VECTOR('',#20864,1.);
#5864=VECTOR('',#20869,0.0866025403784439);
#5865=VECTOR('',#20886,1.);
#5866=VECTOR('',#20887,1.);
#5867=VECTOR('',#20888,1.);
#5868=VECTOR('',#20891,1.);
#5869=VECTOR('',#20892,1.);
#5870=VECTOR('',#20895,1.);
#5871=VECTOR('',#20896,1.);
#5872=VECTOR('',#20899,1.);
#5873=VECTOR('',#20900,1.);
#5874=VECTOR('',#20903,1.);
#5875=VECTOR('',#20904,1.);
#5876=VECTOR('',#20907,1.);
#5877=VECTOR('',#20908,1.);
#5878=VECTOR('',#20911,1.);
#5879=VECTOR('',#20912,1.);
#5880=VECTOR('',#20915,1.);
#5881=VECTOR('',#20916,1.);
#5882=VECTOR('',#20919,1.);
#5883=VECTOR('',#20920,1.);
#5884=VECTOR('',#20923,1.);
#5885=VECTOR('',#20926,1.);
#5886=VECTOR('',#20931,1.);
#5887=VECTOR('',#20934,1.);
#5888=VECTOR('',#20935,1.);
#5889=VECTOR('',#20938,1.);
#5890=VECTOR('',#20941,1.);
#5891=VECTOR('',#20944,1.);
#5892=VECTOR('',#20945,1.);
#5893=VECTOR('',#20948,1.);
#5894=VECTOR('',#20955,1.);
#5895=VECTOR('',#20964,1.);
#5896=VECTOR('',#20965,1.);
#5897=VECTOR('',#20968,1.);
#5898=VECTOR('',#20971,1.);
#5899=VECTOR('',#20972,1.);
#5900=VECTOR('',#20975,1.);
#5901=VECTOR('',#20978,1.);
#5902=VECTOR('',#20979,1.);
#5903=VECTOR('',#20982,1.);
#5904=VECTOR('',#20985,1.);
#5905=VECTOR('',#20986,1.);
#5906=VECTOR('',#20989,1.);
#5907=VECTOR('',#20992,1.);
#5908=VECTOR('',#20993,1.);
#5909=VECTOR('',#20996,1.);
#5910=VECTOR('',#20999,1.);
#5911=VECTOR('',#21000,1.);
#5912=VECTOR('',#21003,1.);
#5913=VECTOR('',#21006,1.);
#5914=VECTOR('',#21007,1.);
#5915=VECTOR('',#21010,1.);
#5916=VECTOR('',#21013,1.);
#5917=VECTOR('',#21014,1.);
#5918=VECTOR('',#21017,1.);
#5919=VECTOR('',#21020,1.);
#5920=VECTOR('',#21021,1.);
#5921=VECTOR('',#21024,1.);
#5922=VECTOR('',#21027,1.);
#5923=VECTOR('',#21028,1.);
#5924=VECTOR('',#21031,1.);
#5925=VECTOR('',#21034,1.);
#5926=VECTOR('',#21035,1.);
#5927=VECTOR('',#21038,1.);
#5928=VECTOR('',#21041,1.);
#5929=VECTOR('',#21042,1.);
#5930=VECTOR('',#21045,1.);
#5931=VECTOR('',#21048,1.);
#5932=VECTOR('',#21049,1.);
#5933=VECTOR('',#21052,1.);
#5934=VECTOR('',#21055,1.);
#5935=VECTOR('',#21056,1.);
#5936=VECTOR('',#21059,1.);
#5937=VECTOR('',#21062,1.);
#5938=VECTOR('',#21063,1.);
#5939=VECTOR('',#21066,1.);
#5940=VECTOR('',#21069,1.);
#5941=VECTOR('',#21070,1.);
#5942=VECTOR('',#21073,1.);
#5943=VECTOR('',#21076,1.);
#5944=VECTOR('',#21077,1.);
#5945=VECTOR('',#21080,1.);
#5946=VECTOR('',#21083,1.);
#5947=VECTOR('',#21084,1.);
#5948=VECTOR('',#21087,1.);
#5949=VECTOR('',#21090,1.);
#5950=VECTOR('',#21091,1.);
#5951=VECTOR('',#21094,1.);
#5952=VECTOR('',#21097,1.);
#5953=VECTOR('',#21098,1.);
#5954=VECTOR('',#21101,1.);
#5955=VECTOR('',#21104,1.);
#5956=VECTOR('',#21105,1.);
#5957=VECTOR('',#21108,1.);
#5958=VECTOR('',#21111,1.);
#5959=VECTOR('',#21112,1.);
#5960=VECTOR('',#21115,1.);
#5961=VECTOR('',#21118,1.);
#5962=VECTOR('',#21119,1.);
#5963=VECTOR('',#21122,1.);
#5964=VECTOR('',#21125,1.);
#5965=VECTOR('',#21126,1.);
#5966=VECTOR('',#21129,1.);
#5967=VECTOR('',#21132,1.);
#5968=VECTOR('',#21133,1.);
#5969=VECTOR('',#21136,1.);
#5970=VECTOR('',#21139,1.);
#5971=VECTOR('',#21140,1.);
#5972=VECTOR('',#21143,1.);
#5973=VECTOR('',#21146,1.);
#5974=VECTOR('',#21147,1.);
#5975=VECTOR('',#21150,1.);
#5976=VECTOR('',#21153,1.);
#5977=VECTOR('',#21154,1.);
#5978=VECTOR('',#21157,1.);
#5979=VECTOR('',#21160,1.);
#5980=VECTOR('',#21161,1.);
#5981=VECTOR('',#21164,1.);
#5982=VECTOR('',#21167,1.);
#5983=VECTOR('',#21168,1.);
#5984=VECTOR('',#21171,1.);
#5985=VECTOR('',#21174,1.);
#5986=VECTOR('',#21175,1.);
#5987=VECTOR('',#21178,1.);
#5988=VECTOR('',#21181,1.);
#5989=VECTOR('',#21182,1.);
#5990=VECTOR('',#21185,1.);
#5991=VECTOR('',#21188,1.);
#5992=VECTOR('',#21189,1.);
#5993=VECTOR('',#21192,1.);
#5994=VECTOR('',#21195,1.);
#5995=VECTOR('',#21196,1.);
#5996=VECTOR('',#21199,1.);
#5997=VECTOR('',#21202,1.);
#5998=VECTOR('',#21203,1.);
#5999=VECTOR('',#21206,1.);
#6000=VECTOR('',#21209,1.);
#6001=VECTOR('',#21210,1.);
#6002=VECTOR('',#21213,1.);
#6003=VECTOR('',#21364,0.18);
#6004=VECTOR('',#21369,0.33);
#7076=VERTEX_POINT('',#32270);
#7077=VERTEX_POINT('',#32271);
#7078=VERTEX_POINT('',#32273);
#7079=VERTEX_POINT('',#32284);
#7080=VERTEX_POINT('',#32294);
#7081=VERTEX_POINT('',#32295);
#7082=VERTEX_POINT('',#32342);
#7083=VERTEX_POINT('',#32343);
#7084=VERTEX_POINT('',#32390);
#7085=VERTEX_POINT('',#32391);
#7086=VERTEX_POINT('',#32441);
#7087=VERTEX_POINT('',#32442);
#7088=VERTEX_POINT('',#32492);
#7089=VERTEX_POINT('',#32493);
#7090=VERTEX_POINT('',#32540);
#7091=VERTEX_POINT('',#32541);
#7092=VERTEX_POINT('',#32588);
#7093=VERTEX_POINT('',#32589);
#7094=VERTEX_POINT('',#32642);
#7095=VERTEX_POINT('',#32643);
#7096=VERTEX_POINT('',#32690);
#7097=VERTEX_POINT('',#32691);
#7098=VERTEX_POINT('',#32738);
#7099=VERTEX_POINT('',#32739);
#7100=VERTEX_POINT('',#32792);
#7101=VERTEX_POINT('',#32793);
#7102=VERTEX_POINT('',#32840);
#7103=VERTEX_POINT('',#32841);
#7104=VERTEX_POINT('',#32888);
#7105=VERTEX_POINT('',#32889);
#7106=VERTEX_POINT('',#32936);
#7107=VERTEX_POINT('',#32937);
#7108=VERTEX_POINT('',#32990);
#7109=VERTEX_POINT('',#32991);
#7110=VERTEX_POINT('',#33038);
#7111=VERTEX_POINT('',#33039);
#7112=VERTEX_POINT('',#33086);
#7113=VERTEX_POINT('',#33087);
#7114=VERTEX_POINT('',#33140);
#7115=VERTEX_POINT('',#33141);
#7116=VERTEX_POINT('',#33188);
#7117=VERTEX_POINT('',#33189);
#7118=VERTEX_POINT('',#33236);
#7119=VERTEX_POINT('',#33237);
#7120=VERTEX_POINT('',#33290);
#7121=VERTEX_POINT('',#33291);
#7122=VERTEX_POINT('',#33338);
#7123=VERTEX_POINT('',#33339);
#7124=VERTEX_POINT('',#33341);
#7125=VERTEX_POINT('',#33348);
#7126=VERTEX_POINT('',#33356);
#7127=VERTEX_POINT('',#33357);
#7128=VERTEX_POINT('',#33380);
#7129=VERTEX_POINT('',#33381);
#7130=VERTEX_POINT('',#33405);
#7131=VERTEX_POINT('',#33406);
#7132=VERTEX_POINT('',#33430);
#7133=VERTEX_POINT('',#33431);
#7134=VERTEX_POINT('',#33454);
#7135=VERTEX_POINT('',#33455);
#7136=VERTEX_POINT('',#33479);
#7137=VERTEX_POINT('',#33480);
#7138=VERTEX_POINT('',#33504);
#7139=VERTEX_POINT('',#33505);
#7140=VERTEX_POINT('',#33528);
#7141=VERTEX_POINT('',#33529);
#7142=VERTEX_POINT('',#33553);
#7143=VERTEX_POINT('',#33554);
#7144=VERTEX_POINT('',#33578);
#7145=VERTEX_POINT('',#33579);
#7146=VERTEX_POINT('',#33602);
#7147=VERTEX_POINT('',#33603);
#7148=VERTEX_POINT('',#33626);
#7149=VERTEX_POINT('',#33627);
#7150=VERTEX_POINT('',#33651);
#7151=VERTEX_POINT('',#33652);
#7152=VERTEX_POINT('',#33676);
#7153=VERTEX_POINT('',#33677);
#7154=VERTEX_POINT('',#33700);
#7155=VERTEX_POINT('',#33701);
#7156=VERTEX_POINT('',#33725);
#7157=VERTEX_POINT('',#33726);
#7158=VERTEX_POINT('',#33750);
#7159=VERTEX_POINT('',#33751);
#7160=VERTEX_POINT('',#33774);
#7161=VERTEX_POINT('',#33775);
#7162=VERTEX_POINT('',#33799);
#7163=VERTEX_POINT('',#33800);
#7164=VERTEX_POINT('',#33823);
#7165=VERTEX_POINT('',#33824);
#7166=VERTEX_POINT('',#33848);
#7167=VERTEX_POINT('',#33849);
#7168=VERTEX_POINT('',#33872);
#7169=VERTEX_POINT('',#33925);
#7170=VERTEX_POINT('',#33927);
#7171=VERTEX_POINT('',#34576);
#7172=VERTEX_POINT('',#34639);
#7173=VERTEX_POINT('',#34642);
#7174=VERTEX_POINT('',#35298);
#7175=VERTEX_POINT('',#35304);
#7176=VERTEX_POINT('',#35305);
#7177=VERTEX_POINT('',#35307);
#7178=VERTEX_POINT('',#35309);
#7179=VERTEX_POINT('',#35311);
#7180=VERTEX_POINT('',#35313);
#7181=VERTEX_POINT('',#35315);
#7182=VERTEX_POINT('',#35317);
#7183=VERTEX_POINT('',#35319);
#7184=VERTEX_POINT('',#35321);
#7185=VERTEX_POINT('',#35323);
#7186=VERTEX_POINT('',#35325);
#7187=VERTEX_POINT('',#35327);
#7188=VERTEX_POINT('',#35329);
#7189=VERTEX_POINT('',#35331);
#7190=VERTEX_POINT('',#35333);
#7191=VERTEX_POINT('',#35335);
#7192=VERTEX_POINT('',#35337);
#7193=VERTEX_POINT('',#35339);
#7194=VERTEX_POINT('',#35341);
#7195=VERTEX_POINT('',#35343);
#7196=VERTEX_POINT('',#35345);
#7197=VERTEX_POINT('',#35347);
#7198=VERTEX_POINT('',#35349);
#7199=VERTEX_POINT('',#35351);
#7200=VERTEX_POINT('',#35353);
#7201=VERTEX_POINT('',#35355);
#7202=VERTEX_POINT('',#35357);
#7203=VERTEX_POINT('',#35359);
#7204=VERTEX_POINT('',#35361);
#7205=VERTEX_POINT('',#35363);
#7206=VERTEX_POINT('',#35365);
#7207=VERTEX_POINT('',#35367);
#7208=VERTEX_POINT('',#35369);
#7209=VERTEX_POINT('',#35371);
#7210=VERTEX_POINT('',#35373);
#7211=VERTEX_POINT('',#35375);
#7212=VERTEX_POINT('',#35377);
#7213=VERTEX_POINT('',#35379);
#7214=VERTEX_POINT('',#35381);
#7215=VERTEX_POINT('',#35383);
#7216=VERTEX_POINT('',#35385);
#7217=VERTEX_POINT('',#35387);
#7218=VERTEX_POINT('',#35389);
#7219=VERTEX_POINT('',#35391);
#7220=VERTEX_POINT('',#35393);
#7221=VERTEX_POINT('',#35395);
#7222=VERTEX_POINT('',#35397);
#7223=VERTEX_POINT('',#35399);
#7224=VERTEX_POINT('',#35401);
#7225=VERTEX_POINT('',#35403);
#7226=VERTEX_POINT('',#35405);
#7227=VERTEX_POINT('',#35407);
#7228=VERTEX_POINT('',#35409);
#7229=VERTEX_POINT('',#35411);
#7230=VERTEX_POINT('',#35413);
#7231=VERTEX_POINT('',#35415);
#7232=VERTEX_POINT('',#35417);
#7233=VERTEX_POINT('',#35419);
#7234=VERTEX_POINT('',#35421);
#7235=VERTEX_POINT('',#35423);
#7236=VERTEX_POINT('',#35425);
#7237=VERTEX_POINT('',#35427);
#7238=VERTEX_POINT('',#35429);
#7239=VERTEX_POINT('',#35431);
#7240=VERTEX_POINT('',#35433);
#7241=VERTEX_POINT('',#35435);
#7242=VERTEX_POINT('',#35437);
#7243=VERTEX_POINT('',#35439);
#7244=VERTEX_POINT('',#35441);
#7245=VERTEX_POINT('',#35443);
#7246=VERTEX_POINT('',#35445);
#7247=VERTEX_POINT('',#35447);
#7248=VERTEX_POINT('',#35449);
#7249=VERTEX_POINT('',#35451);
#7250=VERTEX_POINT('',#35453);
#7251=VERTEX_POINT('',#35455);
#7252=VERTEX_POINT('',#35457);
#7253=VERTEX_POINT('',#35459);
#7254=VERTEX_POINT('',#35461);
#7255=VERTEX_POINT('',#35463);
#7256=VERTEX_POINT('',#35465);
#7257=VERTEX_POINT('',#35467);
#7258=VERTEX_POINT('',#35469);
#7259=VERTEX_POINT('',#35471);
#7260=VERTEX_POINT('',#35473);
#7261=VERTEX_POINT('',#35475);
#7262=VERTEX_POINT('',#35477);
#7263=VERTEX_POINT('',#35479);
#7264=VERTEX_POINT('',#35481);
#7265=VERTEX_POINT('',#35483);
#7266=VERTEX_POINT('',#35485);
#7267=VERTEX_POINT('',#35487);
#7268=VERTEX_POINT('',#35489);
#7269=VERTEX_POINT('',#35491);
#7270=VERTEX_POINT('',#35493);
#7271=VERTEX_POINT('',#35495);
#7272=VERTEX_POINT('',#35497);
#7273=VERTEX_POINT('',#35499);
#7274=VERTEX_POINT('',#35501);
#7275=VERTEX_POINT('',#35503);
#7276=VERTEX_POINT('',#35505);
#7277=VERTEX_POINT('',#35507);
#7278=VERTEX_POINT('',#35509);
#7279=VERTEX_POINT('',#35511);
#7280=VERTEX_POINT('',#35513);
#7281=VERTEX_POINT('',#35515);
#7282=VERTEX_POINT('',#35517);
#7283=VERTEX_POINT('',#35521);
#7284=VERTEX_POINT('',#35522);
#7285=VERTEX_POINT('',#35526);
#7286=VERTEX_POINT('',#35530);
#7287=VERTEX_POINT('',#35534);
#7288=VERTEX_POINT('',#35538);
#7289=VERTEX_POINT('',#35545);
#7290=VERTEX_POINT('',#35546);
#7291=VERTEX_POINT('',#35548);
#7292=VERTEX_POINT('',#35553);
#7293=VERTEX_POINT('',#35557);
#7294=VERTEX_POINT('',#35562);
#7295=VERTEX_POINT('',#35566);
#7296=VERTEX_POINT('',#35571);
#7297=VERTEX_POINT('',#35575);
#7298=VERTEX_POINT('',#35580);
#7299=VERTEX_POINT('',#35584);
#7300=VERTEX_POINT('',#35589);
#7301=VERTEX_POINT('',#35593);
#7302=VERTEX_POINT('',#35598);
#7303=VERTEX_POINT('',#35604);
#7304=VERTEX_POINT('',#35606);
#7305=VERTEX_POINT('',#35610);
#7306=VERTEX_POINT('',#35614);
#7307=VERTEX_POINT('',#35618);
#7308=VERTEX_POINT('',#35622);
#7309=VERTEX_POINT('',#35626);
#7310=VERTEX_POINT('',#35630);
#7311=VERTEX_POINT('',#35634);
#7312=VERTEX_POINT('',#35638);
#7313=VERTEX_POINT('',#35649);
#7314=VERTEX_POINT('',#35657);
#7315=VERTEX_POINT('',#35670);
#7316=VERTEX_POINT('',#35671);
#7317=VERTEX_POINT('',#35678);
#7318=VERTEX_POINT('',#35684);
#7319=VERTEX_POINT('',#35685);
#7320=VERTEX_POINT('',#35692);
#7321=VERTEX_POINT('',#35698);
#7322=VERTEX_POINT('',#35699);
#7323=VERTEX_POINT('',#35706);
#7324=VERTEX_POINT('',#35712);
#7325=VERTEX_POINT('',#35713);
#7326=VERTEX_POINT('',#35720);
#7327=VERTEX_POINT('',#35726);
#7328=VERTEX_POINT('',#35727);
#7329=VERTEX_POINT('',#35734);
#7330=VERTEX_POINT('',#35740);
#7331=VERTEX_POINT('',#35741);
#7332=VERTEX_POINT('',#35748);
#7333=VERTEX_POINT('',#35754);
#7334=VERTEX_POINT('',#35755);
#7335=VERTEX_POINT('',#35762);
#7336=VERTEX_POINT('',#35768);
#7337=VERTEX_POINT('',#35769);
#7338=VERTEX_POINT('',#35776);
#7339=VERTEX_POINT('',#35782);
#7340=VERTEX_POINT('',#35783);
#7341=VERTEX_POINT('',#35790);
#7342=VERTEX_POINT('',#35796);
#7343=VERTEX_POINT('',#35797);
#7344=VERTEX_POINT('',#35804);
#7345=VERTEX_POINT('',#35810);
#7346=VERTEX_POINT('',#35811);
#7347=VERTEX_POINT('',#35818);
#7348=VERTEX_POINT('',#35824);
#7349=VERTEX_POINT('',#35825);
#7350=VERTEX_POINT('',#35832);
#7351=VERTEX_POINT('',#35838);
#7352=VERTEX_POINT('',#35839);
#7353=VERTEX_POINT('',#35846);
#7354=VERTEX_POINT('',#35852);
#7355=VERTEX_POINT('',#35853);
#7356=VERTEX_POINT('',#35860);
#7357=VERTEX_POINT('',#35866);
#7358=VERTEX_POINT('',#35867);
#7359=VERTEX_POINT('',#35874);
#7360=VERTEX_POINT('',#35880);
#7361=VERTEX_POINT('',#35881);
#7362=VERTEX_POINT('',#35888);
#7363=VERTEX_POINT('',#35894);
#7364=VERTEX_POINT('',#35895);
#7365=VERTEX_POINT('',#35902);
#7366=VERTEX_POINT('',#35908);
#7367=VERTEX_POINT('',#35909);
#7368=VERTEX_POINT('',#35916);
#7369=VERTEX_POINT('',#35922);
#7370=VERTEX_POINT('',#35923);
#7371=VERTEX_POINT('',#35930);
#7372=VERTEX_POINT('',#35936);
#7373=VERTEX_POINT('',#35937);
#7374=VERTEX_POINT('',#35944);
#7375=VERTEX_POINT('',#35950);
#7376=VERTEX_POINT('',#35951);
#7377=VERTEX_POINT('',#35958);
#7378=VERTEX_POINT('',#35964);
#7379=VERTEX_POINT('',#35965);
#7380=VERTEX_POINT('',#35972);
#7381=VERTEX_POINT('',#35978);
#7382=VERTEX_POINT('',#35979);
#7383=VERTEX_POINT('',#35986);
#7384=VERTEX_POINT('',#35992);
#7385=VERTEX_POINT('',#35993);
#7386=VERTEX_POINT('',#36000);
#7387=VERTEX_POINT('',#36006);
#7388=VERTEX_POINT('',#36007);
#7389=VERTEX_POINT('',#36014);
#7390=VERTEX_POINT('',#36020);
#7391=VERTEX_POINT('',#36021);
#7392=VERTEX_POINT('',#36028);
#7393=VERTEX_POINT('',#36034);
#7394=VERTEX_POINT('',#36035);
#7395=VERTEX_POINT('',#36042);
#7396=VERTEX_POINT('',#36048);
#7397=VERTEX_POINT('',#36049);
#7398=VERTEX_POINT('',#36056);
#7399=VERTEX_POINT('',#36062);
#7400=VERTEX_POINT('',#36063);
#7401=VERTEX_POINT('',#36070);
#7402=VERTEX_POINT('',#36076);
#7403=VERTEX_POINT('',#36077);
#7404=VERTEX_POINT('',#36084);
#7405=VERTEX_POINT('',#36090);
#7406=VERTEX_POINT('',#36091);
#7407=VERTEX_POINT('',#36098);
#7408=VERTEX_POINT('',#36104);
#7409=VERTEX_POINT('',#36105);
#7410=VERTEX_POINT('',#36112);
#7411=VERTEX_POINT('',#36118);
#7412=VERTEX_POINT('',#36119);
#7413=VERTEX_POINT('',#36126);
#7414=VERTEX_POINT('',#36132);
#7415=VERTEX_POINT('',#36133);
#7416=VERTEX_POINT('',#36140);
#7417=VERTEX_POINT('',#36146);
#7418=VERTEX_POINT('',#36147);
#7419=VERTEX_POINT('',#36154);
#7420=VERTEX_POINT('',#36160);
#7421=VERTEX_POINT('',#36161);
#7422=VERTEX_POINT('',#36168);
#7423=VERTEX_POINT('',#36246);
#7424=VERTEX_POINT('',#36251);
#9177=EDGE_CURVE('',#7076,#7077,#4518,.T.);
#9178=EDGE_CURVE('',#7076,#7078,#729,.T.);
#9179=EDGE_CURVE('',#7078,#7079,#1518,.T.);
#9180=EDGE_CURVE('',#7079,#7077,#730,.T.);
#9181=EDGE_CURVE('',#7080,#7081,#4519,.T.);
#9182=EDGE_CURVE('',#7080,#7076,#731,.T.);
#9183=EDGE_CURVE('',#7077,#7081,#732,.T.);
#9184=EDGE_CURVE('',#7082,#7083,#4520,.T.);
#9185=EDGE_CURVE('',#7082,#7080,#733,.T.);
#9186=EDGE_CURVE('',#7081,#7083,#734,.T.);
#9187=EDGE_CURVE('',#7084,#7085,#4521,.T.);
#9188=EDGE_CURVE('',#7084,#7082,#735,.T.);
#9189=EDGE_CURVE('',#7083,#7085,#736,.T.);
#9190=EDGE_CURVE('',#7086,#7087,#4522,.T.);
#9191=EDGE_CURVE('',#7086,#7084,#737,.T.);
#9192=EDGE_CURVE('',#7085,#7087,#738,.T.);
#9193=EDGE_CURVE('',#7088,#7089,#4523,.T.);
#9194=EDGE_CURVE('',#7088,#7086,#739,.T.);
#9195=EDGE_CURVE('',#7087,#7089,#740,.T.);
#9196=EDGE_CURVE('',#7090,#7091,#4524,.T.);
#9197=EDGE_CURVE('',#7090,#7088,#741,.T.);
#9198=EDGE_CURVE('',#7089,#7091,#742,.T.);
#9199=EDGE_CURVE('',#7092,#7093,#4525,.T.);
#9200=EDGE_CURVE('',#7092,#7090,#743,.T.);
#9201=EDGE_CURVE('',#7091,#7093,#744,.T.);
#9202=EDGE_CURVE('',#7094,#7095,#4526,.T.);
#9203=EDGE_CURVE('',#7094,#7092,#745,.T.);
#9204=EDGE_CURVE('',#7093,#7095,#746,.T.);
#9205=EDGE_CURVE('',#7096,#7097,#4527,.T.);
#9206=EDGE_CURVE('',#7096,#7094,#747,.T.);
#9207=EDGE_CURVE('',#7095,#7097,#748,.T.);
#9208=EDGE_CURVE('',#7098,#7099,#4528,.T.);
#9209=EDGE_CURVE('',#7098,#7096,#749,.T.);
#9210=EDGE_CURVE('',#7097,#7099,#750,.T.);
#9211=EDGE_CURVE('',#7100,#7101,#4529,.T.);
#9212=EDGE_CURVE('',#7100,#7098,#751,.T.);
#9213=EDGE_CURVE('',#7099,#7101,#752,.T.);
#9214=EDGE_CURVE('',#7102,#7103,#4530,.T.);
#9215=EDGE_CURVE('',#7102,#7100,#753,.T.);
#9216=EDGE_CURVE('',#7101,#7103,#754,.T.);
#9217=EDGE_CURVE('',#7104,#7105,#4531,.T.);
#9218=EDGE_CURVE('',#7104,#7102,#755,.T.);
#9219=EDGE_CURVE('',#7103,#7105,#756,.T.);
#9220=EDGE_CURVE('',#7106,#7107,#4532,.T.);
#9221=EDGE_CURVE('',#7106,#7104,#757,.T.);
#9222=EDGE_CURVE('',#7105,#7107,#758,.T.);
#9223=EDGE_CURVE('',#7108,#7109,#4533,.T.);
#9224=EDGE_CURVE('',#7108,#7106,#759,.T.);
#9225=EDGE_CURVE('',#7107,#7109,#760,.T.);
#9226=EDGE_CURVE('',#7110,#7111,#4534,.T.);
#9227=EDGE_CURVE('',#7110,#7108,#761,.T.);
#9228=EDGE_CURVE('',#7109,#7111,#762,.T.);
#9229=EDGE_CURVE('',#7112,#7113,#4535,.T.);
#9230=EDGE_CURVE('',#7112,#7110,#763,.T.);
#9231=EDGE_CURVE('',#7111,#7113,#764,.T.);
#9232=EDGE_CURVE('',#7114,#7115,#4536,.T.);
#9233=EDGE_CURVE('',#7114,#7112,#765,.T.);
#9234=EDGE_CURVE('',#7113,#7115,#766,.T.);
#9235=EDGE_CURVE('',#7116,#7117,#4537,.T.);
#9236=EDGE_CURVE('',#7116,#7114,#767,.T.);
#9237=EDGE_CURVE('',#7115,#7117,#768,.T.);
#9238=EDGE_CURVE('',#7118,#7119,#4538,.T.);
#9239=EDGE_CURVE('',#7118,#7116,#769,.T.);
#9240=EDGE_CURVE('',#7117,#7119,#770,.T.);
#9241=EDGE_CURVE('',#7120,#7121,#4539,.T.);
#9242=EDGE_CURVE('',#7120,#7118,#771,.T.);
#9243=EDGE_CURVE('',#7119,#7121,#772,.T.);
#9244=EDGE_CURVE('',#7122,#7123,#4540,.T.);
#9245=EDGE_CURVE('',#7122,#7124,#773,.T.);
#9246=EDGE_CURVE('',#7125,#7124,#1519,.T.);
#9247=EDGE_CURVE('',#7123,#7125,#774,.T.);
#9248=EDGE_CURVE('',#7126,#7127,#4541,.T.);
#9249=EDGE_CURVE('',#7126,#7122,#775,.T.);
#9250=EDGE_CURVE('',#7127,#7123,#776,.T.);
#9251=EDGE_CURVE('',#7128,#7129,#4542,.T.);
#9252=EDGE_CURVE('',#7128,#7126,#777,.T.);
#9253=EDGE_CURVE('',#7129,#7127,#778,.T.);
#9254=EDGE_CURVE('',#7130,#7131,#4543,.T.);
#9255=EDGE_CURVE('',#7130,#7128,#779,.T.);
#9256=EDGE_CURVE('',#7131,#7129,#780,.T.);
#9257=EDGE_CURVE('',#7132,#7133,#4544,.T.);
#9258=EDGE_CURVE('',#7132,#7130,#781,.T.);
#9259=EDGE_CURVE('',#7133,#7131,#782,.T.);
#9260=EDGE_CURVE('',#7134,#7135,#4545,.T.);
#9261=EDGE_CURVE('',#7134,#7132,#783,.T.);
#9262=EDGE_CURVE('',#7135,#7133,#784,.T.);
#9263=EDGE_CURVE('',#7136,#7137,#4546,.T.);
#9264=EDGE_CURVE('',#7136,#7134,#785,.T.);
#9265=EDGE_CURVE('',#7137,#7135,#786,.T.);
#9266=EDGE_CURVE('',#7138,#7139,#4547,.T.);
#9267=EDGE_CURVE('',#7138,#7136,#787,.T.);
#9268=EDGE_CURVE('',#7139,#7137,#788,.T.);
#9269=EDGE_CURVE('',#7140,#7141,#4548,.T.);
#9270=EDGE_CURVE('',#7140,#7138,#789,.T.);
#9271=EDGE_CURVE('',#7141,#7139,#790,.T.);
#9272=EDGE_CURVE('',#7142,#7143,#4549,.T.);
#9273=EDGE_CURVE('',#7142,#7140,#791,.T.);
#9274=EDGE_CURVE('',#7143,#7141,#792,.T.);
#9275=EDGE_CURVE('',#7144,#7145,#4550,.T.);
#9276=EDGE_CURVE('',#7144,#7142,#793,.T.);
#9277=EDGE_CURVE('',#7145,#7143,#794,.T.);
#9278=EDGE_CURVE('',#7146,#7147,#4551,.T.);
#9279=EDGE_CURVE('',#7146,#7144,#795,.T.);
#9280=EDGE_CURVE('',#7147,#7145,#796,.T.);
#9281=EDGE_CURVE('',#7148,#7149,#4552,.T.);
#9282=EDGE_CURVE('',#7148,#7146,#797,.T.);
#9283=EDGE_CURVE('',#7149,#7147,#798,.T.);
#9284=EDGE_CURVE('',#7150,#7151,#4553,.T.);
#9285=EDGE_CURVE('',#7150,#7148,#799,.T.);
#9286=EDGE_CURVE('',#7151,#7149,#800,.T.);
#9287=EDGE_CURVE('',#7152,#7153,#4554,.T.);
#9288=EDGE_CURVE('',#7152,#7150,#801,.T.);
#9289=EDGE_CURVE('',#7153,#7151,#802,.T.);
#9290=EDGE_CURVE('',#7154,#7155,#4555,.T.);
#9291=EDGE_CURVE('',#7154,#7152,#803,.T.);
#9292=EDGE_CURVE('',#7155,#7153,#804,.T.);
#9293=EDGE_CURVE('',#7156,#7157,#4556,.T.);
#9294=EDGE_CURVE('',#7156,#7154,#805,.T.);
#9295=EDGE_CURVE('',#7157,#7155,#806,.T.);
#9296=EDGE_CURVE('',#7158,#7159,#4557,.T.);
#9297=EDGE_CURVE('',#7158,#7156,#807,.T.);
#9298=EDGE_CURVE('',#7159,#7157,#808,.T.);
#9299=EDGE_CURVE('',#7160,#7161,#4558,.T.);
#9300=EDGE_CURVE('',#7160,#7158,#809,.T.);
#9301=EDGE_CURVE('',#7161,#7159,#810,.T.);
#9302=EDGE_CURVE('',#7162,#7163,#4559,.T.);
#9303=EDGE_CURVE('',#7162,#7160,#811,.T.);
#9304=EDGE_CURVE('',#7163,#7161,#812,.T.);
#9305=EDGE_CURVE('',#7164,#7165,#4560,.T.);
#9306=EDGE_CURVE('',#7164,#7162,#813,.T.);
#9307=EDGE_CURVE('',#7165,#7163,#814,.T.);
#9308=EDGE_CURVE('',#7166,#7167,#4561,.T.);
#9309=EDGE_CURVE('',#7166,#7164,#815,.T.);
#9310=EDGE_CURVE('',#7167,#7165,#816,.T.);
#9311=EDGE_CURVE('',#7124,#7168,#817,.T.);
#9312=EDGE_CURVE('',#7169,#7168,#1520,.T.);
#9313=EDGE_CURVE('',#7170,#7169,#1521,.T.);
#9314=EDGE_CURVE('',#7170,#7125,#818,.T.);
#9315=EDGE_CURVE('',#7121,#7170,#819,.T.);
#9316=EDGE_CURVE('',#7171,#7079,#820,.T.);
#9317=EDGE_CURVE('',#7171,#7167,#821,.T.);
#9318=EDGE_CURVE('',#7079,#7172,#1522,.T.);
#9319=EDGE_CURVE('',#7172,#7078,#1523,.T.);
#9320=EDGE_CURVE('',#7078,#7173,#822,.T.);
#9321=EDGE_CURVE('',#7173,#7171,#1524,.T.);
#9322=EDGE_CURVE('',#7173,#7166,#823,.T.);
#9323=EDGE_CURVE('',#7168,#7120,#824,.T.);
#9324=EDGE_CURVE('',#7169,#7174,#1525,.T.);
#9325=EDGE_CURVE('',#7174,#7174,#1526,.T.);
#9326=EDGE_CURVE('',#7168,#7170,#1527,.T.);
#9327=EDGE_CURVE('',#7175,#7176,#4562,.T.);
#9328=EDGE_CURVE('',#7176,#7177,#4563,.T.);
#9329=EDGE_CURVE('',#7178,#7177,#1528,.T.);
#9330=EDGE_CURVE('',#7178,#7179,#4564,.T.);
#9331=EDGE_CURVE('',#7179,#7180,#4565,.T.);
#9332=EDGE_CURVE('',#7181,#7180,#1529,.T.);
#9333=EDGE_CURVE('',#7181,#7182,#4566,.T.);
#9334=EDGE_CURVE('',#7182,#7183,#4567,.T.);
#9335=EDGE_CURVE('',#7184,#7183,#1530,.T.);
#9336=EDGE_CURVE('',#7184,#7185,#4568,.T.);
#9337=EDGE_CURVE('',#7185,#7186,#4569,.T.);
#9338=EDGE_CURVE('',#7187,#7186,#1531,.T.);
#9339=EDGE_CURVE('',#7187,#7188,#4570,.T.);
#9340=EDGE_CURVE('',#7188,#7189,#4571,.T.);
#9341=EDGE_CURVE('',#7190,#7189,#1532,.T.);
#9342=EDGE_CURVE('',#7190,#7191,#4572,.T.);
#9343=EDGE_CURVE('',#7191,#7192,#4573,.T.);
#9344=EDGE_CURVE('',#7193,#7192,#1533,.T.);
#9345=EDGE_CURVE('',#7193,#7194,#4574,.T.);
#9346=EDGE_CURVE('',#7194,#7195,#4575,.T.);
#9347=EDGE_CURVE('',#7196,#7195,#1534,.T.);
#9348=EDGE_CURVE('',#7196,#7197,#4576,.T.);
#9349=EDGE_CURVE('',#7197,#7198,#4577,.T.);
#9350=EDGE_CURVE('',#7199,#7198,#1535,.T.);
#9351=EDGE_CURVE('',#7199,#7200,#4578,.T.);
#9352=EDGE_CURVE('',#7200,#7201,#4579,.T.);
#9353=EDGE_CURVE('',#7202,#7201,#1536,.T.);
#9354=EDGE_CURVE('',#7202,#7203,#4580,.T.);
#9355=EDGE_CURVE('',#7203,#7204,#4581,.T.);
#9356=EDGE_CURVE('',#7205,#7204,#1537,.T.);
#9357=EDGE_CURVE('',#7205,#7206,#4582,.T.);
#9358=EDGE_CURVE('',#7206,#7207,#4583,.T.);
#9359=EDGE_CURVE('',#7208,#7207,#1538,.T.);
#9360=EDGE_CURVE('',#7208,#7209,#4584,.T.);
#9361=EDGE_CURVE('',#7209,#7210,#4585,.T.);
#9362=EDGE_CURVE('',#7211,#7210,#1539,.T.);
#9363=EDGE_CURVE('',#7211,#7212,#4586,.T.);
#9364=EDGE_CURVE('',#7212,#7213,#4587,.T.);
#9365=EDGE_CURVE('',#7214,#7213,#1540,.T.);
#9366=EDGE_CURVE('',#7214,#7215,#4588,.T.);
#9367=EDGE_CURVE('',#7215,#7216,#4589,.T.);
#9368=EDGE_CURVE('',#7217,#7216,#1541,.T.);
#9369=EDGE_CURVE('',#7217,#7218,#4590,.T.);
#9370=EDGE_CURVE('',#7218,#7219,#4591,.T.);
#9371=EDGE_CURVE('',#7220,#7219,#1542,.T.);
#9372=EDGE_CURVE('',#7220,#7221,#4592,.T.);
#9373=EDGE_CURVE('',#7221,#7222,#4593,.T.);
#9374=EDGE_CURVE('',#7223,#7222,#1543,.T.);
#9375=EDGE_CURVE('',#7223,#7224,#4594,.T.);
#9376=EDGE_CURVE('',#7224,#7225,#4595,.T.);
#9377=EDGE_CURVE('',#7226,#7225,#1544,.T.);
#9378=EDGE_CURVE('',#7226,#7227,#4596,.T.);
#9379=EDGE_CURVE('',#7227,#7228,#4597,.T.);
#9380=EDGE_CURVE('',#7229,#7228,#1545,.T.);
#9381=EDGE_CURVE('',#7229,#7230,#4598,.T.);
#9382=EDGE_CURVE('',#7230,#7231,#4599,.T.);
#9383=EDGE_CURVE('',#7232,#7231,#1546,.T.);
#9384=EDGE_CURVE('',#7232,#7233,#4600,.T.);
#9385=EDGE_CURVE('',#7233,#7234,#4601,.T.);
#9386=EDGE_CURVE('',#7235,#7234,#1547,.T.);
#9387=EDGE_CURVE('',#7235,#7236,#4602,.T.);
#9388=EDGE_CURVE('',#7236,#7237,#4603,.T.);
#9389=EDGE_CURVE('',#7238,#7237,#1548,.T.);
#9390=EDGE_CURVE('',#7238,#7239,#4604,.T.);
#9391=EDGE_CURVE('',#7239,#7240,#4605,.T.);
#9392=EDGE_CURVE('',#7241,#7240,#1549,.T.);
#9393=EDGE_CURVE('',#7241,#7242,#4606,.T.);
#9394=EDGE_CURVE('',#7242,#7243,#4607,.T.);
#9395=EDGE_CURVE('',#7244,#7243,#1550,.T.);
#9396=EDGE_CURVE('',#7244,#7245,#4608,.T.);
#9397=EDGE_CURVE('',#7245,#7246,#4609,.T.);
#9398=EDGE_CURVE('',#7247,#7246,#1551,.T.);
#9399=EDGE_CURVE('',#7247,#7248,#4610,.T.);
#9400=EDGE_CURVE('',#7248,#7249,#4611,.T.);
#9401=EDGE_CURVE('',#7250,#7249,#1552,.T.);
#9402=EDGE_CURVE('',#7250,#7251,#4612,.T.);
#9403=EDGE_CURVE('',#7251,#7252,#4613,.T.);
#9404=EDGE_CURVE('',#7253,#7252,#1553,.T.);
#9405=EDGE_CURVE('',#7253,#7254,#4614,.T.);
#9406=EDGE_CURVE('',#7254,#7255,#4615,.T.);
#9407=EDGE_CURVE('',#7256,#7255,#1554,.T.);
#9408=EDGE_CURVE('',#7256,#7257,#4616,.T.);
#9409=EDGE_CURVE('',#7257,#7258,#4617,.T.);
#9410=EDGE_CURVE('',#7259,#7258,#1555,.T.);
#9411=EDGE_CURVE('',#7259,#7260,#4618,.T.);
#9412=EDGE_CURVE('',#7260,#7261,#4619,.T.);
#9413=EDGE_CURVE('',#7262,#7261,#1556,.T.);
#9414=EDGE_CURVE('',#7262,#7263,#4620,.T.);
#9415=EDGE_CURVE('',#7263,#7264,#4621,.T.);
#9416=EDGE_CURVE('',#7265,#7264,#1557,.T.);
#9417=EDGE_CURVE('',#7265,#7266,#4622,.T.);
#9418=EDGE_CURVE('',#7266,#7267,#4623,.T.);
#9419=EDGE_CURVE('',#7268,#7267,#1558,.T.);
#9420=EDGE_CURVE('',#7268,#7269,#4624,.T.);
#9421=EDGE_CURVE('',#7269,#7270,#4625,.T.);
#9422=EDGE_CURVE('',#7271,#7270,#1559,.T.);
#9423=EDGE_CURVE('',#7271,#7272,#4626,.T.);
#9424=EDGE_CURVE('',#7272,#7273,#4627,.T.);
#9425=EDGE_CURVE('',#7274,#7273,#1560,.T.);
#9426=EDGE_CURVE('',#7274,#7275,#4628,.T.);
#9427=EDGE_CURVE('',#7275,#7276,#4629,.T.);
#9428=EDGE_CURVE('',#7277,#7276,#1561,.T.);
#9429=EDGE_CURVE('',#7277,#7278,#4630,.T.);
#9430=EDGE_CURVE('',#7278,#7279,#4631,.T.);
#9431=EDGE_CURVE('',#7280,#7279,#1562,.T.);
#9432=EDGE_CURVE('',#7280,#7281,#4632,.T.);
#9433=EDGE_CURVE('',#7281,#7282,#4633,.T.);
#9434=EDGE_CURVE('',#7175,#7282,#1563,.T.);
#9435=EDGE_CURVE('',#7283,#7284,#4634,.T.);
#9436=EDGE_CURVE('',#7284,#7283,#1564,.T.);
#9437=EDGE_CURVE('',#7284,#7285,#4635,.T.);
#9438=EDGE_CURVE('',#7285,#7284,#1565,.T.);
#9439=EDGE_CURVE('',#7285,#7286,#4636,.T.);
#9440=EDGE_CURVE('',#7286,#7285,#1566,.T.);
#9441=EDGE_CURVE('',#7286,#7287,#4637,.T.);
#9442=EDGE_CURVE('',#7287,#7286,#1567,.T.);
#9443=EDGE_CURVE('',#7287,#7288,#4638,.T.);
#9444=EDGE_CURVE('',#7288,#7287,#1568,.T.);
#9445=EDGE_CURVE('',#7288,#7283,#4639,.T.);
#9446=EDGE_CURVE('',#7283,#7288,#1569,.T.);
#9447=EDGE_CURVE('',#7289,#7290,#4640,.T.);
#9448=EDGE_CURVE('',#7291,#7290,#1570,.T.);
#9449=EDGE_CURVE('',#7285,#7291,#252,.T.);
#9450=EDGE_CURVE('',#7292,#7284,#253,.T.);
#9451=EDGE_CURVE('',#7293,#7292,#1571,.T.);
#9452=EDGE_CURVE('',#7284,#7293,#254,.T.);
#9453=EDGE_CURVE('',#7294,#7283,#255,.T.);
#9454=EDGE_CURVE('',#7295,#7294,#1572,.T.);
#9455=EDGE_CURVE('',#7283,#7295,#256,.T.);
#9456=EDGE_CURVE('',#7296,#7288,#257,.T.);
#9457=EDGE_CURVE('',#7297,#7296,#1573,.T.);
#9458=EDGE_CURVE('',#7288,#7297,#258,.T.);
#9459=EDGE_CURVE('',#7298,#7287,#259,.T.);
#9460=EDGE_CURVE('',#7299,#7298,#1574,.T.);
#9461=EDGE_CURVE('',#7287,#7299,#260,.T.);
#9462=EDGE_CURVE('',#7300,#7286,#261,.T.);
#9463=EDGE_CURVE('',#7301,#7300,#1575,.T.);
#9464=EDGE_CURVE('',#7286,#7301,#262,.T.);
#9465=EDGE_CURVE('',#7302,#7285,#263,.T.);
#9466=EDGE_CURVE('',#7290,#7302,#1576,.T.);
#9467=EDGE_CURVE('',#7303,#7286,#4641,.T.);
#9468=EDGE_CURVE('',#7304,#7303,#4642,.T.);
#9469=EDGE_CURVE('',#7304,#7285,#4643,.T.);
#9470=EDGE_CURVE('',#7285,#7305,#4644,.T.);
#9471=EDGE_CURVE('',#7305,#7302,#4645,.T.);
#9472=EDGE_CURVE('',#7306,#7287,#4646,.T.);
#9473=EDGE_CURVE('',#7303,#7306,#4647,.T.);
#9474=EDGE_CURVE('',#7299,#7307,#4648,.T.);
#9475=EDGE_CURVE('',#7287,#7307,#4649,.T.);
#9476=EDGE_CURVE('',#7286,#7308,#4650,.T.);
#9477=EDGE_CURVE('',#7308,#7300,#4651,.T.);
#9478=EDGE_CURVE('',#7309,#7304,#4652,.T.);
#9479=EDGE_CURVE('',#7309,#7284,#4653,.T.);
#9480=EDGE_CURVE('',#7284,#7310,#4654,.T.);
#9481=EDGE_CURVE('',#7310,#7292,#4655,.T.);
#9482=EDGE_CURVE('',#7311,#7288,#4656,.T.);
#9483=EDGE_CURVE('',#7306,#7311,#4657,.T.);
#9484=EDGE_CURVE('',#7297,#7312,#4658,.T.);
#9485=EDGE_CURVE('',#7288,#7312,#4659,.T.);
#9486=EDGE_CURVE('',#7307,#7298,#4660,.T.);
#9487=EDGE_CURVE('',#7301,#7308,#4661,.T.);
#9488=EDGE_CURVE('',#7312,#7296,#4662,.T.);
#9489=EDGE_CURVE('',#7313,#7294,#4663,.T.);
#9490=EDGE_CURVE('',#7295,#7313,#4664,.T.);
#9491=EDGE_CURVE('',#7293,#7310,#4665,.T.);
#9492=EDGE_CURVE('',#7291,#7305,#4666,.T.);
#9493=EDGE_CURVE('',#7314,#7283,#4667,.T.);
#9494=EDGE_CURVE('',#7311,#7314,#4668,.T.);
#9495=EDGE_CURVE('',#7283,#7313,#4669,.T.);
#9496=EDGE_CURVE('',#7314,#7309,#4670,.T.);
#9497=EDGE_CURVE('',#7315,#7316,#264,.T.);
#9498=EDGE_CURVE('',#7315,#7176,#4671,.T.);
#9499=EDGE_CURVE('',#7316,#7175,#4672,.T.);
#9500=EDGE_CURVE('',#7317,#7315,#265,.T.);
#9501=EDGE_CURVE('',#7177,#7317,#4673,.T.);
#9502=EDGE_CURVE('',#7318,#7319,#266,.T.);
#9503=EDGE_CURVE('',#7318,#7182,#4674,.T.);
#9504=EDGE_CURVE('',#7319,#7181,#4675,.T.);
#9505=EDGE_CURVE('',#7320,#7318,#267,.T.);
#9506=EDGE_CURVE('',#7183,#7320,#4676,.T.);
#9507=EDGE_CURVE('',#7321,#7322,#268,.T.);
#9508=EDGE_CURVE('',#7321,#7188,#4677,.T.);
#9509=EDGE_CURVE('',#7322,#7187,#4678,.T.);
#9510=EDGE_CURVE('',#7323,#7321,#269,.T.);
#9511=EDGE_CURVE('',#7189,#7323,#4679,.T.);
#9512=EDGE_CURVE('',#7324,#7325,#270,.T.);
#9513=EDGE_CURVE('',#7324,#7194,#4680,.T.);
#9514=EDGE_CURVE('',#7325,#7193,#4681,.T.);
#9515=EDGE_CURVE('',#7326,#7324,#271,.T.);
#9516=EDGE_CURVE('',#7195,#7326,#4682,.T.);
#9517=EDGE_CURVE('',#7327,#7328,#272,.T.);
#9518=EDGE_CURVE('',#7327,#7200,#4683,.T.);
#9519=EDGE_CURVE('',#7328,#7199,#4684,.T.);
#9520=EDGE_CURVE('',#7329,#7327,#273,.T.);
#9521=EDGE_CURVE('',#7201,#7329,#4685,.T.);
#9522=EDGE_CURVE('',#7330,#7331,#274,.T.);
#9523=EDGE_CURVE('',#7330,#7206,#4686,.T.);
#9524=EDGE_CURVE('',#7331,#7205,#4687,.T.);
#9525=EDGE_CURVE('',#7332,#7330,#275,.T.);
#9526=EDGE_CURVE('',#7207,#7332,#4688,.T.);
#9527=EDGE_CURVE('',#7333,#7334,#276,.T.);
#9528=EDGE_CURVE('',#7333,#7212,#4689,.T.);
#9529=EDGE_CURVE('',#7334,#7211,#4690,.T.);
#9530=EDGE_CURVE('',#7335,#7333,#277,.T.);
#9531=EDGE_CURVE('',#7213,#7335,#4691,.T.);
#9532=EDGE_CURVE('',#7336,#7337,#278,.T.);
#9533=EDGE_CURVE('',#7336,#7218,#4692,.T.);
#9534=EDGE_CURVE('',#7337,#7217,#4693,.T.);
#9535=EDGE_CURVE('',#7338,#7336,#279,.T.);
#9536=EDGE_CURVE('',#7219,#7338,#4694,.T.);
#9537=EDGE_CURVE('',#7339,#7340,#280,.T.);
#9538=EDGE_CURVE('',#7339,#7224,#4695,.T.);
#9539=EDGE_CURVE('',#7340,#7223,#4696,.T.);
#9540=EDGE_CURVE('',#7341,#7339,#281,.T.);
#9541=EDGE_CURVE('',#7225,#7341,#4697,.T.);
#9542=EDGE_CURVE('',#7342,#7343,#282,.T.);
#9543=EDGE_CURVE('',#7342,#7227,#4698,.T.);
#9544=EDGE_CURVE('',#7343,#7226,#4699,.T.);
#9545=EDGE_CURVE('',#7344,#7342,#283,.T.);
#9546=EDGE_CURVE('',#7228,#7344,#4700,.T.);
#9547=EDGE_CURVE('',#7345,#7346,#284,.T.);
#9548=EDGE_CURVE('',#7345,#7233,#4701,.T.);
#9549=EDGE_CURVE('',#7346,#7232,#4702,.T.);
#9550=EDGE_CURVE('',#7347,#7345,#285,.T.);
#9551=EDGE_CURVE('',#7234,#7347,#4703,.T.);
#9552=EDGE_CURVE('',#7348,#7349,#286,.T.);
#9553=EDGE_CURVE('',#7348,#7239,#4704,.T.);
#9554=EDGE_CURVE('',#7349,#7238,#4705,.T.);
#9555=EDGE_CURVE('',#7350,#7348,#287,.T.);
#9556=EDGE_CURVE('',#7240,#7350,#4706,.T.);
#9557=EDGE_CURVE('',#7351,#7352,#288,.T.);
#9558=EDGE_CURVE('',#7351,#7245,#4707,.T.);
#9559=EDGE_CURVE('',#7352,#7244,#4708,.T.);
#9560=EDGE_CURVE('',#7353,#7351,#289,.T.);
#9561=EDGE_CURVE('',#7246,#7353,#4709,.T.);
#9562=EDGE_CURVE('',#7354,#7355,#290,.T.);
#9563=EDGE_CURVE('',#7354,#7251,#4710,.T.);
#9564=EDGE_CURVE('',#7355,#7250,#4711,.T.);
#9565=EDGE_CURVE('',#7356,#7354,#291,.T.);
#9566=EDGE_CURVE('',#7252,#7356,#4712,.T.);
#9567=EDGE_CURVE('',#7357,#7358,#292,.T.);
#9568=EDGE_CURVE('',#7357,#7257,#4713,.T.);
#9569=EDGE_CURVE('',#7358,#7256,#4714,.T.);
#9570=EDGE_CURVE('',#7359,#7357,#293,.T.);
#9571=EDGE_CURVE('',#7258,#7359,#4715,.T.);
#9572=EDGE_CURVE('',#7360,#7361,#294,.T.);
#9573=EDGE_CURVE('',#7360,#7263,#4716,.T.);
#9574=EDGE_CURVE('',#7361,#7262,#4717,.T.);
#9575=EDGE_CURVE('',#7362,#7360,#295,.T.);
#9576=EDGE_CURVE('',#7264,#7362,#4718,.T.);
#9577=EDGE_CURVE('',#7363,#7364,#296,.T.);
#9578=EDGE_CURVE('',#7363,#7269,#4719,.T.);
#9579=EDGE_CURVE('',#7364,#7268,#4720,.T.);
#9580=EDGE_CURVE('',#7365,#7363,#297,.T.);
#9581=EDGE_CURVE('',#7270,#7365,#4721,.T.);
#9582=EDGE_CURVE('',#7366,#7367,#298,.T.);
#9583=EDGE_CURVE('',#7366,#7275,#4722,.T.);
#9584=EDGE_CURVE('',#7367,#7274,#4723,.T.);
#9585=EDGE_CURVE('',#7368,#7366,#299,.T.);
#9586=EDGE_CURVE('',#7276,#7368,#4724,.T.);
#9587=EDGE_CURVE('',#7369,#7370,#300,.T.);
#9588=EDGE_CURVE('',#7369,#7272,#4725,.T.);
#9589=EDGE_CURVE('',#7370,#7271,#4726,.T.);
#9590=EDGE_CURVE('',#7371,#7369,#301,.T.);
#9591=EDGE_CURVE('',#7273,#7371,#4727,.T.);
#9592=EDGE_CURVE('',#7372,#7373,#302,.T.);
#9593=EDGE_CURVE('',#7372,#7266,#4728,.T.);
#9594=EDGE_CURVE('',#7373,#7265,#4729,.T.);
#9595=EDGE_CURVE('',#7374,#7372,#303,.T.);
#9596=EDGE_CURVE('',#7267,#7374,#4730,.T.);
#9597=EDGE_CURVE('',#7375,#7376,#304,.T.);
#9598=EDGE_CURVE('',#7375,#7260,#4731,.T.);
#9599=EDGE_CURVE('',#7376,#7259,#4732,.T.);
#9600=EDGE_CURVE('',#7377,#7375,#305,.T.);
#9601=EDGE_CURVE('',#7261,#7377,#4733,.T.);
#9602=EDGE_CURVE('',#7378,#7379,#306,.T.);
#9603=EDGE_CURVE('',#7378,#7254,#4734,.T.);
#9604=EDGE_CURVE('',#7379,#7253,#4735,.T.);
#9605=EDGE_CURVE('',#7380,#7378,#307,.T.);
#9606=EDGE_CURVE('',#7255,#7380,#4736,.T.);
#9607=EDGE_CURVE('',#7381,#7382,#308,.T.);
#9608=EDGE_CURVE('',#7381,#7248,#4737,.T.);
#9609=EDGE_CURVE('',#7382,#7247,#4738,.T.);
#9610=EDGE_CURVE('',#7383,#7381,#309,.T.);
#9611=EDGE_CURVE('',#7249,#7383,#4739,.T.);
#9612=EDGE_CURVE('',#7384,#7385,#310,.T.);
#9613=EDGE_CURVE('',#7384,#7242,#4740,.T.);
#9614=EDGE_CURVE('',#7385,#7241,#4741,.T.);
#9615=EDGE_CURVE('',#7386,#7384,#311,.T.);
#9616=EDGE_CURVE('',#7243,#7386,#4742,.T.);
#9617=EDGE_CURVE('',#7387,#7388,#312,.T.);
#9618=EDGE_CURVE('',#7387,#7236,#4743,.T.);
#9619=EDGE_CURVE('',#7388,#7235,#4744,.T.);
#9620=EDGE_CURVE('',#7389,#7387,#313,.T.);
#9621=EDGE_CURVE('',#7237,#7389,#4745,.T.);
#9622=EDGE_CURVE('',#7390,#7391,#314,.T.);
#9623=EDGE_CURVE('',#7390,#7230,#4746,.T.);
#9624=EDGE_CURVE('',#7391,#7229,#4747,.T.);
#9625=EDGE_CURVE('',#7392,#7390,#315,.T.);
#9626=EDGE_CURVE('',#7231,#7392,#4748,.T.);
#9627=EDGE_CURVE('',#7393,#7394,#316,.T.);
#9628=EDGE_CURVE('',#7393,#7278,#4749,.T.);
#9629=EDGE_CURVE('',#7394,#7277,#4750,.T.);
#9630=EDGE_CURVE('',#7395,#7393,#317,.T.);
#9631=EDGE_CURVE('',#7279,#7395,#4751,.T.);
#9632=EDGE_CURVE('',#7396,#7397,#318,.T.);
#9633=EDGE_CURVE('',#7396,#7221,#4752,.T.);
#9634=EDGE_CURVE('',#7397,#7220,#4753,.T.);
#9635=EDGE_CURVE('',#7398,#7396,#319,.T.);
#9636=EDGE_CURVE('',#7222,#7398,#4754,.T.);
#9637=EDGE_CURVE('',#7399,#7400,#320,.T.);
#9638=EDGE_CURVE('',#7399,#7215,#4755,.T.);
#9639=EDGE_CURVE('',#7400,#7214,#4756,.T.);
#9640=EDGE_CURVE('',#7401,#7399,#321,.T.);
#9641=EDGE_CURVE('',#7216,#7401,#4757,.T.);
#9642=EDGE_CURVE('',#7402,#7403,#322,.T.);
#9643=EDGE_CURVE('',#7402,#7209,#4758,.T.);
#9644=EDGE_CURVE('',#7403,#7208,#4759,.T.);
#9645=EDGE_CURVE('',#7404,#7402,#323,.T.);
#9646=EDGE_CURVE('',#7210,#7404,#4760,.T.);
#9647=EDGE_CURVE('',#7405,#7406,#324,.T.);
#9648=EDGE_CURVE('',#7405,#7203,#4761,.T.);
#9649=EDGE_CURVE('',#7406,#7202,#4762,.T.);
#9650=EDGE_CURVE('',#7407,#7405,#325,.T.);
#9651=EDGE_CURVE('',#7204,#7407,#4763,.T.);
#9652=EDGE_CURVE('',#7408,#7409,#326,.T.);
#9653=EDGE_CURVE('',#7408,#7197,#4764,.T.);
#9654=EDGE_CURVE('',#7409,#7196,#4765,.T.);
#9655=EDGE_CURVE('',#7410,#7408,#327,.T.);
#9656=EDGE_CURVE('',#7198,#7410,#4766,.T.);
#9657=EDGE_CURVE('',#7411,#7412,#328,.T.);
#9658=EDGE_CURVE('',#7411,#7191,#4767,.T.);
#9659=EDGE_CURVE('',#7412,#7190,#4768,.T.);
#9660=EDGE_CURVE('',#7413,#7411,#329,.T.);
#9661=EDGE_CURVE('',#7192,#7413,#4769,.T.);
#9662=EDGE_CURVE('',#7414,#7415,#330,.T.);
#9663=EDGE_CURVE('',#7414,#7185,#4770,.T.);
#9664=EDGE_CURVE('',#7415,#7184,#4771,.T.);
#9665=EDGE_CURVE('',#7416,#7414,#331,.T.);
#9666=EDGE_CURVE('',#7186,#7416,#4772,.T.);
#9667=EDGE_CURVE('',#7417,#7418,#332,.T.);
#9668=EDGE_CURVE('',#7417,#7179,#4773,.T.);
#9669=EDGE_CURVE('',#7418,#7178,#4774,.T.);
#9670=EDGE_CURVE('',#7419,#7417,#333,.T.);
#9671=EDGE_CURVE('',#7180,#7419,#4775,.T.);
#9672=EDGE_CURVE('',#7420,#7421,#334,.T.);
#9673=EDGE_CURVE('',#7420,#7281,#4776,.T.);
#9674=EDGE_CURVE('',#7421,#7280,#4777,.T.);
#9675=EDGE_CURVE('',#7422,#7420,#335,.T.);
#9676=EDGE_CURVE('',#7282,#7422,#4778,.T.);
#9677=EDGE_CURVE('',#7421,#7395,#1577,.T.);
#9678=EDGE_CURVE('',#7394,#7368,#1578,.T.);
#9679=EDGE_CURVE('',#7367,#7371,#1579,.T.);
#9680=EDGE_CURVE('',#7370,#7365,#1580,.T.);
#9681=EDGE_CURVE('',#7364,#7374,#1581,.T.);
#9682=EDGE_CURVE('',#7373,#7362,#1582,.T.);
#9683=EDGE_CURVE('',#7361,#7377,#1583,.T.);
#9684=EDGE_CURVE('',#7376,#7359,#1584,.T.);
#9685=EDGE_CURVE('',#7358,#7380,#1585,.T.);
#9686=EDGE_CURVE('',#7379,#7356,#1586,.T.);
#9687=EDGE_CURVE('',#7355,#7383,#1587,.T.);
#9688=EDGE_CURVE('',#7382,#7353,#1588,.T.);
#9689=EDGE_CURVE('',#7352,#7386,#1589,.T.);
#9690=EDGE_CURVE('',#7385,#7350,#1590,.T.);
#9691=EDGE_CURVE('',#7349,#7389,#1591,.T.);
#9692=EDGE_CURVE('',#7388,#7347,#1592,.T.);
#9693=EDGE_CURVE('',#7346,#7392,#1593,.T.);
#9694=EDGE_CURVE('',#7391,#7344,#1594,.T.);
#9695=EDGE_CURVE('',#7343,#7341,#1595,.T.);
#9696=EDGE_CURVE('',#7340,#7398,#1596,.T.);
#9697=EDGE_CURVE('',#7397,#7338,#1597,.T.);
#9698=EDGE_CURVE('',#7337,#7401,#1598,.T.);
#9699=EDGE_CURVE('',#7400,#7335,#1599,.T.);
#9700=EDGE_CURVE('',#7334,#7404,#1600,.T.);
#9701=EDGE_CURVE('',#7403,#7332,#1601,.T.);
#9702=EDGE_CURVE('',#7331,#7407,#1602,.T.);
#9703=EDGE_CURVE('',#7406,#7329,#1603,.T.);
#9704=EDGE_CURVE('',#7328,#7410,#1604,.T.);
#9705=EDGE_CURVE('',#7409,#7326,#1605,.T.);
#9706=EDGE_CURVE('',#7325,#7413,#1606,.T.);
#9707=EDGE_CURVE('',#7412,#7323,#1607,.T.);
#9708=EDGE_CURVE('',#7322,#7416,#1608,.T.);
#9709=EDGE_CURVE('',#7415,#7320,#1609,.T.);
#9710=EDGE_CURVE('',#7319,#7419,#1610,.T.);
#9711=EDGE_CURVE('',#7418,#7317,#1611,.T.);
#9712=EDGE_CURVE('',#7316,#7422,#1612,.T.);
#9713=EDGE_CURVE('',#7423,#7423,#1613,.T.);
#9714=EDGE_CURVE('',#7172,#7423,#4779,.T.);
#9715=EDGE_CURVE('',#7424,#7424,#1614,.T.);
#9716=EDGE_CURVE('',#7424,#7339,#4780,.T.);
#13123=ORIENTED_EDGE('',*,*,#9177,.F.);
#13124=ORIENTED_EDGE('',*,*,#9178,.T.);
#13125=ORIENTED_EDGE('',*,*,#9179,.T.);
#13126=ORIENTED_EDGE('',*,*,#9180,.T.);
#13127=ORIENTED_EDGE('',*,*,#9181,.F.);
#13128=ORIENTED_EDGE('',*,*,#9182,.T.);
#13129=ORIENTED_EDGE('',*,*,#9177,.T.);
#13130=ORIENTED_EDGE('',*,*,#9183,.T.);
#13131=ORIENTED_EDGE('',*,*,#9184,.F.);
#13132=ORIENTED_EDGE('',*,*,#9185,.T.);
#13133=ORIENTED_EDGE('',*,*,#9181,.T.);
#13134=ORIENTED_EDGE('',*,*,#9186,.T.);
#13135=ORIENTED_EDGE('',*,*,#9187,.F.);
#13136=ORIENTED_EDGE('',*,*,#9188,.T.);
#13137=ORIENTED_EDGE('',*,*,#9184,.T.);
#13138=ORIENTED_EDGE('',*,*,#9189,.T.);
#13139=ORIENTED_EDGE('',*,*,#9190,.F.);
#13140=ORIENTED_EDGE('',*,*,#9191,.T.);
#13141=ORIENTED_EDGE('',*,*,#9187,.T.);
#13142=ORIENTED_EDGE('',*,*,#9192,.T.);
#13143=ORIENTED_EDGE('',*,*,#9193,.F.);
#13144=ORIENTED_EDGE('',*,*,#9194,.T.);
#13145=ORIENTED_EDGE('',*,*,#9190,.T.);
#13146=ORIENTED_EDGE('',*,*,#9195,.T.);
#13147=ORIENTED_EDGE('',*,*,#9196,.F.);
#13148=ORIENTED_EDGE('',*,*,#9197,.T.);
#13149=ORIENTED_EDGE('',*,*,#9193,.T.);
#13150=ORIENTED_EDGE('',*,*,#9198,.T.);
#13151=ORIENTED_EDGE('',*,*,#9199,.F.);
#13152=ORIENTED_EDGE('',*,*,#9200,.T.);
#13153=ORIENTED_EDGE('',*,*,#9196,.T.);
#13154=ORIENTED_EDGE('',*,*,#9201,.T.);
#13155=ORIENTED_EDGE('',*,*,#9202,.F.);
#13156=ORIENTED_EDGE('',*,*,#9203,.T.);
#13157=ORIENTED_EDGE('',*,*,#9199,.T.);
#13158=ORIENTED_EDGE('',*,*,#9204,.T.);
#13159=ORIENTED_EDGE('',*,*,#9205,.F.);
#13160=ORIENTED_EDGE('',*,*,#9206,.T.);
#13161=ORIENTED_EDGE('',*,*,#9202,.T.);
#13162=ORIENTED_EDGE('',*,*,#9207,.T.);
#13163=ORIENTED_EDGE('',*,*,#9208,.F.);
#13164=ORIENTED_EDGE('',*,*,#9209,.T.);
#13165=ORIENTED_EDGE('',*,*,#9205,.T.);
#13166=ORIENTED_EDGE('',*,*,#9210,.T.);
#13167=ORIENTED_EDGE('',*,*,#9211,.F.);
#13168=ORIENTED_EDGE('',*,*,#9212,.T.);
#13169=ORIENTED_EDGE('',*,*,#9208,.T.);
#13170=ORIENTED_EDGE('',*,*,#9213,.T.);
#13171=ORIENTED_EDGE('',*,*,#9214,.F.);
#13172=ORIENTED_EDGE('',*,*,#9215,.T.);
#13173=ORIENTED_EDGE('',*,*,#9211,.T.);
#13174=ORIENTED_EDGE('',*,*,#9216,.T.);
#13175=ORIENTED_EDGE('',*,*,#9217,.F.);
#13176=ORIENTED_EDGE('',*,*,#9218,.T.);
#13177=ORIENTED_EDGE('',*,*,#9214,.T.);
#13178=ORIENTED_EDGE('',*,*,#9219,.T.);
#13179=ORIENTED_EDGE('',*,*,#9220,.F.);
#13180=ORIENTED_EDGE('',*,*,#9221,.T.);
#13181=ORIENTED_EDGE('',*,*,#9217,.T.);
#13182=ORIENTED_EDGE('',*,*,#9222,.T.);
#13183=ORIENTED_EDGE('',*,*,#9223,.F.);
#13184=ORIENTED_EDGE('',*,*,#9224,.T.);
#13185=ORIENTED_EDGE('',*,*,#9220,.T.);
#13186=ORIENTED_EDGE('',*,*,#9225,.T.);
#13187=ORIENTED_EDGE('',*,*,#9226,.F.);
#13188=ORIENTED_EDGE('',*,*,#9227,.T.);
#13189=ORIENTED_EDGE('',*,*,#9223,.T.);
#13190=ORIENTED_EDGE('',*,*,#9228,.T.);
#13191=ORIENTED_EDGE('',*,*,#9229,.F.);
#13192=ORIENTED_EDGE('',*,*,#9230,.T.);
#13193=ORIENTED_EDGE('',*,*,#9226,.T.);
#13194=ORIENTED_EDGE('',*,*,#9231,.T.);
#13195=ORIENTED_EDGE('',*,*,#9232,.F.);
#13196=ORIENTED_EDGE('',*,*,#9233,.T.);
#13197=ORIENTED_EDGE('',*,*,#9229,.T.);
#13198=ORIENTED_EDGE('',*,*,#9234,.T.);
#13199=ORIENTED_EDGE('',*,*,#9235,.F.);
#13200=ORIENTED_EDGE('',*,*,#9236,.T.);
#13201=ORIENTED_EDGE('',*,*,#9232,.T.);
#13202=ORIENTED_EDGE('',*,*,#9237,.T.);
#13203=ORIENTED_EDGE('',*,*,#9238,.F.);
#13204=ORIENTED_EDGE('',*,*,#9239,.T.);
#13205=ORIENTED_EDGE('',*,*,#9235,.T.);
#13206=ORIENTED_EDGE('',*,*,#9240,.T.);
#13207=ORIENTED_EDGE('',*,*,#9241,.F.);
#13208=ORIENTED_EDGE('',*,*,#9242,.T.);
#13209=ORIENTED_EDGE('',*,*,#9238,.T.);
#13210=ORIENTED_EDGE('',*,*,#9243,.T.);
#13211=ORIENTED_EDGE('',*,*,#9244,.F.);
#13212=ORIENTED_EDGE('',*,*,#9245,.T.);
#13213=ORIENTED_EDGE('',*,*,#9246,.F.);
#13214=ORIENTED_EDGE('',*,*,#9247,.F.);
#13215=ORIENTED_EDGE('',*,*,#9248,.F.);
#13216=ORIENTED_EDGE('',*,*,#9249,.T.);
#13217=ORIENTED_EDGE('',*,*,#9244,.T.);
#13218=ORIENTED_EDGE('',*,*,#9250,.F.);
#13219=ORIENTED_EDGE('',*,*,#9251,.F.);
#13220=ORIENTED_EDGE('',*,*,#9252,.T.);
#13221=ORIENTED_EDGE('',*,*,#9248,.T.);
#13222=ORIENTED_EDGE('',*,*,#9253,.F.);
#13223=ORIENTED_EDGE('',*,*,#9254,.F.);
#13224=ORIENTED_EDGE('',*,*,#9255,.T.);
#13225=ORIENTED_EDGE('',*,*,#9251,.T.);
#13226=ORIENTED_EDGE('',*,*,#9256,.F.);
#13227=ORIENTED_EDGE('',*,*,#9257,.F.);
#13228=ORIENTED_EDGE('',*,*,#9258,.T.);
#13229=ORIENTED_EDGE('',*,*,#9254,.T.);
#13230=ORIENTED_EDGE('',*,*,#9259,.F.);
#13231=ORIENTED_EDGE('',*,*,#9260,.F.);
#13232=ORIENTED_EDGE('',*,*,#9261,.T.);
#13233=ORIENTED_EDGE('',*,*,#9257,.T.);
#13234=ORIENTED_EDGE('',*,*,#9262,.F.);
#13235=ORIENTED_EDGE('',*,*,#9263,.F.);
#13236=ORIENTED_EDGE('',*,*,#9264,.T.);
#13237=ORIENTED_EDGE('',*,*,#9260,.T.);
#13238=ORIENTED_EDGE('',*,*,#9265,.F.);
#13239=ORIENTED_EDGE('',*,*,#9266,.F.);
#13240=ORIENTED_EDGE('',*,*,#9267,.T.);
#13241=ORIENTED_EDGE('',*,*,#9263,.T.);
#13242=ORIENTED_EDGE('',*,*,#9268,.F.);
#13243=ORIENTED_EDGE('',*,*,#9269,.F.);
#13244=ORIENTED_EDGE('',*,*,#9270,.T.);
#13245=ORIENTED_EDGE('',*,*,#9266,.T.);
#13246=ORIENTED_EDGE('',*,*,#9271,.F.);
#13247=ORIENTED_EDGE('',*,*,#9272,.F.);
#13248=ORIENTED_EDGE('',*,*,#9273,.T.);
#13249=ORIENTED_EDGE('',*,*,#9269,.T.);
#13250=ORIENTED_EDGE('',*,*,#9274,.F.);
#13251=ORIENTED_EDGE('',*,*,#9275,.F.);
#13252=ORIENTED_EDGE('',*,*,#9276,.T.);
#13253=ORIENTED_EDGE('',*,*,#9272,.T.);
#13254=ORIENTED_EDGE('',*,*,#9277,.F.);
#13255=ORIENTED_EDGE('',*,*,#9278,.F.);
#13256=ORIENTED_EDGE('',*,*,#9279,.T.);
#13257=ORIENTED_EDGE('',*,*,#9275,.T.);
#13258=ORIENTED_EDGE('',*,*,#9280,.F.);
#13259=ORIENTED_EDGE('',*,*,#9281,.F.);
#13260=ORIENTED_EDGE('',*,*,#9282,.T.);
#13261=ORIENTED_EDGE('',*,*,#9278,.T.);
#13262=ORIENTED_EDGE('',*,*,#9283,.F.);
#13263=ORIENTED_EDGE('',*,*,#9284,.F.);
#13264=ORIENTED_EDGE('',*,*,#9285,.T.);
#13265=ORIENTED_EDGE('',*,*,#9281,.T.);
#13266=ORIENTED_EDGE('',*,*,#9286,.F.);
#13267=ORIENTED_EDGE('',*,*,#9287,.F.);
#13268=ORIENTED_EDGE('',*,*,#9288,.T.);
#13269=ORIENTED_EDGE('',*,*,#9284,.T.);
#13270=ORIENTED_EDGE('',*,*,#9289,.F.);
#13271=ORIENTED_EDGE('',*,*,#9290,.F.);
#13272=ORIENTED_EDGE('',*,*,#9291,.T.);
#13273=ORIENTED_EDGE('',*,*,#9287,.T.);
#13274=ORIENTED_EDGE('',*,*,#9292,.F.);
#13275=ORIENTED_EDGE('',*,*,#9293,.F.);
#13276=ORIENTED_EDGE('',*,*,#9294,.T.);
#13277=ORIENTED_EDGE('',*,*,#9290,.T.);
#13278=ORIENTED_EDGE('',*,*,#9295,.F.);
#13279=ORIENTED_EDGE('',*,*,#9296,.F.);
#13280=ORIENTED_EDGE('',*,*,#9297,.T.);
#13281=ORIENTED_EDGE('',*,*,#9293,.T.);
#13282=ORIENTED_EDGE('',*,*,#9298,.F.);
#13283=ORIENTED_EDGE('',*,*,#9299,.F.);
#13284=ORIENTED_EDGE('',*,*,#9300,.T.);
#13285=ORIENTED_EDGE('',*,*,#9296,.T.);
#13286=ORIENTED_EDGE('',*,*,#9301,.F.);
#13287=ORIENTED_EDGE('',*,*,#9302,.F.);
#13288=ORIENTED_EDGE('',*,*,#9303,.T.);
#13289=ORIENTED_EDGE('',*,*,#9299,.T.);
#13290=ORIENTED_EDGE('',*,*,#9304,.F.);
#13291=ORIENTED_EDGE('',*,*,#9305,.F.);
#13292=ORIENTED_EDGE('',*,*,#9306,.T.);
#13293=ORIENTED_EDGE('',*,*,#9302,.T.);
#13294=ORIENTED_EDGE('',*,*,#9307,.F.);
#13295=ORIENTED_EDGE('',*,*,#9308,.F.);
#13296=ORIENTED_EDGE('',*,*,#9309,.T.);
#13297=ORIENTED_EDGE('',*,*,#9305,.T.);
#13298=ORIENTED_EDGE('',*,*,#9310,.F.);
#13299=ORIENTED_EDGE('',*,*,#9246,.T.);
#13300=ORIENTED_EDGE('',*,*,#9311,.T.);
#13301=ORIENTED_EDGE('',*,*,#9312,.F.);
#13302=ORIENTED_EDGE('',*,*,#9313,.F.);
#13303=ORIENTED_EDGE('',*,*,#9314,.T.);
#13304=ORIENTED_EDGE('',*,*,#9314,.F.);
#13305=ORIENTED_EDGE('',*,*,#9315,.F.);
#13306=ORIENTED_EDGE('',*,*,#9243,.F.);
#13307=ORIENTED_EDGE('',*,*,#9240,.F.);
#13308=ORIENTED_EDGE('',*,*,#9237,.F.);
#13309=ORIENTED_EDGE('',*,*,#9234,.F.);
#13310=ORIENTED_EDGE('',*,*,#9231,.F.);
#13311=ORIENTED_EDGE('',*,*,#9228,.F.);
#13312=ORIENTED_EDGE('',*,*,#9225,.F.);
#13313=ORIENTED_EDGE('',*,*,#9222,.F.);
#13314=ORIENTED_EDGE('',*,*,#9219,.F.);
#13315=ORIENTED_EDGE('',*,*,#9216,.F.);
#13316=ORIENTED_EDGE('',*,*,#9213,.F.);
#13317=ORIENTED_EDGE('',*,*,#9210,.F.);
#13318=ORIENTED_EDGE('',*,*,#9207,.F.);
#13319=ORIENTED_EDGE('',*,*,#9204,.F.);
#13320=ORIENTED_EDGE('',*,*,#9201,.F.);
#13321=ORIENTED_EDGE('',*,*,#9198,.F.);
#13322=ORIENTED_EDGE('',*,*,#9195,.F.);
#13323=ORIENTED_EDGE('',*,*,#9192,.F.);
#13324=ORIENTED_EDGE('',*,*,#9189,.F.);
#13325=ORIENTED_EDGE('',*,*,#9186,.F.);
#13326=ORIENTED_EDGE('',*,*,#9183,.F.);
#13327=ORIENTED_EDGE('',*,*,#9180,.F.);
#13328=ORIENTED_EDGE('',*,*,#9316,.F.);
#13329=ORIENTED_EDGE('',*,*,#9317,.T.);
#13330=ORIENTED_EDGE('',*,*,#9310,.T.);
#13331=ORIENTED_EDGE('',*,*,#9307,.T.);
#13332=ORIENTED_EDGE('',*,*,#9304,.T.);
#13333=ORIENTED_EDGE('',*,*,#9301,.T.);
#13334=ORIENTED_EDGE('',*,*,#9298,.T.);
#13335=ORIENTED_EDGE('',*,*,#9295,.T.);
#13336=ORIENTED_EDGE('',*,*,#9292,.T.);
#13337=ORIENTED_EDGE('',*,*,#9289,.T.);
#13338=ORIENTED_EDGE('',*,*,#9286,.T.);
#13339=ORIENTED_EDGE('',*,*,#9283,.T.);
#13340=ORIENTED_EDGE('',*,*,#9280,.T.);
#13341=ORIENTED_EDGE('',*,*,#9277,.T.);
#13342=ORIENTED_EDGE('',*,*,#9274,.T.);
#13343=ORIENTED_EDGE('',*,*,#9271,.T.);
#13344=ORIENTED_EDGE('',*,*,#9268,.T.);
#13345=ORIENTED_EDGE('',*,*,#9265,.T.);
#13346=ORIENTED_EDGE('',*,*,#9262,.T.);
#13347=ORIENTED_EDGE('',*,*,#9259,.T.);
#13348=ORIENTED_EDGE('',*,*,#9256,.T.);
#13349=ORIENTED_EDGE('',*,*,#9253,.T.);
#13350=ORIENTED_EDGE('',*,*,#9250,.T.);
#13351=ORIENTED_EDGE('',*,*,#9247,.T.);
#13352=ORIENTED_EDGE('',*,*,#9318,.T.);
#13353=ORIENTED_EDGE('',*,*,#9319,.T.);
#13354=ORIENTED_EDGE('',*,*,#9320,.T.);
#13355=ORIENTED_EDGE('',*,*,#9321,.T.);
#13356=ORIENTED_EDGE('',*,*,#9316,.T.);
#13357=ORIENTED_EDGE('',*,*,#9308,.T.);
#13358=ORIENTED_EDGE('',*,*,#9317,.F.);
#13359=ORIENTED_EDGE('',*,*,#9321,.F.);
#13360=ORIENTED_EDGE('',*,*,#9322,.T.);
#13361=ORIENTED_EDGE('',*,*,#9311,.F.);
#13362=ORIENTED_EDGE('',*,*,#9245,.F.);
#13363=ORIENTED_EDGE('',*,*,#9249,.F.);
#13364=ORIENTED_EDGE('',*,*,#9252,.F.);
#13365=ORIENTED_EDGE('',*,*,#9255,.F.);
#13366=ORIENTED_EDGE('',*,*,#9258,.F.);
#13367=ORIENTED_EDGE('',*,*,#9261,.F.);
#13368=ORIENTED_EDGE('',*,*,#9264,.F.);
#13369=ORIENTED_EDGE('',*,*,#9267,.F.);
#13370=ORIENTED_EDGE('',*,*,#9270,.F.);
#13371=ORIENTED_EDGE('',*,*,#9273,.F.);
#13372=ORIENTED_EDGE('',*,*,#9276,.F.);
#13373=ORIENTED_EDGE('',*,*,#9279,.F.);
#13374=ORIENTED_EDGE('',*,*,#9282,.F.);
#13375=ORIENTED_EDGE('',*,*,#9285,.F.);
#13376=ORIENTED_EDGE('',*,*,#9288,.F.);
#13377=ORIENTED_EDGE('',*,*,#9291,.F.);
#13378=ORIENTED_EDGE('',*,*,#9294,.F.);
#13379=ORIENTED_EDGE('',*,*,#9297,.F.);
#13380=ORIENTED_EDGE('',*,*,#9300,.F.);
#13381=ORIENTED_EDGE('',*,*,#9303,.F.);
#13382=ORIENTED_EDGE('',*,*,#9306,.F.);
#13383=ORIENTED_EDGE('',*,*,#9309,.F.);
#13384=ORIENTED_EDGE('',*,*,#9322,.F.);
#13385=ORIENTED_EDGE('',*,*,#9320,.F.);
#13386=ORIENTED_EDGE('',*,*,#9178,.F.);
#13387=ORIENTED_EDGE('',*,*,#9182,.F.);
#13388=ORIENTED_EDGE('',*,*,#9185,.F.);
#13389=ORIENTED_EDGE('',*,*,#9188,.F.);
#13390=ORIENTED_EDGE('',*,*,#9191,.F.);
#13391=ORIENTED_EDGE('',*,*,#9194,.F.);
#13392=ORIENTED_EDGE('',*,*,#9197,.F.);
#13393=ORIENTED_EDGE('',*,*,#9200,.F.);
#13394=ORIENTED_EDGE('',*,*,#9203,.F.);
#13395=ORIENTED_EDGE('',*,*,#9206,.F.);
#13396=ORIENTED_EDGE('',*,*,#9209,.F.);
#13397=ORIENTED_EDGE('',*,*,#9212,.F.);
#13398=ORIENTED_EDGE('',*,*,#9215,.F.);
#13399=ORIENTED_EDGE('',*,*,#9218,.F.);
#13400=ORIENTED_EDGE('',*,*,#9221,.F.);
#13401=ORIENTED_EDGE('',*,*,#9224,.F.);
#13402=ORIENTED_EDGE('',*,*,#9227,.F.);
#13403=ORIENTED_EDGE('',*,*,#9230,.F.);
#13404=ORIENTED_EDGE('',*,*,#9233,.F.);
#13405=ORIENTED_EDGE('',*,*,#9236,.F.);
#13406=ORIENTED_EDGE('',*,*,#9239,.F.);
#13407=ORIENTED_EDGE('',*,*,#9242,.F.);
#13408=ORIENTED_EDGE('',*,*,#9323,.F.);
#13409=ORIENTED_EDGE('',*,*,#9313,.T.);
#13410=ORIENTED_EDGE('',*,*,#9324,.T.);
#13411=ORIENTED_EDGE('',*,*,#9325,.T.);
#13412=ORIENTED_EDGE('',*,*,#9324,.F.);
#13413=ORIENTED_EDGE('',*,*,#9312,.T.);
#13414=ORIENTED_EDGE('',*,*,#9326,.T.);
#13415=ORIENTED_EDGE('',*,*,#9241,.T.);
#13416=ORIENTED_EDGE('',*,*,#9315,.T.);
#13417=ORIENTED_EDGE('',*,*,#9326,.F.);
#13418=ORIENTED_EDGE('',*,*,#9323,.T.);
#13419=ORIENTED_EDGE('',*,*,#9327,.T.);
#13420=ORIENTED_EDGE('',*,*,#9328,.T.);
#13421=ORIENTED_EDGE('',*,*,#9329,.F.);
#13422=ORIENTED_EDGE('',*,*,#9330,.T.);
#13423=ORIENTED_EDGE('',*,*,#9331,.T.);
#13424=ORIENTED_EDGE('',*,*,#9332,.F.);
#13425=ORIENTED_EDGE('',*,*,#9333,.T.);
#13426=ORIENTED_EDGE('',*,*,#9334,.T.);
#13427=ORIENTED_EDGE('',*,*,#9335,.F.);
#13428=ORIENTED_EDGE('',*,*,#9336,.T.);
#13429=ORIENTED_EDGE('',*,*,#9337,.T.);
#13430=ORIENTED_EDGE('',*,*,#9338,.F.);
#13431=ORIENTED_EDGE('',*,*,#9339,.T.);
#13432=ORIENTED_EDGE('',*,*,#9340,.T.);
#13433=ORIENTED_EDGE('',*,*,#9341,.F.);
#13434=ORIENTED_EDGE('',*,*,#9342,.T.);
#13435=ORIENTED_EDGE('',*,*,#9343,.T.);
#13436=ORIENTED_EDGE('',*,*,#9344,.F.);
#13437=ORIENTED_EDGE('',*,*,#9345,.T.);
#13438=ORIENTED_EDGE('',*,*,#9346,.T.);
#13439=ORIENTED_EDGE('',*,*,#9347,.F.);
#13440=ORIENTED_EDGE('',*,*,#9348,.T.);
#13441=ORIENTED_EDGE('',*,*,#9349,.T.);
#13442=ORIENTED_EDGE('',*,*,#9350,.F.);
#13443=ORIENTED_EDGE('',*,*,#9351,.T.);
#13444=ORIENTED_EDGE('',*,*,#9352,.T.);
#13445=ORIENTED_EDGE('',*,*,#9353,.F.);
#13446=ORIENTED_EDGE('',*,*,#9354,.T.);
#13447=ORIENTED_EDGE('',*,*,#9355,.T.);
#13448=ORIENTED_EDGE('',*,*,#9356,.F.);
#13449=ORIENTED_EDGE('',*,*,#9357,.T.);
#13450=ORIENTED_EDGE('',*,*,#9358,.T.);
#13451=ORIENTED_EDGE('',*,*,#9359,.F.);
#13452=ORIENTED_EDGE('',*,*,#9360,.T.);
#13453=ORIENTED_EDGE('',*,*,#9361,.T.);
#13454=ORIENTED_EDGE('',*,*,#9362,.F.);
#13455=ORIENTED_EDGE('',*,*,#9363,.T.);
#13456=ORIENTED_EDGE('',*,*,#9364,.T.);
#13457=ORIENTED_EDGE('',*,*,#9365,.F.);
#13458=ORIENTED_EDGE('',*,*,#9366,.T.);
#13459=ORIENTED_EDGE('',*,*,#9367,.T.);
#13460=ORIENTED_EDGE('',*,*,#9368,.F.);
#13461=ORIENTED_EDGE('',*,*,#9369,.T.);
#13462=ORIENTED_EDGE('',*,*,#9370,.T.);
#13463=ORIENTED_EDGE('',*,*,#9371,.F.);
#13464=ORIENTED_EDGE('',*,*,#9372,.T.);
#13465=ORIENTED_EDGE('',*,*,#9373,.T.);
#13466=ORIENTED_EDGE('',*,*,#9374,.F.);
#13467=ORIENTED_EDGE('',*,*,#9375,.T.);
#13468=ORIENTED_EDGE('',*,*,#9376,.T.);
#13469=ORIENTED_EDGE('',*,*,#9377,.F.);
#13470=ORIENTED_EDGE('',*,*,#9378,.T.);
#13471=ORIENTED_EDGE('',*,*,#9379,.T.);
#13472=ORIENTED_EDGE('',*,*,#9380,.F.);
#13473=ORIENTED_EDGE('',*,*,#9381,.T.);
#13474=ORIENTED_EDGE('',*,*,#9382,.T.);
#13475=ORIENTED_EDGE('',*,*,#9383,.F.);
#13476=ORIENTED_EDGE('',*,*,#9384,.T.);
#13477=ORIENTED_EDGE('',*,*,#9385,.T.);
#13478=ORIENTED_EDGE('',*,*,#9386,.F.);
#13479=ORIENTED_EDGE('',*,*,#9387,.T.);
#13480=ORIENTED_EDGE('',*,*,#9388,.T.);
#13481=ORIENTED_EDGE('',*,*,#9389,.F.);
#13482=ORIENTED_EDGE('',*,*,#9390,.T.);
#13483=ORIENTED_EDGE('',*,*,#9391,.T.);
#13484=ORIENTED_EDGE('',*,*,#9392,.F.);
#13485=ORIENTED_EDGE('',*,*,#9393,.T.);
#13486=ORIENTED_EDGE('',*,*,#9394,.T.);
#13487=ORIENTED_EDGE('',*,*,#9395,.F.);
#13488=ORIENTED_EDGE('',*,*,#9396,.T.);
#13489=ORIENTED_EDGE('',*,*,#9397,.T.);
#13490=ORIENTED_EDGE('',*,*,#9398,.F.);
#13491=ORIENTED_EDGE('',*,*,#9399,.T.);
#13492=ORIENTED_EDGE('',*,*,#9400,.T.);
#13493=ORIENTED_EDGE('',*,*,#9401,.F.);
#13494=ORIENTED_EDGE('',*,*,#9402,.T.);
#13495=ORIENTED_EDGE('',*,*,#9403,.T.);
#13496=ORIENTED_EDGE('',*,*,#9404,.F.);
#13497=ORIENTED_EDGE('',*,*,#9405,.T.);
#13498=ORIENTED_EDGE('',*,*,#9406,.T.);
#13499=ORIENTED_EDGE('',*,*,#9407,.F.);
#13500=ORIENTED_EDGE('',*,*,#9408,.T.);
#13501=ORIENTED_EDGE('',*,*,#9409,.T.);
#13502=ORIENTED_EDGE('',*,*,#9410,.F.);
#13503=ORIENTED_EDGE('',*,*,#9411,.T.);
#13504=ORIENTED_EDGE('',*,*,#9412,.T.);
#13505=ORIENTED_EDGE('',*,*,#9413,.F.);
#13506=ORIENTED_EDGE('',*,*,#9414,.T.);
#13507=ORIENTED_EDGE('',*,*,#9415,.T.);
#13508=ORIENTED_EDGE('',*,*,#9416,.F.);
#13509=ORIENTED_EDGE('',*,*,#9417,.T.);
#13510=ORIENTED_EDGE('',*,*,#9418,.T.);
#13511=ORIENTED_EDGE('',*,*,#9419,.F.);
#13512=ORIENTED_EDGE('',*,*,#9420,.T.);
#13513=ORIENTED_EDGE('',*,*,#9421,.T.);
#13514=ORIENTED_EDGE('',*,*,#9422,.F.);
#13515=ORIENTED_EDGE('',*,*,#9423,.T.);
#13516=ORIENTED_EDGE('',*,*,#9424,.T.);
#13517=ORIENTED_EDGE('',*,*,#9425,.F.);
#13518=ORIENTED_EDGE('',*,*,#9426,.T.);
#13519=ORIENTED_EDGE('',*,*,#9427,.T.);
#13520=ORIENTED_EDGE('',*,*,#9428,.F.);
#13521=ORIENTED_EDGE('',*,*,#9429,.T.);
#13522=ORIENTED_EDGE('',*,*,#9430,.T.);
#13523=ORIENTED_EDGE('',*,*,#9431,.F.);
#13524=ORIENTED_EDGE('',*,*,#9432,.T.);
#13525=ORIENTED_EDGE('',*,*,#9433,.T.);
#13526=ORIENTED_EDGE('',*,*,#9434,.F.);
#13527=ORIENTED_EDGE('',*,*,#9325,.F.);
#13528=ORIENTED_EDGE('',*,*,#9435,.F.);
#13529=ORIENTED_EDGE('',*,*,#9436,.F.);
#13530=ORIENTED_EDGE('',*,*,#9437,.F.);
#13531=ORIENTED_EDGE('',*,*,#9438,.F.);
#13532=ORIENTED_EDGE('',*,*,#9439,.F.);
#13533=ORIENTED_EDGE('',*,*,#9440,.F.);
#13534=ORIENTED_EDGE('',*,*,#9441,.F.);
#13535=ORIENTED_EDGE('',*,*,#9442,.F.);
#13536=ORIENTED_EDGE('',*,*,#9443,.F.);
#13537=ORIENTED_EDGE('',*,*,#9444,.F.);
#13538=ORIENTED_EDGE('',*,*,#9445,.F.);
#13539=ORIENTED_EDGE('',*,*,#9446,.F.);
#13540=ORIENTED_EDGE('',*,*,#9447,.T.);
#13541=ORIENTED_EDGE('',*,*,#9448,.F.);
#13542=ORIENTED_EDGE('',*,*,#9449,.F.);
#13543=ORIENTED_EDGE('',*,*,#9438,.T.);
#13544=ORIENTED_EDGE('',*,*,#9450,.F.);
#13545=ORIENTED_EDGE('',*,*,#9451,.F.);
#13546=ORIENTED_EDGE('',*,*,#9452,.F.);
#13547=ORIENTED_EDGE('',*,*,#9436,.T.);
#13548=ORIENTED_EDGE('',*,*,#9453,.F.);
#13549=ORIENTED_EDGE('',*,*,#9454,.F.);
#13550=ORIENTED_EDGE('',*,*,#9455,.F.);
#13551=ORIENTED_EDGE('',*,*,#9446,.T.);
#13552=ORIENTED_EDGE('',*,*,#9456,.F.);
#13553=ORIENTED_EDGE('',*,*,#9457,.F.);
#13554=ORIENTED_EDGE('',*,*,#9458,.F.);
#13555=ORIENTED_EDGE('',*,*,#9444,.T.);
#13556=ORIENTED_EDGE('',*,*,#9459,.F.);
#13557=ORIENTED_EDGE('',*,*,#9460,.F.);
#13558=ORIENTED_EDGE('',*,*,#9461,.F.);
#13559=ORIENTED_EDGE('',*,*,#9442,.T.);
#13560=ORIENTED_EDGE('',*,*,#9462,.F.);
#13561=ORIENTED_EDGE('',*,*,#9463,.F.);
#13562=ORIENTED_EDGE('',*,*,#9464,.F.);
#13563=ORIENTED_EDGE('',*,*,#9440,.T.);
#13564=ORIENTED_EDGE('',*,*,#9465,.F.);
#13565=ORIENTED_EDGE('',*,*,#9466,.F.);
#13566=ORIENTED_EDGE('',*,*,#9447,.F.);
#13567=ORIENTED_EDGE('',*,*,#9439,.T.);
#13568=ORIENTED_EDGE('',*,*,#9467,.F.);
#13569=ORIENTED_EDGE('',*,*,#9468,.F.);
#13570=ORIENTED_EDGE('',*,*,#9469,.T.);
#13571=ORIENTED_EDGE('',*,*,#9465,.T.);
#13572=ORIENTED_EDGE('',*,*,#9470,.T.);
#13573=ORIENTED_EDGE('',*,*,#9471,.T.);
#13574=ORIENTED_EDGE('',*,*,#9441,.T.);
#13575=ORIENTED_EDGE('',*,*,#9472,.F.);
#13576=ORIENTED_EDGE('',*,*,#9473,.F.);
#13577=ORIENTED_EDGE('',*,*,#9467,.T.);
#13578=ORIENTED_EDGE('',*,*,#9461,.T.);
#13579=ORIENTED_EDGE('',*,*,#9474,.T.);
#13580=ORIENTED_EDGE('',*,*,#9475,.F.);
#13581=ORIENTED_EDGE('',*,*,#9462,.T.);
#13582=ORIENTED_EDGE('',*,*,#9476,.T.);
#13583=ORIENTED_EDGE('',*,*,#9477,.T.);
#13584=ORIENTED_EDGE('',*,*,#9437,.T.);
#13585=ORIENTED_EDGE('',*,*,#9469,.F.);
#13586=ORIENTED_EDGE('',*,*,#9478,.F.);
#13587=ORIENTED_EDGE('',*,*,#9479,.T.);
#13588=ORIENTED_EDGE('',*,*,#9450,.T.);
#13589=ORIENTED_EDGE('',*,*,#9480,.T.);
#13590=ORIENTED_EDGE('',*,*,#9481,.T.);
#13591=ORIENTED_EDGE('',*,*,#9443,.T.);
#13592=ORIENTED_EDGE('',*,*,#9482,.F.);
#13593=ORIENTED_EDGE('',*,*,#9483,.F.);
#13594=ORIENTED_EDGE('',*,*,#9472,.T.);
#13595=ORIENTED_EDGE('',*,*,#9458,.T.);
#13596=ORIENTED_EDGE('',*,*,#9484,.T.);
#13597=ORIENTED_EDGE('',*,*,#9485,.F.);
#13598=ORIENTED_EDGE('',*,*,#9459,.T.);
#13599=ORIENTED_EDGE('',*,*,#9475,.T.);
#13600=ORIENTED_EDGE('',*,*,#9486,.T.);
#13601=ORIENTED_EDGE('',*,*,#9463,.T.);
#13602=ORIENTED_EDGE('',*,*,#9477,.F.);
#13603=ORIENTED_EDGE('',*,*,#9487,.F.);
#13604=ORIENTED_EDGE('',*,*,#9460,.T.);
#13605=ORIENTED_EDGE('',*,*,#9486,.F.);
#13606=ORIENTED_EDGE('',*,*,#9474,.F.);
#13607=ORIENTED_EDGE('',*,*,#9457,.T.);
#13608=ORIENTED_EDGE('',*,*,#9488,.F.);
#13609=ORIENTED_EDGE('',*,*,#9484,.F.);
#13610=ORIENTED_EDGE('',*,*,#9454,.T.);
#13611=ORIENTED_EDGE('',*,*,#9489,.F.);
#13612=ORIENTED_EDGE('',*,*,#9490,.F.);
#13613=ORIENTED_EDGE('',*,*,#9451,.T.);
#13614=ORIENTED_EDGE('',*,*,#9481,.F.);
#13615=ORIENTED_EDGE('',*,*,#9491,.F.);
#13616=ORIENTED_EDGE('',*,*,#9448,.T.);
#13617=ORIENTED_EDGE('',*,*,#9466,.T.);
#13618=ORIENTED_EDGE('',*,*,#9471,.F.);
#13619=ORIENTED_EDGE('',*,*,#9492,.F.);
#13620=ORIENTED_EDGE('',*,*,#9445,.T.);
#13621=ORIENTED_EDGE('',*,*,#9493,.F.);
#13622=ORIENTED_EDGE('',*,*,#9494,.F.);
#13623=ORIENTED_EDGE('',*,*,#9482,.T.);
#13624=ORIENTED_EDGE('',*,*,#9455,.T.);
#13625=ORIENTED_EDGE('',*,*,#9490,.T.);
#13626=ORIENTED_EDGE('',*,*,#9495,.F.);
#13627=ORIENTED_EDGE('',*,*,#9456,.T.);
#13628=ORIENTED_EDGE('',*,*,#9485,.T.);
#13629=ORIENTED_EDGE('',*,*,#9488,.T.);
#13630=ORIENTED_EDGE('',*,*,#9453,.T.);
#13631=ORIENTED_EDGE('',*,*,#9495,.T.);
#13632=ORIENTED_EDGE('',*,*,#9489,.T.);
#13633=ORIENTED_EDGE('',*,*,#9435,.T.);
#13634=ORIENTED_EDGE('',*,*,#9479,.F.);
#13635=ORIENTED_EDGE('',*,*,#9496,.F.);
#13636=ORIENTED_EDGE('',*,*,#9493,.T.);
#13637=ORIENTED_EDGE('',*,*,#9464,.T.);
#13638=ORIENTED_EDGE('',*,*,#9487,.T.);
#13639=ORIENTED_EDGE('',*,*,#9476,.F.);
#13640=ORIENTED_EDGE('',*,*,#9449,.T.);
#13641=ORIENTED_EDGE('',*,*,#9492,.T.);
#13642=ORIENTED_EDGE('',*,*,#9470,.F.);
#13643=ORIENTED_EDGE('',*,*,#9452,.T.);
#13644=ORIENTED_EDGE('',*,*,#9491,.T.);
#13645=ORIENTED_EDGE('',*,*,#9480,.F.);
#13646=ORIENTED_EDGE('',*,*,#9497,.F.);
#13647=ORIENTED_EDGE('',*,*,#9498,.T.);
#13648=ORIENTED_EDGE('',*,*,#9327,.F.);
#13649=ORIENTED_EDGE('',*,*,#9499,.F.);
#13650=ORIENTED_EDGE('',*,*,#9500,.F.);
#13651=ORIENTED_EDGE('',*,*,#9501,.F.);
#13652=ORIENTED_EDGE('',*,*,#9328,.F.);
#13653=ORIENTED_EDGE('',*,*,#9498,.F.);
#13654=ORIENTED_EDGE('',*,*,#9502,.F.);
#13655=ORIENTED_EDGE('',*,*,#9503,.T.);
#13656=ORIENTED_EDGE('',*,*,#9333,.F.);
#13657=ORIENTED_EDGE('',*,*,#9504,.F.);
#13658=ORIENTED_EDGE('',*,*,#9505,.F.);
#13659=ORIENTED_EDGE('',*,*,#9506,.F.);
#13660=ORIENTED_EDGE('',*,*,#9334,.F.);
#13661=ORIENTED_EDGE('',*,*,#9503,.F.);
#13662=ORIENTED_EDGE('',*,*,#9507,.F.);
#13663=ORIENTED_EDGE('',*,*,#9508,.T.);
#13664=ORIENTED_EDGE('',*,*,#9339,.F.);
#13665=ORIENTED_EDGE('',*,*,#9509,.F.);
#13666=ORIENTED_EDGE('',*,*,#9510,.F.);
#13667=ORIENTED_EDGE('',*,*,#9511,.F.);
#13668=ORIENTED_EDGE('',*,*,#9340,.F.);
#13669=ORIENTED_EDGE('',*,*,#9508,.F.);
#13670=ORIENTED_EDGE('',*,*,#9512,.F.);
#13671=ORIENTED_EDGE('',*,*,#9513,.T.);
#13672=ORIENTED_EDGE('',*,*,#9345,.F.);
#13673=ORIENTED_EDGE('',*,*,#9514,.F.);
#13674=ORIENTED_EDGE('',*,*,#9515,.F.);
#13675=ORIENTED_EDGE('',*,*,#9516,.F.);
#13676=ORIENTED_EDGE('',*,*,#9346,.F.);
#13677=ORIENTED_EDGE('',*,*,#9513,.F.);
#13678=ORIENTED_EDGE('',*,*,#9517,.F.);
#13679=ORIENTED_EDGE('',*,*,#9518,.T.);
#13680=ORIENTED_EDGE('',*,*,#9351,.F.);
#13681=ORIENTED_EDGE('',*,*,#9519,.F.);
#13682=ORIENTED_EDGE('',*,*,#9520,.F.);
#13683=ORIENTED_EDGE('',*,*,#9521,.F.);
#13684=ORIENTED_EDGE('',*,*,#9352,.F.);
#13685=ORIENTED_EDGE('',*,*,#9518,.F.);
#13686=ORIENTED_EDGE('',*,*,#9522,.F.);
#13687=ORIENTED_EDGE('',*,*,#9523,.T.);
#13688=ORIENTED_EDGE('',*,*,#9357,.F.);
#13689=ORIENTED_EDGE('',*,*,#9524,.F.);
#13690=ORIENTED_EDGE('',*,*,#9525,.F.);
#13691=ORIENTED_EDGE('',*,*,#9526,.F.);
#13692=ORIENTED_EDGE('',*,*,#9358,.F.);
#13693=ORIENTED_EDGE('',*,*,#9523,.F.);
#13694=ORIENTED_EDGE('',*,*,#9527,.F.);
#13695=ORIENTED_EDGE('',*,*,#9528,.T.);
#13696=ORIENTED_EDGE('',*,*,#9363,.F.);
#13697=ORIENTED_EDGE('',*,*,#9529,.F.);
#13698=ORIENTED_EDGE('',*,*,#9530,.F.);
#13699=ORIENTED_EDGE('',*,*,#9531,.F.);
#13700=ORIENTED_EDGE('',*,*,#9364,.F.);
#13701=ORIENTED_EDGE('',*,*,#9528,.F.);
#13702=ORIENTED_EDGE('',*,*,#9532,.F.);
#13703=ORIENTED_EDGE('',*,*,#9533,.T.);
#13704=ORIENTED_EDGE('',*,*,#9369,.F.);
#13705=ORIENTED_EDGE('',*,*,#9534,.F.);
#13706=ORIENTED_EDGE('',*,*,#9535,.F.);
#13707=ORIENTED_EDGE('',*,*,#9536,.F.);
#13708=ORIENTED_EDGE('',*,*,#9370,.F.);
#13709=ORIENTED_EDGE('',*,*,#9533,.F.);
#13710=ORIENTED_EDGE('',*,*,#9537,.F.);
#13711=ORIENTED_EDGE('',*,*,#9538,.T.);
#13712=ORIENTED_EDGE('',*,*,#9375,.F.);
#13713=ORIENTED_EDGE('',*,*,#9539,.F.);
#13714=ORIENTED_EDGE('',*,*,#9540,.F.);
#13715=ORIENTED_EDGE('',*,*,#9541,.F.);
#13716=ORIENTED_EDGE('',*,*,#9376,.F.);
#13717=ORIENTED_EDGE('',*,*,#9538,.F.);
#13718=ORIENTED_EDGE('',*,*,#9542,.F.);
#13719=ORIENTED_EDGE('',*,*,#9543,.T.);
#13720=ORIENTED_EDGE('',*,*,#9378,.F.);
#13721=ORIENTED_EDGE('',*,*,#9544,.F.);
#13722=ORIENTED_EDGE('',*,*,#9545,.F.);
#13723=ORIENTED_EDGE('',*,*,#9546,.F.);
#13724=ORIENTED_EDGE('',*,*,#9379,.F.);
#13725=ORIENTED_EDGE('',*,*,#9543,.F.);
#13726=ORIENTED_EDGE('',*,*,#9547,.F.);
#13727=ORIENTED_EDGE('',*,*,#9548,.T.);
#13728=ORIENTED_EDGE('',*,*,#9384,.F.);
#13729=ORIENTED_EDGE('',*,*,#9549,.F.);
#13730=ORIENTED_EDGE('',*,*,#9550,.F.);
#13731=ORIENTED_EDGE('',*,*,#9551,.F.);
#13732=ORIENTED_EDGE('',*,*,#9385,.F.);
#13733=ORIENTED_EDGE('',*,*,#9548,.F.);
#13734=ORIENTED_EDGE('',*,*,#9552,.F.);
#13735=ORIENTED_EDGE('',*,*,#9553,.T.);
#13736=ORIENTED_EDGE('',*,*,#9390,.F.);
#13737=ORIENTED_EDGE('',*,*,#9554,.F.);
#13738=ORIENTED_EDGE('',*,*,#9555,.F.);
#13739=ORIENTED_EDGE('',*,*,#9556,.F.);
#13740=ORIENTED_EDGE('',*,*,#9391,.F.);
#13741=ORIENTED_EDGE('',*,*,#9553,.F.);
#13742=ORIENTED_EDGE('',*,*,#9557,.F.);
#13743=ORIENTED_EDGE('',*,*,#9558,.T.);
#13744=ORIENTED_EDGE('',*,*,#9396,.F.);
#13745=ORIENTED_EDGE('',*,*,#9559,.F.);
#13746=ORIENTED_EDGE('',*,*,#9560,.F.);
#13747=ORIENTED_EDGE('',*,*,#9561,.F.);
#13748=ORIENTED_EDGE('',*,*,#9397,.F.);
#13749=ORIENTED_EDGE('',*,*,#9558,.F.);
#13750=ORIENTED_EDGE('',*,*,#9562,.F.);
#13751=ORIENTED_EDGE('',*,*,#9563,.T.);
#13752=ORIENTED_EDGE('',*,*,#9402,.F.);
#13753=ORIENTED_EDGE('',*,*,#9564,.F.);
#13754=ORIENTED_EDGE('',*,*,#9565,.F.);
#13755=ORIENTED_EDGE('',*,*,#9566,.F.);
#13756=ORIENTED_EDGE('',*,*,#9403,.F.);
#13757=ORIENTED_EDGE('',*,*,#9563,.F.);
#13758=ORIENTED_EDGE('',*,*,#9567,.F.);
#13759=ORIENTED_EDGE('',*,*,#9568,.T.);
#13760=ORIENTED_EDGE('',*,*,#9408,.F.);
#13761=ORIENTED_EDGE('',*,*,#9569,.F.);
#13762=ORIENTED_EDGE('',*,*,#9570,.F.);
#13763=ORIENTED_EDGE('',*,*,#9571,.F.);
#13764=ORIENTED_EDGE('',*,*,#9409,.F.);
#13765=ORIENTED_EDGE('',*,*,#9568,.F.);
#13766=ORIENTED_EDGE('',*,*,#9572,.F.);
#13767=ORIENTED_EDGE('',*,*,#9573,.T.);
#13768=ORIENTED_EDGE('',*,*,#9414,.F.);
#13769=ORIENTED_EDGE('',*,*,#9574,.F.);
#13770=ORIENTED_EDGE('',*,*,#9575,.F.);
#13771=ORIENTED_EDGE('',*,*,#9576,.F.);
#13772=ORIENTED_EDGE('',*,*,#9415,.F.);
#13773=ORIENTED_EDGE('',*,*,#9573,.F.);
#13774=ORIENTED_EDGE('',*,*,#9577,.F.);
#13775=ORIENTED_EDGE('',*,*,#9578,.T.);
#13776=ORIENTED_EDGE('',*,*,#9420,.F.);
#13777=ORIENTED_EDGE('',*,*,#9579,.F.);
#13778=ORIENTED_EDGE('',*,*,#9580,.F.);
#13779=ORIENTED_EDGE('',*,*,#9581,.F.);
#13780=ORIENTED_EDGE('',*,*,#9421,.F.);
#13781=ORIENTED_EDGE('',*,*,#9578,.F.);
#13782=ORIENTED_EDGE('',*,*,#9582,.F.);
#13783=ORIENTED_EDGE('',*,*,#9583,.T.);
#13784=ORIENTED_EDGE('',*,*,#9426,.F.);
#13785=ORIENTED_EDGE('',*,*,#9584,.F.);
#13786=ORIENTED_EDGE('',*,*,#9585,.F.);
#13787=ORIENTED_EDGE('',*,*,#9586,.F.);
#13788=ORIENTED_EDGE('',*,*,#9427,.F.);
#13789=ORIENTED_EDGE('',*,*,#9583,.F.);
#13790=ORIENTED_EDGE('',*,*,#9587,.F.);
#13791=ORIENTED_EDGE('',*,*,#9588,.T.);
#13792=ORIENTED_EDGE('',*,*,#9423,.F.);
#13793=ORIENTED_EDGE('',*,*,#9589,.F.);
#13794=ORIENTED_EDGE('',*,*,#9590,.F.);
#13795=ORIENTED_EDGE('',*,*,#9591,.F.);
#13796=ORIENTED_EDGE('',*,*,#9424,.F.);
#13797=ORIENTED_EDGE('',*,*,#9588,.F.);
#13798=ORIENTED_EDGE('',*,*,#9592,.F.);
#13799=ORIENTED_EDGE('',*,*,#9593,.T.);
#13800=ORIENTED_EDGE('',*,*,#9417,.F.);
#13801=ORIENTED_EDGE('',*,*,#9594,.F.);
#13802=ORIENTED_EDGE('',*,*,#9595,.F.);
#13803=ORIENTED_EDGE('',*,*,#9596,.F.);
#13804=ORIENTED_EDGE('',*,*,#9418,.F.);
#13805=ORIENTED_EDGE('',*,*,#9593,.F.);
#13806=ORIENTED_EDGE('',*,*,#9597,.F.);
#13807=ORIENTED_EDGE('',*,*,#9598,.T.);
#13808=ORIENTED_EDGE('',*,*,#9411,.F.);
#13809=ORIENTED_EDGE('',*,*,#9599,.F.);
#13810=ORIENTED_EDGE('',*,*,#9600,.F.);
#13811=ORIENTED_EDGE('',*,*,#9601,.F.);
#13812=ORIENTED_EDGE('',*,*,#9412,.F.);
#13813=ORIENTED_EDGE('',*,*,#9598,.F.);
#13814=ORIENTED_EDGE('',*,*,#9602,.F.);
#13815=ORIENTED_EDGE('',*,*,#9603,.T.);
#13816=ORIENTED_EDGE('',*,*,#9405,.F.);
#13817=ORIENTED_EDGE('',*,*,#9604,.F.);
#13818=ORIENTED_EDGE('',*,*,#9605,.F.);
#13819=ORIENTED_EDGE('',*,*,#9606,.F.);
#13820=ORIENTED_EDGE('',*,*,#9406,.F.);
#13821=ORIENTED_EDGE('',*,*,#9603,.F.);
#13822=ORIENTED_EDGE('',*,*,#9607,.F.);
#13823=ORIENTED_EDGE('',*,*,#9608,.T.);
#13824=ORIENTED_EDGE('',*,*,#9399,.F.);
#13825=ORIENTED_EDGE('',*,*,#9609,.F.);
#13826=ORIENTED_EDGE('',*,*,#9610,.F.);
#13827=ORIENTED_EDGE('',*,*,#9611,.F.);
#13828=ORIENTED_EDGE('',*,*,#9400,.F.);
#13829=ORIENTED_EDGE('',*,*,#9608,.F.);
#13830=ORIENTED_EDGE('',*,*,#9612,.F.);
#13831=ORIENTED_EDGE('',*,*,#9613,.T.);
#13832=ORIENTED_EDGE('',*,*,#9393,.F.);
#13833=ORIENTED_EDGE('',*,*,#9614,.F.);
#13834=ORIENTED_EDGE('',*,*,#9615,.F.);
#13835=ORIENTED_EDGE('',*,*,#9616,.F.);
#13836=ORIENTED_EDGE('',*,*,#9394,.F.);
#13837=ORIENTED_EDGE('',*,*,#9613,.F.);
#13838=ORIENTED_EDGE('',*,*,#9617,.F.);
#13839=ORIENTED_EDGE('',*,*,#9618,.T.);
#13840=ORIENTED_EDGE('',*,*,#9387,.F.);
#13841=ORIENTED_EDGE('',*,*,#9619,.F.);
#13842=ORIENTED_EDGE('',*,*,#9620,.F.);
#13843=ORIENTED_EDGE('',*,*,#9621,.F.);
#13844=ORIENTED_EDGE('',*,*,#9388,.F.);
#13845=ORIENTED_EDGE('',*,*,#9618,.F.);
#13846=ORIENTED_EDGE('',*,*,#9622,.F.);
#13847=ORIENTED_EDGE('',*,*,#9623,.T.);
#13848=ORIENTED_EDGE('',*,*,#9381,.F.);
#13849=ORIENTED_EDGE('',*,*,#9624,.F.);
#13850=ORIENTED_EDGE('',*,*,#9625,.F.);
#13851=ORIENTED_EDGE('',*,*,#9626,.F.);
#13852=ORIENTED_EDGE('',*,*,#9382,.F.);
#13853=ORIENTED_EDGE('',*,*,#9623,.F.);
#13854=ORIENTED_EDGE('',*,*,#9627,.F.);
#13855=ORIENTED_EDGE('',*,*,#9628,.T.);
#13856=ORIENTED_EDGE('',*,*,#9429,.F.);
#13857=ORIENTED_EDGE('',*,*,#9629,.F.);
#13858=ORIENTED_EDGE('',*,*,#9630,.F.);
#13859=ORIENTED_EDGE('',*,*,#9631,.F.);
#13860=ORIENTED_EDGE('',*,*,#9430,.F.);
#13861=ORIENTED_EDGE('',*,*,#9628,.F.);
#13862=ORIENTED_EDGE('',*,*,#9632,.F.);
#13863=ORIENTED_EDGE('',*,*,#9633,.T.);
#13864=ORIENTED_EDGE('',*,*,#9372,.F.);
#13865=ORIENTED_EDGE('',*,*,#9634,.F.);
#13866=ORIENTED_EDGE('',*,*,#9635,.F.);
#13867=ORIENTED_EDGE('',*,*,#9636,.F.);
#13868=ORIENTED_EDGE('',*,*,#9373,.F.);
#13869=ORIENTED_EDGE('',*,*,#9633,.F.);
#13870=ORIENTED_EDGE('',*,*,#9637,.F.);
#13871=ORIENTED_EDGE('',*,*,#9638,.T.);
#13872=ORIENTED_EDGE('',*,*,#9366,.F.);
#13873=ORIENTED_EDGE('',*,*,#9639,.F.);
#13874=ORIENTED_EDGE('',*,*,#9640,.F.);
#13875=ORIENTED_EDGE('',*,*,#9641,.F.);
#13876=ORIENTED_EDGE('',*,*,#9367,.F.);
#13877=ORIENTED_EDGE('',*,*,#9638,.F.);
#13878=ORIENTED_EDGE('',*,*,#9642,.F.);
#13879=ORIENTED_EDGE('',*,*,#9643,.T.);
#13880=ORIENTED_EDGE('',*,*,#9360,.F.);
#13881=ORIENTED_EDGE('',*,*,#9644,.F.);
#13882=ORIENTED_EDGE('',*,*,#9645,.F.);
#13883=ORIENTED_EDGE('',*,*,#9646,.F.);
#13884=ORIENTED_EDGE('',*,*,#9361,.F.);
#13885=ORIENTED_EDGE('',*,*,#9643,.F.);
#13886=ORIENTED_EDGE('',*,*,#9647,.F.);
#13887=ORIENTED_EDGE('',*,*,#9648,.T.);
#13888=ORIENTED_EDGE('',*,*,#9354,.F.);
#13889=ORIENTED_EDGE('',*,*,#9649,.F.);
#13890=ORIENTED_EDGE('',*,*,#9650,.F.);
#13891=ORIENTED_EDGE('',*,*,#9651,.F.);
#13892=ORIENTED_EDGE('',*,*,#9355,.F.);
#13893=ORIENTED_EDGE('',*,*,#9648,.F.);
#13894=ORIENTED_EDGE('',*,*,#9652,.F.);
#13895=ORIENTED_EDGE('',*,*,#9653,.T.);
#13896=ORIENTED_EDGE('',*,*,#9348,.F.);
#13897=ORIENTED_EDGE('',*,*,#9654,.F.);
#13898=ORIENTED_EDGE('',*,*,#9655,.F.);
#13899=ORIENTED_EDGE('',*,*,#9656,.F.);
#13900=ORIENTED_EDGE('',*,*,#9349,.F.);
#13901=ORIENTED_EDGE('',*,*,#9653,.F.);
#13902=ORIENTED_EDGE('',*,*,#9657,.F.);
#13903=ORIENTED_EDGE('',*,*,#9658,.T.);
#13904=ORIENTED_EDGE('',*,*,#9342,.F.);
#13905=ORIENTED_EDGE('',*,*,#9659,.F.);
#13906=ORIENTED_EDGE('',*,*,#9660,.F.);
#13907=ORIENTED_EDGE('',*,*,#9661,.F.);
#13908=ORIENTED_EDGE('',*,*,#9343,.F.);
#13909=ORIENTED_EDGE('',*,*,#9658,.F.);
#13910=ORIENTED_EDGE('',*,*,#9662,.F.);
#13911=ORIENTED_EDGE('',*,*,#9663,.T.);
#13912=ORIENTED_EDGE('',*,*,#9336,.F.);
#13913=ORIENTED_EDGE('',*,*,#9664,.F.);
#13914=ORIENTED_EDGE('',*,*,#9665,.F.);
#13915=ORIENTED_EDGE('',*,*,#9666,.F.);
#13916=ORIENTED_EDGE('',*,*,#9337,.F.);
#13917=ORIENTED_EDGE('',*,*,#9663,.F.);
#13918=ORIENTED_EDGE('',*,*,#9667,.F.);
#13919=ORIENTED_EDGE('',*,*,#9668,.T.);
#13920=ORIENTED_EDGE('',*,*,#9330,.F.);
#13921=ORIENTED_EDGE('',*,*,#9669,.F.);
#13922=ORIENTED_EDGE('',*,*,#9670,.F.);
#13923=ORIENTED_EDGE('',*,*,#9671,.F.);
#13924=ORIENTED_EDGE('',*,*,#9331,.F.);
#13925=ORIENTED_EDGE('',*,*,#9668,.F.);
#13926=ORIENTED_EDGE('',*,*,#9672,.F.);
#13927=ORIENTED_EDGE('',*,*,#9673,.T.);
#13928=ORIENTED_EDGE('',*,*,#9432,.F.);
#13929=ORIENTED_EDGE('',*,*,#9674,.F.);
#13930=ORIENTED_EDGE('',*,*,#9675,.F.);
#13931=ORIENTED_EDGE('',*,*,#9676,.F.);
#13932=ORIENTED_EDGE('',*,*,#9433,.F.);
#13933=ORIENTED_EDGE('',*,*,#9673,.F.);
#13934=ORIENTED_EDGE('',*,*,#9631,.T.);
#13935=ORIENTED_EDGE('',*,*,#9677,.F.);
#13936=ORIENTED_EDGE('',*,*,#9674,.T.);
#13937=ORIENTED_EDGE('',*,*,#9431,.T.);
#13938=ORIENTED_EDGE('',*,*,#9586,.T.);
#13939=ORIENTED_EDGE('',*,*,#9678,.F.);
#13940=ORIENTED_EDGE('',*,*,#9629,.T.);
#13941=ORIENTED_EDGE('',*,*,#9428,.T.);
#13942=ORIENTED_EDGE('',*,*,#9584,.T.);
#13943=ORIENTED_EDGE('',*,*,#9425,.T.);
#13944=ORIENTED_EDGE('',*,*,#9591,.T.);
#13945=ORIENTED_EDGE('',*,*,#9679,.F.);
#13946=ORIENTED_EDGE('',*,*,#9581,.T.);
#13947=ORIENTED_EDGE('',*,*,#9680,.F.);
#13948=ORIENTED_EDGE('',*,*,#9589,.T.);
#13949=ORIENTED_EDGE('',*,*,#9422,.T.);
#13950=ORIENTED_EDGE('',*,*,#9579,.T.);
#13951=ORIENTED_EDGE('',*,*,#9419,.T.);
#13952=ORIENTED_EDGE('',*,*,#9596,.T.);
#13953=ORIENTED_EDGE('',*,*,#9681,.F.);
#13954=ORIENTED_EDGE('',*,*,#9576,.T.);
#13955=ORIENTED_EDGE('',*,*,#9682,.F.);
#13956=ORIENTED_EDGE('',*,*,#9594,.T.);
#13957=ORIENTED_EDGE('',*,*,#9416,.T.);
#13958=ORIENTED_EDGE('',*,*,#9574,.T.);
#13959=ORIENTED_EDGE('',*,*,#9413,.T.);
#13960=ORIENTED_EDGE('',*,*,#9601,.T.);
#13961=ORIENTED_EDGE('',*,*,#9683,.F.);
#13962=ORIENTED_EDGE('',*,*,#9571,.T.);
#13963=ORIENTED_EDGE('',*,*,#9684,.F.);
#13964=ORIENTED_EDGE('',*,*,#9599,.T.);
#13965=ORIENTED_EDGE('',*,*,#9410,.T.);
#13966=ORIENTED_EDGE('',*,*,#9569,.T.);
#13967=ORIENTED_EDGE('',*,*,#9407,.T.);
#13968=ORIENTED_EDGE('',*,*,#9606,.T.);
#13969=ORIENTED_EDGE('',*,*,#9685,.F.);
#13970=ORIENTED_EDGE('',*,*,#9566,.T.);
#13971=ORIENTED_EDGE('',*,*,#9686,.F.);
#13972=ORIENTED_EDGE('',*,*,#9604,.T.);
#13973=ORIENTED_EDGE('',*,*,#9404,.T.);
#13974=ORIENTED_EDGE('',*,*,#9564,.T.);
#13975=ORIENTED_EDGE('',*,*,#9401,.T.);
#13976=ORIENTED_EDGE('',*,*,#9611,.T.);
#13977=ORIENTED_EDGE('',*,*,#9687,.F.);
#13978=ORIENTED_EDGE('',*,*,#9561,.T.);
#13979=ORIENTED_EDGE('',*,*,#9688,.F.);
#13980=ORIENTED_EDGE('',*,*,#9609,.T.);
#13981=ORIENTED_EDGE('',*,*,#9398,.T.);
#13982=ORIENTED_EDGE('',*,*,#9559,.T.);
#13983=ORIENTED_EDGE('',*,*,#9395,.T.);
#13984=ORIENTED_EDGE('',*,*,#9616,.T.);
#13985=ORIENTED_EDGE('',*,*,#9689,.F.);
#13986=ORIENTED_EDGE('',*,*,#9556,.T.);
#13987=ORIENTED_EDGE('',*,*,#9690,.F.);
#13988=ORIENTED_EDGE('',*,*,#9614,.T.);
#13989=ORIENTED_EDGE('',*,*,#9392,.T.);
#13990=ORIENTED_EDGE('',*,*,#9554,.T.);
#13991=ORIENTED_EDGE('',*,*,#9389,.T.);
#13992=ORIENTED_EDGE('',*,*,#9621,.T.);
#13993=ORIENTED_EDGE('',*,*,#9691,.F.);
#13994=ORIENTED_EDGE('',*,*,#9551,.T.);
#13995=ORIENTED_EDGE('',*,*,#9692,.F.);
#13996=ORIENTED_EDGE('',*,*,#9619,.T.);
#13997=ORIENTED_EDGE('',*,*,#9386,.T.);
#13998=ORIENTED_EDGE('',*,*,#9549,.T.);
#13999=ORIENTED_EDGE('',*,*,#9383,.T.);
#14000=ORIENTED_EDGE('',*,*,#9626,.T.);
#14001=ORIENTED_EDGE('',*,*,#9693,.F.);
#14002=ORIENTED_EDGE('',*,*,#9546,.T.);
#14003=ORIENTED_EDGE('',*,*,#9694,.F.);
#14004=ORIENTED_EDGE('',*,*,#9624,.T.);
#14005=ORIENTED_EDGE('',*,*,#9380,.T.);
#14006=ORIENTED_EDGE('',*,*,#9541,.T.);
#14007=ORIENTED_EDGE('',*,*,#9695,.F.);
#14008=ORIENTED_EDGE('',*,*,#9544,.T.);
#14009=ORIENTED_EDGE('',*,*,#9377,.T.);
#14010=ORIENTED_EDGE('',*,*,#9539,.T.);
#14011=ORIENTED_EDGE('',*,*,#9374,.T.);
#14012=ORIENTED_EDGE('',*,*,#9636,.T.);
#14013=ORIENTED_EDGE('',*,*,#9696,.F.);
#14014=ORIENTED_EDGE('',*,*,#9536,.T.);
#14015=ORIENTED_EDGE('',*,*,#9697,.F.);
#14016=ORIENTED_EDGE('',*,*,#9634,.T.);
#14017=ORIENTED_EDGE('',*,*,#9371,.T.);
#14018=ORIENTED_EDGE('',*,*,#9534,.T.);
#14019=ORIENTED_EDGE('',*,*,#9368,.T.);
#14020=ORIENTED_EDGE('',*,*,#9641,.T.);
#14021=ORIENTED_EDGE('',*,*,#9698,.F.);
#14022=ORIENTED_EDGE('',*,*,#9531,.T.);
#14023=ORIENTED_EDGE('',*,*,#9699,.F.);
#14024=ORIENTED_EDGE('',*,*,#9639,.T.);
#14025=ORIENTED_EDGE('',*,*,#9365,.T.);
#14026=ORIENTED_EDGE('',*,*,#9529,.T.);
#14027=ORIENTED_EDGE('',*,*,#9362,.T.);
#14028=ORIENTED_EDGE('',*,*,#9646,.T.);
#14029=ORIENTED_EDGE('',*,*,#9700,.F.);
#14030=ORIENTED_EDGE('',*,*,#9526,.T.);
#14031=ORIENTED_EDGE('',*,*,#9701,.F.);
#14032=ORIENTED_EDGE('',*,*,#9644,.T.);
#14033=ORIENTED_EDGE('',*,*,#9359,.T.);
#14034=ORIENTED_EDGE('',*,*,#9524,.T.);
#14035=ORIENTED_EDGE('',*,*,#9356,.T.);
#14036=ORIENTED_EDGE('',*,*,#9651,.T.);
#14037=ORIENTED_EDGE('',*,*,#9702,.F.);
#14038=ORIENTED_EDGE('',*,*,#9521,.T.);
#14039=ORIENTED_EDGE('',*,*,#9703,.F.);
#14040=ORIENTED_EDGE('',*,*,#9649,.T.);
#14041=ORIENTED_EDGE('',*,*,#9353,.T.);
#14042=ORIENTED_EDGE('',*,*,#9519,.T.);
#14043=ORIENTED_EDGE('',*,*,#9350,.T.);
#14044=ORIENTED_EDGE('',*,*,#9656,.T.);
#14045=ORIENTED_EDGE('',*,*,#9704,.F.);
#14046=ORIENTED_EDGE('',*,*,#9516,.T.);
#14047=ORIENTED_EDGE('',*,*,#9705,.F.);
#14048=ORIENTED_EDGE('',*,*,#9654,.T.);
#14049=ORIENTED_EDGE('',*,*,#9347,.T.);
#14050=ORIENTED_EDGE('',*,*,#9514,.T.);
#14051=ORIENTED_EDGE('',*,*,#9344,.T.);
#14052=ORIENTED_EDGE('',*,*,#9661,.T.);
#14053=ORIENTED_EDGE('',*,*,#9706,.F.);
#14054=ORIENTED_EDGE('',*,*,#9511,.T.);
#14055=ORIENTED_EDGE('',*,*,#9707,.F.);
#14056=ORIENTED_EDGE('',*,*,#9659,.T.);
#14057=ORIENTED_EDGE('',*,*,#9341,.T.);
#14058=ORIENTED_EDGE('',*,*,#9509,.T.);
#14059=ORIENTED_EDGE('',*,*,#9338,.T.);
#14060=ORIENTED_EDGE('',*,*,#9666,.T.);
#14061=ORIENTED_EDGE('',*,*,#9708,.F.);
#14062=ORIENTED_EDGE('',*,*,#9506,.T.);
#14063=ORIENTED_EDGE('',*,*,#9709,.F.);
#14064=ORIENTED_EDGE('',*,*,#9664,.T.);
#14065=ORIENTED_EDGE('',*,*,#9335,.T.);
#14066=ORIENTED_EDGE('',*,*,#9504,.T.);
#14067=ORIENTED_EDGE('',*,*,#9332,.T.);
#14068=ORIENTED_EDGE('',*,*,#9671,.T.);
#14069=ORIENTED_EDGE('',*,*,#9710,.F.);
#14070=ORIENTED_EDGE('',*,*,#9501,.T.);
#14071=ORIENTED_EDGE('',*,*,#9711,.F.);
#14072=ORIENTED_EDGE('',*,*,#9669,.T.);
#14073=ORIENTED_EDGE('',*,*,#9329,.T.);
#14074=ORIENTED_EDGE('',*,*,#9499,.T.);
#14075=ORIENTED_EDGE('',*,*,#9434,.T.);
#14076=ORIENTED_EDGE('',*,*,#9676,.T.);
#14077=ORIENTED_EDGE('',*,*,#9712,.F.);
#14078=ORIENTED_EDGE('',*,*,#9713,.F.);
#14079=ORIENTED_EDGE('',*,*,#9318,.F.);
#14080=ORIENTED_EDGE('',*,*,#9179,.F.);
#14081=ORIENTED_EDGE('',*,*,#9319,.F.);
#14082=ORIENTED_EDGE('',*,*,#9714,.T.);
#14083=ORIENTED_EDGE('',*,*,#9713,.T.);
#14084=ORIENTED_EDGE('',*,*,#9714,.F.);
#14085=ORIENTED_EDGE('',*,*,#9715,.F.);
#14086=ORIENTED_EDGE('',*,*,#9716,.T.);
#14087=ORIENTED_EDGE('',*,*,#9537,.T.);
#14088=ORIENTED_EDGE('',*,*,#9696,.T.);
#14089=ORIENTED_EDGE('',*,*,#9635,.T.);
#14090=ORIENTED_EDGE('',*,*,#9632,.T.);
#14091=ORIENTED_EDGE('',*,*,#9697,.T.);
#14092=ORIENTED_EDGE('',*,*,#9535,.T.);
#14093=ORIENTED_EDGE('',*,*,#9532,.T.);
#14094=ORIENTED_EDGE('',*,*,#9698,.T.);
#14095=ORIENTED_EDGE('',*,*,#9640,.T.);
#14096=ORIENTED_EDGE('',*,*,#9637,.T.);
#14097=ORIENTED_EDGE('',*,*,#9699,.T.);
#14098=ORIENTED_EDGE('',*,*,#9530,.T.);
#14099=ORIENTED_EDGE('',*,*,#9527,.T.);
#14100=ORIENTED_EDGE('',*,*,#9700,.T.);
#14101=ORIENTED_EDGE('',*,*,#9645,.T.);
#14102=ORIENTED_EDGE('',*,*,#9642,.T.);
#14103=ORIENTED_EDGE('',*,*,#9701,.T.);
#14104=ORIENTED_EDGE('',*,*,#9525,.T.);
#14105=ORIENTED_EDGE('',*,*,#9522,.T.);
#14106=ORIENTED_EDGE('',*,*,#9702,.T.);
#14107=ORIENTED_EDGE('',*,*,#9650,.T.);
#14108=ORIENTED_EDGE('',*,*,#9647,.T.);
#14109=ORIENTED_EDGE('',*,*,#9703,.T.);
#14110=ORIENTED_EDGE('',*,*,#9520,.T.);
#14111=ORIENTED_EDGE('',*,*,#9517,.T.);
#14112=ORIENTED_EDGE('',*,*,#9704,.T.);
#14113=ORIENTED_EDGE('',*,*,#9655,.T.);
#14114=ORIENTED_EDGE('',*,*,#9652,.T.);
#14115=ORIENTED_EDGE('',*,*,#9705,.T.);
#14116=ORIENTED_EDGE('',*,*,#9515,.T.);
#14117=ORIENTED_EDGE('',*,*,#9512,.T.);
#14118=ORIENTED_EDGE('',*,*,#9706,.T.);
#14119=ORIENTED_EDGE('',*,*,#9660,.T.);
#14120=ORIENTED_EDGE('',*,*,#9657,.T.);
#14121=ORIENTED_EDGE('',*,*,#9707,.T.);
#14122=ORIENTED_EDGE('',*,*,#9510,.T.);
#14123=ORIENTED_EDGE('',*,*,#9507,.T.);
#14124=ORIENTED_EDGE('',*,*,#9708,.T.);
#14125=ORIENTED_EDGE('',*,*,#9665,.T.);
#14126=ORIENTED_EDGE('',*,*,#9662,.T.);
#14127=ORIENTED_EDGE('',*,*,#9709,.T.);
#14128=ORIENTED_EDGE('',*,*,#9505,.T.);
#14129=ORIENTED_EDGE('',*,*,#9502,.T.);
#14130=ORIENTED_EDGE('',*,*,#9710,.T.);
#14131=ORIENTED_EDGE('',*,*,#9670,.T.);
#14132=ORIENTED_EDGE('',*,*,#9667,.T.);
#14133=ORIENTED_EDGE('',*,*,#9711,.T.);
#14134=ORIENTED_EDGE('',*,*,#9500,.T.);
#14135=ORIENTED_EDGE('',*,*,#9497,.T.);
#14136=ORIENTED_EDGE('',*,*,#9712,.T.);
#14137=ORIENTED_EDGE('',*,*,#9675,.T.);
#14138=ORIENTED_EDGE('',*,*,#9672,.T.);
#14139=ORIENTED_EDGE('',*,*,#9677,.T.);
#14140=ORIENTED_EDGE('',*,*,#9630,.T.);
#14141=ORIENTED_EDGE('',*,*,#9627,.T.);
#14142=ORIENTED_EDGE('',*,*,#9678,.T.);
#14143=ORIENTED_EDGE('',*,*,#9585,.T.);
#14144=ORIENTED_EDGE('',*,*,#9582,.T.);
#14145=ORIENTED_EDGE('',*,*,#9679,.T.);
#14146=ORIENTED_EDGE('',*,*,#9590,.T.);
#14147=ORIENTED_EDGE('',*,*,#9587,.T.);
#14148=ORIENTED_EDGE('',*,*,#9680,.T.);
#14149=ORIENTED_EDGE('',*,*,#9580,.T.);
#14150=ORIENTED_EDGE('',*,*,#9577,.T.);
#14151=ORIENTED_EDGE('',*,*,#9681,.T.);
#14152=ORIENTED_EDGE('',*,*,#9595,.T.);
#14153=ORIENTED_EDGE('',*,*,#9592,.T.);
#14154=ORIENTED_EDGE('',*,*,#9682,.T.);
#14155=ORIENTED_EDGE('',*,*,#9575,.T.);
#14156=ORIENTED_EDGE('',*,*,#9572,.T.);
#14157=ORIENTED_EDGE('',*,*,#9683,.T.);
#14158=ORIENTED_EDGE('',*,*,#9600,.T.);
#14159=ORIENTED_EDGE('',*,*,#9597,.T.);
#14160=ORIENTED_EDGE('',*,*,#9684,.T.);
#14161=ORIENTED_EDGE('',*,*,#9570,.T.);
#14162=ORIENTED_EDGE('',*,*,#9567,.T.);
#14163=ORIENTED_EDGE('',*,*,#9685,.T.);
#14164=ORIENTED_EDGE('',*,*,#9605,.T.);
#14165=ORIENTED_EDGE('',*,*,#9602,.T.);
#14166=ORIENTED_EDGE('',*,*,#9686,.T.);
#14167=ORIENTED_EDGE('',*,*,#9565,.T.);
#14168=ORIENTED_EDGE('',*,*,#9562,.T.);
#14169=ORIENTED_EDGE('',*,*,#9687,.T.);
#14170=ORIENTED_EDGE('',*,*,#9610,.T.);
#14171=ORIENTED_EDGE('',*,*,#9607,.T.);
#14172=ORIENTED_EDGE('',*,*,#9688,.T.);
#14173=ORIENTED_EDGE('',*,*,#9560,.T.);
#14174=ORIENTED_EDGE('',*,*,#9557,.T.);
#14175=ORIENTED_EDGE('',*,*,#9689,.T.);
#14176=ORIENTED_EDGE('',*,*,#9615,.T.);
#14177=ORIENTED_EDGE('',*,*,#9612,.T.);
#14178=ORIENTED_EDGE('',*,*,#9690,.T.);
#14179=ORIENTED_EDGE('',*,*,#9555,.T.);
#14180=ORIENTED_EDGE('',*,*,#9552,.T.);
#14181=ORIENTED_EDGE('',*,*,#9691,.T.);
#14182=ORIENTED_EDGE('',*,*,#9620,.T.);
#14183=ORIENTED_EDGE('',*,*,#9617,.T.);
#14184=ORIENTED_EDGE('',*,*,#9692,.T.);
#14185=ORIENTED_EDGE('',*,*,#9550,.T.);
#14186=ORIENTED_EDGE('',*,*,#9547,.T.);
#14187=ORIENTED_EDGE('',*,*,#9693,.T.);
#14188=ORIENTED_EDGE('',*,*,#9625,.T.);
#14189=ORIENTED_EDGE('',*,*,#9622,.T.);
#14190=ORIENTED_EDGE('',*,*,#9694,.T.);
#14191=ORIENTED_EDGE('',*,*,#9545,.T.);
#14192=ORIENTED_EDGE('',*,*,#9542,.T.);
#14193=ORIENTED_EDGE('',*,*,#9695,.T.);
#14194=ORIENTED_EDGE('',*,*,#9540,.T.);
#14195=ORIENTED_EDGE('',*,*,#9716,.F.);
#14196=ORIENTED_EDGE('',*,*,#9715,.T.);
#14197=ORIENTED_EDGE('',*,*,#9483,.T.);
#14198=ORIENTED_EDGE('',*,*,#9494,.T.);
#14199=ORIENTED_EDGE('',*,*,#9496,.T.);
#14200=ORIENTED_EDGE('',*,*,#9478,.T.);
#14201=ORIENTED_EDGE('',*,*,#9468,.T.);
#14202=ORIENTED_EDGE('',*,*,#9473,.T.);
#15158=PLANE('',#17379);
#15159=PLANE('',#17382);
#15160=PLANE('',#17392);
#15161=PLANE('',#17429);
#15162=PLANE('',#17431);
#15163=PLANE('',#17433);
#15164=PLANE('',#17435);
#15165=PLANE('',#17437);
#15166=PLANE('',#17439);
#15167=PLANE('',#17449);
#15168=PLANE('',#17450);
#15169=PLANE('',#17451);
#15170=PLANE('',#17452);
#15171=PLANE('',#17453);
#15172=PLANE('',#17454);
#15173=PLANE('',#17455);
#15174=PLANE('',#17456);
#15175=PLANE('',#17457);
#15176=PLANE('',#17458);
#15177=PLANE('',#17459);
#15178=PLANE('',#17460);
#15179=PLANE('',#17461);
#15180=PLANE('',#17462);
#15181=PLANE('',#17463);
#15182=PLANE('',#17464);
#15183=PLANE('',#17465);
#15184=PLANE('',#17466);
#15185=PLANE('',#17467);
#15186=PLANE('',#17468);
#15187=PLANE('',#17469);
#15188=PLANE('',#17470);
#15189=PLANE('',#17471);
#15190=PLANE('',#17472);
#15191=PLANE('',#17473);
#15192=PLANE('',#17474);
#15193=PLANE('',#17475);
#15194=PLANE('',#17476);
#15195=PLANE('',#17477);
#15196=PLANE('',#17478);
#15197=PLANE('',#17479);
#15198=PLANE('',#17480);
#15199=PLANE('',#17481);
#15200=PLANE('',#17482);
#15201=PLANE('',#17483);
#15202=PLANE('',#17484);
#15203=PLANE('',#17485);
#15204=PLANE('',#17486);
#15205=PLANE('',#17487);
#15206=PLANE('',#17488);
#15207=PLANE('',#17489);
#15208=PLANE('',#17490);
#15209=PLANE('',#17491);
#15210=PLANE('',#17492);
#15211=PLANE('',#17493);
#15212=PLANE('',#17494);
#15213=PLANE('',#17495);
#15214=PLANE('',#17496);
#15215=PLANE('',#17497);
#15216=PLANE('',#17498);
#15217=PLANE('',#17499);
#15218=PLANE('',#17500);
#15219=PLANE('',#17501);
#15220=PLANE('',#17502);
#15221=PLANE('',#17503);
#15222=PLANE('',#17504);
#15223=PLANE('',#17505);
#15224=PLANE('',#17506);
#15225=PLANE('',#17507);
#15226=PLANE('',#17508);
#15227=PLANE('',#17509);
#15228=PLANE('',#17510);
#15229=PLANE('',#17511);
#15230=PLANE('',#17512);
#15231=PLANE('',#17513);
#15232=PLANE('',#17514);
#15233=PLANE('',#17515);
#15234=PLANE('',#17516);
#15235=PLANE('',#17517);
#15236=PLANE('',#17518);
#15237=PLANE('',#17519);
#15238=PLANE('',#17520);
#15239=PLANE('',#17521);
#15240=PLANE('',#17522);
#15241=PLANE('',#17523);
#15242=PLANE('',#17524);
#15243=PLANE('',#17525);
#15244=PLANE('',#17526);
#15245=PLANE('',#17527);
#15246=PLANE('',#17528);
#15247=PLANE('',#17529);
#15248=PLANE('',#17530);
#15249=PLANE('',#17531);
#15250=PLANE('',#17532);
#15251=PLANE('',#17533);
#15252=PLANE('',#17534);
#15253=PLANE('',#17535);
#15254=PLANE('',#17536);
#15255=PLANE('',#17537);
#15256=PLANE('',#17538);
#15257=PLANE('',#17539);
#15258=PLANE('',#17540);
#15259=PLANE('',#17541);
#15260=PLANE('',#17542);
#15261=PLANE('',#17543);
#15262=PLANE('',#17544);
#15263=PLANE('',#17617);
#15264=PLANE('',#17622);
#15934=ADVANCED_FACE('',(#2391),#1029,.T.);
#15935=ADVANCED_FACE('',(#2392),#1030,.T.);
#15936=ADVANCED_FACE('',(#2393),#1031,.T.);
#15937=ADVANCED_FACE('',(#2394),#1032,.T.);
#15938=ADVANCED_FACE('',(#2395),#1033,.T.);
#15939=ADVANCED_FACE('',(#2396),#1034,.T.);
#15940=ADVANCED_FACE('',(#2397),#1035,.T.);
#15941=ADVANCED_FACE('',(#2398),#1036,.T.);
#15942=ADVANCED_FACE('',(#2399),#1037,.T.);
#15943=ADVANCED_FACE('',(#2400),#1038,.T.);
#15944=ADVANCED_FACE('',(#2401),#1039,.T.);
#15945=ADVANCED_FACE('',(#2402),#1040,.T.);
#15946=ADVANCED_FACE('',(#2403),#1041,.T.);
#15947=ADVANCED_FACE('',(#2404),#1042,.T.);
#15948=ADVANCED_FACE('',(#2405),#1043,.T.);
#15949=ADVANCED_FACE('',(#2406),#1044,.T.);
#15950=ADVANCED_FACE('',(#2407),#1045,.T.);
#15951=ADVANCED_FACE('',(#2408),#1046,.T.);
#15952=ADVANCED_FACE('',(#2409),#1047,.T.);
#15953=ADVANCED_FACE('',(#2410),#1048,.T.);
#15954=ADVANCED_FACE('',(#2411),#1049,.T.);
#15955=ADVANCED_FACE('',(#2412),#1050,.T.);
#15956=ADVANCED_FACE('',(#2413),#1051,.T.);
#15957=ADVANCED_FACE('',(#2414),#1052,.T.);
#15958=ADVANCED_FACE('',(#2415),#1053,.T.);
#15959=ADVANCED_FACE('',(#2416),#1054,.T.);
#15960=ADVANCED_FACE('',(#2417),#1055,.T.);
#15961=ADVANCED_FACE('',(#2418),#1056,.T.);
#15962=ADVANCED_FACE('',(#2419),#1057,.T.);
#15963=ADVANCED_FACE('',(#2420),#1058,.T.);
#15964=ADVANCED_FACE('',(#2421),#1059,.T.);
#15965=ADVANCED_FACE('',(#2422),#1060,.T.);
#15966=ADVANCED_FACE('',(#2423),#1061,.T.);
#15967=ADVANCED_FACE('',(#2424),#1062,.T.);
#15968=ADVANCED_FACE('',(#2425),#1063,.T.);
#15969=ADVANCED_FACE('',(#2426),#1064,.T.);
#15970=ADVANCED_FACE('',(#2427),#1065,.T.);
#15971=ADVANCED_FACE('',(#2428),#1066,.T.);
#15972=ADVANCED_FACE('',(#2429),#1067,.T.);
#15973=ADVANCED_FACE('',(#2430),#1068,.T.);
#15974=ADVANCED_FACE('',(#2431),#1069,.T.);
#15975=ADVANCED_FACE('',(#2432),#1070,.T.);
#15976=ADVANCED_FACE('',(#2433),#1071,.T.);
#15977=ADVANCED_FACE('',(#2434),#1072,.T.);
#15978=ADVANCED_FACE('',(#2435),#15158,.F.);
#15979=ADVANCED_FACE('',(#2436),#506,.F.);
#15980=ADVANCED_FACE('',(#2437),#15159,.T.);
#15981=ADVANCED_FACE('',(#2438),#1073,.T.);
#15982=ADVANCED_FACE('',(#2439),#507,.F.);
#15983=ADVANCED_FACE('',(#2440),#489,.F.);
#15984=ADVANCED_FACE('',(#2441),#1074,.T.);
#15985=ADVANCED_FACE('',(#2442,#1202),#15160,.T.);
#15986=ADVANCED_FACE('',(#2443),#15161,.F.);
#15987=ADVANCED_FACE('',(#2444),#15162,.F.);
#15988=ADVANCED_FACE('',(#2445),#15163,.F.);
#15989=ADVANCED_FACE('',(#2446),#15164,.F.);
#15990=ADVANCED_FACE('',(#2447),#15165,.F.);
#15991=ADVANCED_FACE('',(#2448),#15166,.F.);
#15992=ADVANCED_FACE('',(#2449),#1768,.F.);
#15993=ADVANCED_FACE('',(#2450),#15167,.F.);
#15994=ADVANCED_FACE('',(#2451),#15168,.F.);
#15995=ADVANCED_FACE('',(#2452),#15169,.F.);
#15996=ADVANCED_FACE('',(#2453),#15170,.F.);
#15997=ADVANCED_FACE('',(#2454),#15171,.F.);
#15998=ADVANCED_FACE('',(#2455),#15172,.F.);
#15999=ADVANCED_FACE('',(#2456),#15173,.F.);
#16000=ADVANCED_FACE('',(#2457),#15174,.F.);
#16001=ADVANCED_FACE('',(#2458),#15175,.F.);
#16002=ADVANCED_FACE('',(#2459),#15176,.F.);
#16003=ADVANCED_FACE('',(#2460),#15177,.F.);
#16004=ADVANCED_FACE('',(#2461),#15178,.F.);
#16005=ADVANCED_FACE('',(#2462),#15179,.F.);
#16006=ADVANCED_FACE('',(#2463),#15180,.F.);
#16007=ADVANCED_FACE('',(#2464),#15181,.F.);
#16008=ADVANCED_FACE('',(#2465),#15182,.F.);
#16009=ADVANCED_FACE('',(#2466),#15183,.F.);
#16010=ADVANCED_FACE('',(#2467),#15184,.F.);
#16011=ADVANCED_FACE('',(#2468),#15185,.F.);
#16012=ADVANCED_FACE('',(#2469),#15186,.F.);
#16013=ADVANCED_FACE('',(#2470),#15187,.F.);
#16014=ADVANCED_FACE('',(#2471),#15188,.F.);
#16015=ADVANCED_FACE('',(#2472),#15189,.F.);
#16016=ADVANCED_FACE('',(#2473),#15190,.F.);
#16017=ADVANCED_FACE('',(#2474),#15191,.F.);
#16018=ADVANCED_FACE('',(#2475),#15192,.F.);
#16019=ADVANCED_FACE('',(#2476),#15193,.F.);
#16020=ADVANCED_FACE('',(#2477),#15194,.F.);
#16021=ADVANCED_FACE('',(#2478),#15195,.F.);
#16022=ADVANCED_FACE('',(#2479),#15196,.F.);
#16023=ADVANCED_FACE('',(#2480),#15197,.F.);
#16024=ADVANCED_FACE('',(#2481),#15198,.F.);
#16025=ADVANCED_FACE('',(#2482),#15199,.F.);
#16026=ADVANCED_FACE('',(#2483),#15200,.F.);
#16027=ADVANCED_FACE('',(#2484),#15201,.F.);
#16028=ADVANCED_FACE('',(#2485),#15202,.F.);
#16029=ADVANCED_FACE('',(#2486),#15203,.F.);
#16030=ADVANCED_FACE('',(#2487),#15204,.F.);
#16031=ADVANCED_FACE('',(#2488),#15205,.F.);
#16032=ADVANCED_FACE('',(#2489),#15206,.F.);
#16033=ADVANCED_FACE('',(#2490),#15207,.F.);
#16034=ADVANCED_FACE('',(#2491),#15208,.F.);
#16035=ADVANCED_FACE('',(#2492),#15209,.F.);
#16036=ADVANCED_FACE('',(#2493),#15210,.F.);
#16037=ADVANCED_FACE('',(#2494),#15211,.F.);
#16038=ADVANCED_FACE('',(#2495),#15212,.F.);
#16039=ADVANCED_FACE('',(#2496),#15213,.F.);
#16040=ADVANCED_FACE('',(#2497),#15214,.F.);
#16041=ADVANCED_FACE('',(#2498),#15215,.F.);
#16042=ADVANCED_FACE('',(#2499),#15216,.F.);
#16043=ADVANCED_FACE('',(#2500),#15217,.F.);
#16044=ADVANCED_FACE('',(#2501),#15218,.F.);
#16045=ADVANCED_FACE('',(#2502),#15219,.F.);
#16046=ADVANCED_FACE('',(#2503),#15220,.F.);
#16047=ADVANCED_FACE('',(#2504),#15221,.F.);
#16048=ADVANCED_FACE('',(#2505),#15222,.F.);
#16049=ADVANCED_FACE('',(#2506),#15223,.F.);
#16050=ADVANCED_FACE('',(#2507),#15224,.F.);
#16051=ADVANCED_FACE('',(#2508),#15225,.F.);
#16052=ADVANCED_FACE('',(#2509),#15226,.F.);
#16053=ADVANCED_FACE('',(#2510),#15227,.F.);
#16054=ADVANCED_FACE('',(#2511),#15228,.F.);
#16055=ADVANCED_FACE('',(#2512),#15229,.F.);
#16056=ADVANCED_FACE('',(#2513),#15230,.F.);
#16057=ADVANCED_FACE('',(#2514),#15231,.F.);
#16058=ADVANCED_FACE('',(#2515),#15232,.F.);
#16059=ADVANCED_FACE('',(#2516),#15233,.F.);
#16060=ADVANCED_FACE('',(#2517),#15234,.F.);
#16061=ADVANCED_FACE('',(#2518),#15235,.F.);
#16062=ADVANCED_FACE('',(#2519),#15236,.F.);
#16063=ADVANCED_FACE('',(#2520),#15237,.F.);
#16064=ADVANCED_FACE('',(#2521),#15238,.F.);
#16065=ADVANCED_FACE('',(#2522),#15239,.F.);
#16066=ADVANCED_FACE('',(#2523),#15240,.F.);
#16067=ADVANCED_FACE('',(#2524),#15241,.F.);
#16068=ADVANCED_FACE('',(#2525),#15242,.F.);
#16069=ADVANCED_FACE('',(#2526),#15243,.F.);
#16070=ADVANCED_FACE('',(#2527),#15244,.F.);
#16071=ADVANCED_FACE('',(#2528),#15245,.F.);
#16072=ADVANCED_FACE('',(#2529),#15246,.F.);
#16073=ADVANCED_FACE('',(#2530),#15247,.F.);
#16074=ADVANCED_FACE('',(#2531),#15248,.F.);
#16075=ADVANCED_FACE('',(#2532),#15249,.F.);
#16076=ADVANCED_FACE('',(#2533),#15250,.F.);
#16077=ADVANCED_FACE('',(#2534),#15251,.F.);
#16078=ADVANCED_FACE('',(#2535),#15252,.F.);
#16079=ADVANCED_FACE('',(#2536),#15253,.F.);
#16080=ADVANCED_FACE('',(#2537),#15254,.F.);
#16081=ADVANCED_FACE('',(#2538),#15255,.F.);
#16082=ADVANCED_FACE('',(#2539),#15256,.F.);
#16083=ADVANCED_FACE('',(#2540),#15257,.F.);
#16084=ADVANCED_FACE('',(#2541),#15258,.F.);
#16085=ADVANCED_FACE('',(#2542),#15259,.F.);
#16086=ADVANCED_FACE('',(#2543),#15260,.F.);
#16087=ADVANCED_FACE('',(#2544),#15261,.F.);
#16088=ADVANCED_FACE('',(#2545),#15262,.F.);
#16089=ADVANCED_FACE('',(#2546),#1075,.T.);
#16090=ADVANCED_FACE('',(#2547),#1076,.T.);
#16091=ADVANCED_FACE('',(#2548),#1077,.T.);
#16092=ADVANCED_FACE('',(#2549),#1078,.T.);
#16093=ADVANCED_FACE('',(#2550),#1079,.T.);
#16094=ADVANCED_FACE('',(#2551),#1080,.T.);
#16095=ADVANCED_FACE('',(#2552),#1081,.T.);
#16096=ADVANCED_FACE('',(#2553),#1082,.T.);
#16097=ADVANCED_FACE('',(#2554),#1083,.T.);
#16098=ADVANCED_FACE('',(#2555),#1084,.T.);
#16099=ADVANCED_FACE('',(#2556),#1085,.T.);
#16100=ADVANCED_FACE('',(#2557),#1086,.T.);
#16101=ADVANCED_FACE('',(#2558),#1087,.T.);
#16102=ADVANCED_FACE('',(#2559),#1088,.T.);
#16103=ADVANCED_FACE('',(#2560),#1089,.T.);
#16104=ADVANCED_FACE('',(#2561),#1090,.T.);
#16105=ADVANCED_FACE('',(#2562),#1091,.T.);
#16106=ADVANCED_FACE('',(#2563),#1092,.T.);
#16107=ADVANCED_FACE('',(#2564),#1093,.T.);
#16108=ADVANCED_FACE('',(#2565),#1094,.T.);
#16109=ADVANCED_FACE('',(#2566),#1095,.T.);
#16110=ADVANCED_FACE('',(#2567),#1096,.T.);
#16111=ADVANCED_FACE('',(#2568),#1097,.T.);
#16112=ADVANCED_FACE('',(#2569),#1098,.T.);
#16113=ADVANCED_FACE('',(#2570),#1099,.T.);
#16114=ADVANCED_FACE('',(#2571),#1100,.T.);
#16115=ADVANCED_FACE('',(#2572),#1101,.T.);
#16116=ADVANCED_FACE('',(#2573),#1102,.T.);
#16117=ADVANCED_FACE('',(#2574),#1103,.T.);
#16118=ADVANCED_FACE('',(#2575),#1104,.T.);
#16119=ADVANCED_FACE('',(#2576),#1105,.T.);
#16120=ADVANCED_FACE('',(#2577),#1106,.T.);
#16121=ADVANCED_FACE('',(#2578),#1107,.T.);
#16122=ADVANCED_FACE('',(#2579),#1108,.T.);
#16123=ADVANCED_FACE('',(#2580),#1109,.T.);
#16124=ADVANCED_FACE('',(#2581),#1110,.T.);
#16125=ADVANCED_FACE('',(#2582),#15263,.T.);
#16126=ADVANCED_FACE('',(#2583),#1769,.T.);
#16127=ADVANCED_FACE('',(#2584),#1770,.T.);
#16128=ADVANCED_FACE('',(#2585,#1203),#15264,.T.);
#16246=CLOSED_SHELL('',(#15934,#15935,#15936,#15937,#15938,#15939,#15940,
#15941,#15942,#15943,#15944,#15945,#15946,#15947,#15948,#15949,#15950,#15951,
#15952,#15953,#15954,#15955,#15956,#15957,#15958,#15959,#15960,#15961,#15962,
#15963,#15964,#15965,#15966,#15967,#15968,#15969,#15970,#15971,#15972,#15973,
#15974,#15975,#15976,#15977,#15978,#15979,#15980,#15981,#15982,#15983,#15984,
#15985,#15986,#15987,#15988,#15989,#15990,#15991,#15992,#15993,#15994,#15995,
#15996,#15997,#15998,#15999,#16000,#16001,#16002,#16003,#16004,#16005,#16006,
#16007,#16008,#16009,#16010,#16011,#16012,#16013,#16014,#16015,#16016,#16017,
#16018,#16019,#16020,#16021,#16022,#16023,#16024,#16025,#16026,#16027,#16028,
#16029,#16030,#16031,#16032,#16033,#16034,#16035,#16036,#16037,#16038,#16039,
#16040,#16041,#16042,#16043,#16044,#16045,#16046,#16047,#16048,#16049,#16050,
#16051,#16052,#16053,#16054,#16055,#16056,#16057,#16058,#16059,#16060,#16061,
#16062,#16063,#16064,#16065,#16066,#16067,#16068,#16069,#16070,#16071,#16072,
#16073,#16074,#16075,#16076,#16077,#16078,#16079,#16080,#16081,#16082,#16083,
#16084,#16085,#16086,#16087,#16088,#16089,#16090,#16091,#16092,#16093,#16094,
#16095,#16096,#16097,#16098,#16099,#16100,#16101,#16102,#16103,#16104,#16105,
#16106,#16107,#16108,#16109,#16110,#16111,#16112,#16113,#16114,#16115,#16116,
#16117,#16118,#16119,#16120,#16121,#16122,#16123,#16124,#16125,#16126,#16127,
#16128));
#17332=AXIS2_PLACEMENT_3D('',#32268,#20527,#20528);
#17333=AXIS2_PLACEMENT_3D('',#32269,#20529,#20530);
#17334=AXIS2_PLACEMENT_3D('',#32285,#20532,#20533);
#17335=AXIS2_PLACEMENT_3D('',#32293,#20534,#20535);
#17336=AXIS2_PLACEMENT_3D('',#32341,#20537,#20538);
#17337=AXIS2_PLACEMENT_3D('',#32389,#20540,#20541);
#17338=AXIS2_PLACEMENT_3D('',#32440,#20543,#20544);
#17339=AXIS2_PLACEMENT_3D('',#32491,#20546,#20547);
#17340=AXIS2_PLACEMENT_3D('',#32539,#20549,#20550);
#17341=AXIS2_PLACEMENT_3D('',#32587,#20552,#20553);
#17342=AXIS2_PLACEMENT_3D('',#32641,#20555,#20556);
#17343=AXIS2_PLACEMENT_3D('',#32689,#20558,#20559);
#17344=AXIS2_PLACEMENT_3D('',#32737,#20561,#20562);
#17345=AXIS2_PLACEMENT_3D('',#32791,#20564,#20565);
#17346=AXIS2_PLACEMENT_3D('',#32839,#20567,#20568);
#17347=AXIS2_PLACEMENT_3D('',#32887,#20570,#20571);
#17348=AXIS2_PLACEMENT_3D('',#32935,#20573,#20574);
#17349=AXIS2_PLACEMENT_3D('',#32989,#20576,#20577);
#17350=AXIS2_PLACEMENT_3D('',#33037,#20579,#20580);
#17351=AXIS2_PLACEMENT_3D('',#33085,#20582,#20583);
#17352=AXIS2_PLACEMENT_3D('',#33139,#20585,#20586);
#17353=AXIS2_PLACEMENT_3D('',#33187,#20588,#20589);
#17354=AXIS2_PLACEMENT_3D('',#33235,#20591,#20592);
#17355=AXIS2_PLACEMENT_3D('',#33289,#20594,#20595);
#17356=AXIS2_PLACEMENT_3D('',#33337,#20597,#20598);
#17357=AXIS2_PLACEMENT_3D('',#33349,#20600,#20601);
#17358=AXIS2_PLACEMENT_3D('',#33355,#20602,#20603);
#17359=AXIS2_PLACEMENT_3D('',#33379,#20605,#20606);
#17360=AXIS2_PLACEMENT_3D('',#33404,#20608,#20609);
#17361=AXIS2_PLACEMENT_3D('',#33429,#20611,#20612);
#17362=AXIS2_PLACEMENT_3D('',#33453,#20614,#20615);
#17363=AXIS2_PLACEMENT_3D('',#33478,#20617,#20618);
#17364=AXIS2_PLACEMENT_3D('',#33503,#20620,#20621);
#17365=AXIS2_PLACEMENT_3D('',#33527,#20623,#20624);
#17366=AXIS2_PLACEMENT_3D('',#33552,#20626,#20627);
#17367=AXIS2_PLACEMENT_3D('',#33577,#20629,#20630);
#17368=AXIS2_PLACEMENT_3D('',#33601,#20632,#20633);
#17369=AXIS2_PLACEMENT_3D('',#33625,#20635,#20636);
#17370=AXIS2_PLACEMENT_3D('',#33650,#20638,#20639);
#17371=AXIS2_PLACEMENT_3D('',#33675,#20641,#20642);
#17372=AXIS2_PLACEMENT_3D('',#33699,#20644,#20645);
#17373=AXIS2_PLACEMENT_3D('',#33724,#20647,#20648);
#17374=AXIS2_PLACEMENT_3D('',#33749,#20650,#20651);
#17375=AXIS2_PLACEMENT_3D('',#33773,#20653,#20654);
#17376=AXIS2_PLACEMENT_3D('',#33798,#20656,#20657);
#17377=AXIS2_PLACEMENT_3D('',#33822,#20659,#20660);
#17378=AXIS2_PLACEMENT_3D('',#33847,#20662,#20663);
#17379=AXIS2_PLACEMENT_3D('',#33871,#20665,#20666);
#17380=AXIS2_PLACEMENT_3D('',#33926,#20667,#20668);
#17381=AXIS2_PLACEMENT_3D('',#33928,#20669,#20670);
#17382=AXIS2_PLACEMENT_3D('',#34638,#20671,#20672);
#17383=AXIS2_PLACEMENT_3D('',#34640,#20673,#20674);
#17384=AXIS2_PLACEMENT_3D('',#34641,#20675,#20676);
#17385=AXIS2_PLACEMENT_3D('',#34695,#20677,#20678);
#17386=AXIS2_PLACEMENT_3D('',#34696,#20679,#20680);
#17387=AXIS2_PLACEMENT_3D('',#35297,#20681,#20682);
#17388=AXIS2_PLACEMENT_3D('',#35299,#20683,#20684);
#17389=AXIS2_PLACEMENT_3D('',#35300,#20685,#20686);
#17390=AXIS2_PLACEMENT_3D('',#35301,#20687,#20688);
#17391=AXIS2_PLACEMENT_3D('',#35302,#20689,#20690);
#17392=AXIS2_PLACEMENT_3D('',#35303,#20691,#20692);
#17393=AXIS2_PLACEMENT_3D('',#35310,#20695,#20696);
#17394=AXIS2_PLACEMENT_3D('',#35316,#20699,#20700);
#17395=AXIS2_PLACEMENT_3D('',#35322,#20703,#20704);
#17396=AXIS2_PLACEMENT_3D('',#35328,#20707,#20708);
#17397=AXIS2_PLACEMENT_3D('',#35334,#20711,#20712);
#17398=AXIS2_PLACEMENT_3D('',#35340,#20715,#20716);
#17399=AXIS2_PLACEMENT_3D('',#35346,#20719,#20720);
#17400=AXIS2_PLACEMENT_3D('',#35352,#20723,#20724);
#17401=AXIS2_PLACEMENT_3D('',#35358,#20727,#20728);
#17402=AXIS2_PLACEMENT_3D('',#35364,#20731,#20732);
#17403=AXIS2_PLACEMENT_3D('',#35370,#20735,#20736);
#17404=AXIS2_PLACEMENT_3D('',#35376,#20739,#20740);
#17405=AXIS2_PLACEMENT_3D('',#35382,#20743,#20744);
#17406=AXIS2_PLACEMENT_3D('',#35388,#20747,#20748);
#17407=AXIS2_PLACEMENT_3D('',#35394,#20751,#20752);
#17408=AXIS2_PLACEMENT_3D('',#35400,#20755,#20756);
#17409=AXIS2_PLACEMENT_3D('',#35406,#20759,#20760);
#17410=AXIS2_PLACEMENT_3D('',#35412,#20763,#20764);
#17411=AXIS2_PLACEMENT_3D('',#35418,#20767,#20768);
#17412=AXIS2_PLACEMENT_3D('',#35424,#20771,#20772);
#17413=AXIS2_PLACEMENT_3D('',#35430,#20775,#20776);
#17414=AXIS2_PLACEMENT_3D('',#35436,#20779,#20780);
#17415=AXIS2_PLACEMENT_3D('',#35442,#20783,#20784);
#17416=AXIS2_PLACEMENT_3D('',#35448,#20787,#20788);
#17417=AXIS2_PLACEMENT_3D('',#35454,#20791,#20792);
#17418=AXIS2_PLACEMENT_3D('',#35460,#20795,#20796);
#17419=AXIS2_PLACEMENT_3D('',#35466,#20799,#20800);
#17420=AXIS2_PLACEMENT_3D('',#35472,#20803,#20804);
#17421=AXIS2_PLACEMENT_3D('',#35478,#20807,#20808);
#17422=AXIS2_PLACEMENT_3D('',#35484,#20811,#20812);
#17423=AXIS2_PLACEMENT_3D('',#35490,#20815,#20816);
#17424=AXIS2_PLACEMENT_3D('',#35496,#20819,#20820);
#17425=AXIS2_PLACEMENT_3D('',#35502,#20823,#20824);
#17426=AXIS2_PLACEMENT_3D('',#35508,#20827,#20828);
#17427=AXIS2_PLACEMENT_3D('',#35514,#20831,#20832);
#17428=AXIS2_PLACEMENT_3D('',#35519,#20835,#20836);
#17429=AXIS2_PLACEMENT_3D('',#35520,#20837,#20838);
#17430=AXIS2_PLACEMENT_3D('',#35524,#20840,#20841);
#17431=AXIS2_PLACEMENT_3D('',#35525,#20842,#20843);
#17432=AXIS2_PLACEMENT_3D('',#35528,#20845,#20846);
#17433=AXIS2_PLACEMENT_3D('',#35529,#20847,#20848);
#17434=AXIS2_PLACEMENT_3D('',#35532,#20850,#20851);
#17435=AXIS2_PLACEMENT_3D('',#35533,#20852,#20853);
#17436=AXIS2_PLACEMENT_3D('',#35536,#20855,#20856);
#17437=AXIS2_PLACEMENT_3D('',#35537,#20857,#20858);
#17438=AXIS2_PLACEMENT_3D('',#35540,#20860,#20861);
#17439=AXIS2_PLACEMENT_3D('',#35541,#20862,#20863);
#17440=AXIS2_PLACEMENT_3D('',#35543,#20865,#20866);
#17441=AXIS2_PLACEMENT_3D('',#35544,#20867,#20868);
#17442=AXIS2_PLACEMENT_3D('',#35549,#20870,#20871);
#17443=AXIS2_PLACEMENT_3D('',#35558,#20872,#20873);
#17444=AXIS2_PLACEMENT_3D('',#35567,#20874,#20875);
#17445=AXIS2_PLACEMENT_3D('',#35576,#20876,#20877);
#17446=AXIS2_PLACEMENT_3D('',#35585,#20878,#20879);
#17447=AXIS2_PLACEMENT_3D('',#35594,#20880,#20881);
#17448=AXIS2_PLACEMENT_3D('',#35602,#20882,#20883);
#17449=AXIS2_PLACEMENT_3D('',#35603,#20884,#20885);
#17450=AXIS2_PLACEMENT_3D('',#35609,#20889,#20890);
#17451=AXIS2_PLACEMENT_3D('',#35613,#20893,#20894);
#17452=AXIS2_PLACEMENT_3D('',#35617,#20897,#20898);
#17453=AXIS2_PLACEMENT_3D('',#35621,#20901,#20902);
#17454=AXIS2_PLACEMENT_3D('',#35625,#20905,#20906);
#17455=AXIS2_PLACEMENT_3D('',#35629,#20909,#20910);
#17456=AXIS2_PLACEMENT_3D('',#35633,#20913,#20914);
#17457=AXIS2_PLACEMENT_3D('',#35637,#20917,#20918);
#17458=AXIS2_PLACEMENT_3D('',#35641,#20921,#20922);
#17459=AXIS2_PLACEMENT_3D('',#35643,#20924,#20925);
#17460=AXIS2_PLACEMENT_3D('',#35645,#20927,#20928);
#17461=AXIS2_PLACEMENT_3D('',#35646,#20929,#20930);
#17462=AXIS2_PLACEMENT_3D('',#35648,#20932,#20933);
#17463=AXIS2_PLACEMENT_3D('',#35652,#20936,#20937);
#17464=AXIS2_PLACEMENT_3D('',#35654,#20939,#20940);
#17465=AXIS2_PLACEMENT_3D('',#35656,#20942,#20943);
#17466=AXIS2_PLACEMENT_3D('',#35660,#20946,#20947);
#17467=AXIS2_PLACEMENT_3D('',#35662,#20949,#20950);
#17468=AXIS2_PLACEMENT_3D('',#35663,#20951,#20952);
#17469=AXIS2_PLACEMENT_3D('',#35664,#20953,#20954);
#17470=AXIS2_PLACEMENT_3D('',#35666,#20956,#20957);
#17471=AXIS2_PLACEMENT_3D('',#35667,#20958,#20959);
#17472=AXIS2_PLACEMENT_3D('',#35668,#20960,#20961);
#17473=AXIS2_PLACEMENT_3D('',#35669,#20962,#20963);
#17474=AXIS2_PLACEMENT_3D('',#35677,#20966,#20967);
#17475=AXIS2_PLACEMENT_3D('',#35683,#20969,#20970);
#17476=AXIS2_PLACEMENT_3D('',#35691,#20973,#20974);
#17477=AXIS2_PLACEMENT_3D('',#35697,#20976,#20977);
#17478=AXIS2_PLACEMENT_3D('',#35705,#20980,#20981);
#17479=AXIS2_PLACEMENT_3D('',#35711,#20983,#20984);
#17480=AXIS2_PLACEMENT_3D('',#35719,#20987,#20988);
#17481=AXIS2_PLACEMENT_3D('',#35725,#20990,#20991);
#17482=AXIS2_PLACEMENT_3D('',#35733,#20994,#20995);
#17483=AXIS2_PLACEMENT_3D('',#35739,#20997,#20998);
#17484=AXIS2_PLACEMENT_3D('',#35747,#21001,#21002);
#17485=AXIS2_PLACEMENT_3D('',#35753,#21004,#21005);
#17486=AXIS2_PLACEMENT_3D('',#35761,#21008,#21009);
#17487=AXIS2_PLACEMENT_3D('',#35767,#21011,#21012);
#17488=AXIS2_PLACEMENT_3D('',#35775,#21015,#21016);
#17489=AXIS2_PLACEMENT_3D('',#35781,#21018,#21019);
#17490=AXIS2_PLACEMENT_3D('',#35789,#21022,#21023);
#17491=AXIS2_PLACEMENT_3D('',#35795,#21025,#21026);
#17492=AXIS2_PLACEMENT_3D('',#35803,#21029,#21030);
#17493=AXIS2_PLACEMENT_3D('',#35809,#21032,#21033);
#17494=AXIS2_PLACEMENT_3D('',#35817,#21036,#21037);
#17495=AXIS2_PLACEMENT_3D('',#35823,#21039,#21040);
#17496=AXIS2_PLACEMENT_3D('',#35831,#21043,#21044);
#17497=AXIS2_PLACEMENT_3D('',#35837,#21046,#21047);
#17498=AXIS2_PLACEMENT_3D('',#35845,#21050,#21051);
#17499=AXIS2_PLACEMENT_3D('',#35851,#21053,#21054);
#17500=AXIS2_PLACEMENT_3D('',#35859,#21057,#21058);
#17501=AXIS2_PLACEMENT_3D('',#35865,#21060,#21061);
#17502=AXIS2_PLACEMENT_3D('',#35873,#21064,#21065);
#17503=AXIS2_PLACEMENT_3D('',#35879,#21067,#21068);
#17504=AXIS2_PLACEMENT_3D('',#35887,#21071,#21072);
#17505=AXIS2_PLACEMENT_3D('',#35893,#21074,#21075);
#17506=AXIS2_PLACEMENT_3D('',#35901,#21078,#21079);
#17507=AXIS2_PLACEMENT_3D('',#35907,#21081,#21082);
#17508=AXIS2_PLACEMENT_3D('',#35915,#21085,#21086);
#17509=AXIS2_PLACEMENT_3D('',#35921,#21088,#21089);
#17510=AXIS2_PLACEMENT_3D('',#35929,#21092,#21093);
#17511=AXIS2_PLACEMENT_3D('',#35935,#21095,#21096);
#17512=AXIS2_PLACEMENT_3D('',#35943,#21099,#21100);
#17513=AXIS2_PLACEMENT_3D('',#35949,#21102,#21103);
#17514=AXIS2_PLACEMENT_3D('',#35957,#21106,#21107);
#17515=AXIS2_PLACEMENT_3D('',#35963,#21109,#21110);
#17516=AXIS2_PLACEMENT_3D('',#35971,#21113,#21114);
#17517=AXIS2_PLACEMENT_3D('',#35977,#21116,#21117);
#17518=AXIS2_PLACEMENT_3D('',#35985,#21120,#21121);
#17519=AXIS2_PLACEMENT_3D('',#35991,#21123,#21124);
#17520=AXIS2_PLACEMENT_3D('',#35999,#21127,#21128);
#17521=AXIS2_PLACEMENT_3D('',#36005,#21130,#21131);
#17522=AXIS2_PLACEMENT_3D('',#36013,#21134,#21135);
#17523=AXIS2_PLACEMENT_3D('',#36019,#21137,#21138);
#17524=AXIS2_PLACEMENT_3D('',#36027,#21141,#21142);
#17525=AXIS2_PLACEMENT_3D('',#36033,#21144,#21145);
#17526=AXIS2_PLACEMENT_3D('',#36041,#21148,#21149);
#17527=AXIS2_PLACEMENT_3D('',#36047,#21151,#21152);
#17528=AXIS2_PLACEMENT_3D('',#36055,#21155,#21156);
#17529=AXIS2_PLACEMENT_3D('',#36061,#21158,#21159);
#17530=AXIS2_PLACEMENT_3D('',#36069,#21162,#21163);
#17531=AXIS2_PLACEMENT_3D('',#36075,#21165,#21166);
#17532=AXIS2_PLACEMENT_3D('',#36083,#21169,#21170);
#17533=AXIS2_PLACEMENT_3D('',#36089,#21172,#21173);
#17534=AXIS2_PLACEMENT_3D('',#36097,#21176,#21177);
#17535=AXIS2_PLACEMENT_3D('',#36103,#21179,#21180);
#17536=AXIS2_PLACEMENT_3D('',#36111,#21183,#21184);
#17537=AXIS2_PLACEMENT_3D('',#36117,#21186,#21187);
#17538=AXIS2_PLACEMENT_3D('',#36125,#21190,#21191);
#17539=AXIS2_PLACEMENT_3D('',#36131,#21193,#21194);
#17540=AXIS2_PLACEMENT_3D('',#36139,#21197,#21198);
#17541=AXIS2_PLACEMENT_3D('',#36145,#21200,#21201);
#17542=AXIS2_PLACEMENT_3D('',#36153,#21204,#21205);
#17543=AXIS2_PLACEMENT_3D('',#36159,#21207,#21208);
#17544=AXIS2_PLACEMENT_3D('',#36167,#21211,#21212);
#17545=AXIS2_PLACEMENT_3D('',#36173,#21214,#21215);
#17546=AXIS2_PLACEMENT_3D('',#36174,#21216,#21217);
#17547=AXIS2_PLACEMENT_3D('',#36175,#21218,#21219);
#17548=AXIS2_PLACEMENT_3D('',#36176,#21220,#21221);
#17549=AXIS2_PLACEMENT_3D('',#36177,#21222,#21223);
#17550=AXIS2_PLACEMENT_3D('',#36178,#21224,#21225);
#17551=AXIS2_PLACEMENT_3D('',#36179,#21226,#21227);
#17552=AXIS2_PLACEMENT_3D('',#36180,#21228,#21229);
#17553=AXIS2_PLACEMENT_3D('',#36181,#21230,#21231);
#17554=AXIS2_PLACEMENT_3D('',#36182,#21232,#21233);
#17555=AXIS2_PLACEMENT_3D('',#36183,#21234,#21235);
#17556=AXIS2_PLACEMENT_3D('',#36184,#21236,#21237);
#17557=AXIS2_PLACEMENT_3D('',#36185,#21238,#21239);
#17558=AXIS2_PLACEMENT_3D('',#36186,#21240,#21241);
#17559=AXIS2_PLACEMENT_3D('',#36187,#21242,#21243);
#17560=AXIS2_PLACEMENT_3D('',#36188,#21244,#21245);
#17561=AXIS2_PLACEMENT_3D('',#36189,#21246,#21247);
#17562=AXIS2_PLACEMENT_3D('',#36190,#21248,#21249);
#17563=AXIS2_PLACEMENT_3D('',#36191,#21250,#21251);
#17564=AXIS2_PLACEMENT_3D('',#36192,#21252,#21253);
#17565=AXIS2_PLACEMENT_3D('',#36193,#21254,#21255);
#17566=AXIS2_PLACEMENT_3D('',#36194,#21256,#21257);
#17567=AXIS2_PLACEMENT_3D('',#36195,#21258,#21259);
#17568=AXIS2_PLACEMENT_3D('',#36196,#21260,#21261);
#17569=AXIS2_PLACEMENT_3D('',#36197,#21262,#21263);
#17570=AXIS2_PLACEMENT_3D('',#36198,#21264,#21265);
#17571=AXIS2_PLACEMENT_3D('',#36199,#21266,#21267);
#17572=AXIS2_PLACEMENT_3D('',#36200,#21268,#21269);
#17573=AXIS2_PLACEMENT_3D('',#36201,#21270,#21271);
#17574=AXIS2_PLACEMENT_3D('',#36202,#21272,#21273);
#17575=AXIS2_PLACEMENT_3D('',#36203,#21274,#21275);
#17576=AXIS2_PLACEMENT_3D('',#36204,#21276,#21277);
#17577=AXIS2_PLACEMENT_3D('',#36205,#21278,#21279);
#17578=AXIS2_PLACEMENT_3D('',#36206,#21280,#21281);
#17579=AXIS2_PLACEMENT_3D('',#36207,#21282,#21283);
#17580=AXIS2_PLACEMENT_3D('',#36208,#21284,#21285);
#17581=AXIS2_PLACEMENT_3D('',#36209,#21286,#21287);
#17582=AXIS2_PLACEMENT_3D('',#36210,#21288,#21289);
#17583=AXIS2_PLACEMENT_3D('',#36211,#21290,#21291);
#17584=AXIS2_PLACEMENT_3D('',#36212,#21292,#21293);
#17585=AXIS2_PLACEMENT_3D('',#36213,#21294,#21295);
#17586=AXIS2_PLACEMENT_3D('',#36214,#21296,#21297);
#17587=AXIS2_PLACEMENT_3D('',#36215,#21298,#21299);
#17588=AXIS2_PLACEMENT_3D('',#36216,#21300,#21301);
#17589=AXIS2_PLACEMENT_3D('',#36217,#21302,#21303);
#17590=AXIS2_PLACEMENT_3D('',#36218,#21304,#21305);
#17591=AXIS2_PLACEMENT_3D('',#36219,#21306,#21307);
#17592=AXIS2_PLACEMENT_3D('',#36220,#21308,#21309);
#17593=AXIS2_PLACEMENT_3D('',#36221,#21310,#21311);
#17594=AXIS2_PLACEMENT_3D('',#36222,#21312,#21313);
#17595=AXIS2_PLACEMENT_3D('',#36223,#21314,#21315);
#17596=AXIS2_PLACEMENT_3D('',#36224,#21316,#21317);
#17597=AXIS2_PLACEMENT_3D('',#36225,#21318,#21319);
#17598=AXIS2_PLACEMENT_3D('',#36226,#21320,#21321);
#17599=AXIS2_PLACEMENT_3D('',#36227,#21322,#21323);
#17600=AXIS2_PLACEMENT_3D('',#36228,#21324,#21325);
#17601=AXIS2_PLACEMENT_3D('',#36229,#21326,#21327);
#17602=AXIS2_PLACEMENT_3D('',#36230,#21328,#21329);
#17603=AXIS2_PLACEMENT_3D('',#36231,#21330,#21331);
#17604=AXIS2_PLACEMENT_3D('',#36232,#21332,#21333);
#17605=AXIS2_PLACEMENT_3D('',#36233,#21334,#21335);
#17606=AXIS2_PLACEMENT_3D('',#36234,#21336,#21337);
#17607=AXIS2_PLACEMENT_3D('',#36235,#21338,#21339);
#17608=AXIS2_PLACEMENT_3D('',#36236,#21340,#21341);
#17609=AXIS2_PLACEMENT_3D('',#36237,#21342,#21343);
#17610=AXIS2_PLACEMENT_3D('',#36238,#21344,#21345);
#17611=AXIS2_PLACEMENT_3D('',#36239,#21346,#21347);
#17612=AXIS2_PLACEMENT_3D('',#36240,#21348,#21349);
#17613=AXIS2_PLACEMENT_3D('',#36241,#21350,#21351);
#17614=AXIS2_PLACEMENT_3D('',#36242,#21352,#21353);
#17615=AXIS2_PLACEMENT_3D('',#36243,#21354,#21355);
#17616=AXIS2_PLACEMENT_3D('',#36244,#21356,#21357);
#17617=AXIS2_PLACEMENT_3D('',#36245,#21358,#21359);
#17618=AXIS2_PLACEMENT_3D('',#36247,#21360,#21361);
#17619=AXIS2_PLACEMENT_3D('',#36248,#21362,#21363);
#17620=AXIS2_PLACEMENT_3D('',#36250,#21365,#21366);
#17621=AXIS2_PLACEMENT_3D('',#36252,#21367,#21368);
#17622=AXIS2_PLACEMENT_3D('',#36254,#21370,#21371);
#20527=DIRECTION('axis',(0.,0.,1.));
#20528=DIRECTION('refdir',(1.,0.,0.));
#20529=DIRECTION('center_axis',(0.,0.,1.));
#20530=DIRECTION('ref_axis',(1.,0.,0.));
#20531=DIRECTION('',(0.,0.,-1.));
#20532=DIRECTION('center_axis',(0.,0.,1.));
#20533=DIRECTION('ref_axis',(1.,0.,0.));
#20534=DIRECTION('center_axis',(0.,0.,1.));
#20535=DIRECTION('ref_axis',(1.,0.,0.));
#20536=DIRECTION('',(0.,0.,-1.));
#20537=DIRECTION('center_axis',(0.,0.,1.));
#20538=DIRECTION('ref_axis',(1.,0.,0.));
#20539=DIRECTION('',(0.,0.,-1.));
#20540=DIRECTION('center_axis',(0.,0.,1.));
#20541=DIRECTION('ref_axis',(1.,0.,0.));
#20542=DIRECTION('',(0.,0.,-1.));
#20543=DIRECTION('center_axis',(0.,0.,1.));
#20544=DIRECTION('ref_axis',(1.,0.,0.));
#20545=DIRECTION('',(0.,0.,-1.));
#20546=DIRECTION('center_axis',(0.,0.,1.));
#20547=DIRECTION('ref_axis',(1.,0.,0.));
#20548=DIRECTION('',(0.,0.,-1.));
#20549=DIRECTION('center_axis',(0.,0.,1.));
#20550=DIRECTION('ref_axis',(1.,0.,0.));
#20551=DIRECTION('',(0.,0.,-1.));
#20552=DIRECTION('center_axis',(0.,0.,1.));
#20553=DIRECTION('ref_axis',(1.,0.,0.));
#20554=DIRECTION('',(0.,0.,-1.));
#20555=DIRECTION('center_axis',(0.,0.,1.));
#20556=DIRECTION('ref_axis',(1.,0.,0.));
#20557=DIRECTION('',(0.,0.,-1.));
#20558=DIRECTION('center_axis',(0.,0.,1.));
#20559=DIRECTION('ref_axis',(1.,0.,0.));
#20560=DIRECTION('',(0.,0.,-1.));
#20561=DIRECTION('center_axis',(0.,0.,1.));
#20562=DIRECTION('ref_axis',(1.,0.,0.));
#20563=DIRECTION('',(0.,0.,-1.));
#20564=DIRECTION('center_axis',(0.,0.,1.));
#20565=DIRECTION('ref_axis',(1.,0.,0.));
#20566=DIRECTION('',(0.,0.,-1.));
#20567=DIRECTION('center_axis',(0.,0.,1.));
#20568=DIRECTION('ref_axis',(1.,0.,0.));
#20569=DIRECTION('',(0.,0.,-1.));
#20570=DIRECTION('center_axis',(0.,0.,1.));
#20571=DIRECTION('ref_axis',(1.,0.,0.));
#20572=DIRECTION('',(0.,0.,-1.));
#20573=DIRECTION('center_axis',(0.,0.,1.));
#20574=DIRECTION('ref_axis',(1.,0.,0.));
#20575=DIRECTION('',(0.,0.,-1.));
#20576=DIRECTION('center_axis',(0.,0.,1.));
#20577=DIRECTION('ref_axis',(1.,0.,0.));
#20578=DIRECTION('',(0.,0.,-1.));
#20579=DIRECTION('center_axis',(0.,0.,1.));
#20580=DIRECTION('ref_axis',(1.,0.,0.));
#20581=DIRECTION('',(0.,0.,-1.));
#20582=DIRECTION('center_axis',(0.,0.,1.));
#20583=DIRECTION('ref_axis',(1.,0.,0.));
#20584=DIRECTION('',(0.,0.,-1.));
#20585=DIRECTION('center_axis',(0.,0.,1.));
#20586=DIRECTION('ref_axis',(1.,0.,0.));
#20587=DIRECTION('',(0.,0.,-1.));
#20588=DIRECTION('center_axis',(0.,0.,1.));
#20589=DIRECTION('ref_axis',(1.,0.,0.));
#20590=DIRECTION('',(0.,0.,-1.));
#20591=DIRECTION('center_axis',(0.,0.,1.));
#20592=DIRECTION('ref_axis',(1.,0.,0.));
#20593=DIRECTION('',(0.,0.,-1.));
#20594=DIRECTION('center_axis',(0.,0.,1.));
#20595=DIRECTION('ref_axis',(1.,0.,0.));
#20596=DIRECTION('',(0.,0.,-1.));
#20597=DIRECTION('center_axis',(0.,0.,1.));
#20598=DIRECTION('ref_axis',(-0.266010414634152,-0.963970154779787,0.));
#20599=DIRECTION('',(0.,0.,1.));
#20600=DIRECTION('center_axis',(0.,0.,1.));
#20601=DIRECTION('ref_axis',(1.,4.93993055488555E-14,0.));
#20602=DIRECTION('center_axis',(0.,0.,1.));
#20603=DIRECTION('ref_axis',(1.,4.93993055488555E-14,0.));
#20604=DIRECTION('',(0.,0.,1.));
#20605=DIRECTION('center_axis',(0.,0.,1.));
#20606=DIRECTION('ref_axis',(1.,4.93993055488555E-14,0.));
#20607=DIRECTION('',(0.,0.,1.));
#20608=DIRECTION('center_axis',(0.,0.,1.));
#20609=DIRECTION('ref_axis',(1.,4.93993055488555E-14,0.));
#20610=DIRECTION('',(0.,0.,1.));
#20611=DIRECTION('center_axis',(0.,0.,1.));
#20612=DIRECTION('ref_axis',(1.,4.93993055488555E-14,0.));
#20613=DIRECTION('',(0.,0.,1.));
#20614=DIRECTION('center_axis',(0.,0.,1.));
#20615=DIRECTION('ref_axis',(1.,4.93993055488555E-14,0.));
#20616=DIRECTION('',(0.,0.,1.));
#20617=DIRECTION('center_axis',(0.,0.,1.));
#20618=DIRECTION('ref_axis',(1.,4.93993055488555E-14,0.));
#20619=DIRECTION('',(0.,0.,1.));
#20620=DIRECTION('center_axis',(0.,0.,1.));
#20621=DIRECTION('ref_axis',(1.,4.93993055488555E-14,0.));
#20622=DIRECTION('',(0.,0.,1.));
#20623=DIRECTION('center_axis',(0.,0.,1.));
#20624=DIRECTION('ref_axis',(1.,4.93993055488555E-14,0.));
#20625=DIRECTION('',(0.,0.,1.));
#20626=DIRECTION('center_axis',(0.,0.,1.));
#20627=DIRECTION('ref_axis',(1.,4.93993055488555E-14,0.));
#20628=DIRECTION('',(0.,0.,1.));
#20629=DIRECTION('center_axis',(0.,0.,1.));
#20630=DIRECTION('ref_axis',(1.,4.93993055488555E-14,0.));
#20631=DIRECTION('',(0.,0.,1.));
#20632=DIRECTION('center_axis',(0.,0.,1.));
#20633=DIRECTION('ref_axis',(1.,4.93993055488555E-14,0.));
#20634=DIRECTION('',(0.,0.,1.));
#20635=DIRECTION('center_axis',(0.,0.,1.));
#20636=DIRECTION('ref_axis',(1.,4.93993055488555E-14,0.));
#20637=DIRECTION('',(0.,0.,1.));
#20638=DIRECTION('center_axis',(0.,0.,1.));
#20639=DIRECTION('ref_axis',(1.,4.93993055488555E-14,0.));
#20640=DIRECTION('',(0.,0.,1.));
#20641=DIRECTION('center_axis',(0.,0.,1.));
#20642=DIRECTION('ref_axis',(1.,4.93993055488555E-14,0.));
#20643=DIRECTION('',(0.,0.,1.));
#20644=DIRECTION('center_axis',(0.,0.,1.));
#20645=DIRECTION('ref_axis',(1.,4.93993055488555E-14,0.));
#20646=DIRECTION('',(0.,0.,1.));
#20647=DIRECTION('center_axis',(0.,0.,1.));
#20648=DIRECTION('ref_axis',(1.,4.93993055488555E-14,0.));
#20649=DIRECTION('',(0.,0.,1.));
#20650=DIRECTION('center_axis',(0.,0.,1.));
#20651=DIRECTION('ref_axis',(1.,4.93993055488555E-14,0.));
#20652=DIRECTION('',(0.,0.,1.));
#20653=DIRECTION('center_axis',(0.,0.,1.));
#20654=DIRECTION('ref_axis',(1.,4.93993055488555E-14,0.));
#20655=DIRECTION('',(0.,0.,1.));
#20656=DIRECTION('center_axis',(0.,0.,1.));
#20657=DIRECTION('ref_axis',(1.,4.93993055488555E-14,0.));
#20658=DIRECTION('',(0.,0.,1.));
#20659=DIRECTION('center_axis',(0.,0.,1.));
#20660=DIRECTION('ref_axis',(1.,4.93993055488555E-14,0.));
#20661=DIRECTION('',(0.,0.,1.));
#20662=DIRECTION('center_axis',(0.,0.,1.));
#20663=DIRECTION('ref_axis',(1.,4.93993055488555E-14,0.));
#20664=DIRECTION('',(0.,0.,1.));
#20665=DIRECTION('center_axis',(0.,0.,1.));
#20666=DIRECTION('ref_axis',(1.,0.,0.));
#20667=DIRECTION('center_axis',(0.,0.,1.));
#20668=DIRECTION('ref_axis',(1.,0.,0.));
#20669=DIRECTION('center_axis',(0.,0.,1.));
#20670=DIRECTION('ref_axis',(1.,0.,0.));
#20671=DIRECTION('center_axis',(0.,0.,1.));
#20672=DIRECTION('ref_axis',(1.,0.,0.));
#20673=DIRECTION('center_axis',(0.,0.,1.));
#20674=DIRECTION('ref_axis',(1.,0.,0.));
#20675=DIRECTION('center_axis',(0.,0.,1.));
#20676=DIRECTION('ref_axis',(1.,0.,0.));
#20677=DIRECTION('center_axis',(0.,0.,-1.));
#20678=DIRECTION('ref_axis',(1.,4.93993055488555E-14,0.));
#20679=DIRECTION('center_axis',(0.,0.,1.));
#20680=DIRECTION('ref_axis',(1.,4.93993055488555E-14,0.));
#20681=DIRECTION('center_axis',(0.,0.,1.));
#20682=DIRECTION('ref_axis',(1.,0.,0.));
#20683=DIRECTION('center_axis',(1.22464679914735E-16,-1.,0.));
#20684=DIRECTION('ref_axis',(-1.,-1.22464679914735E-16,0.));
#20685=DIRECTION('center_axis',(0.,0.,-1.));
#20686=DIRECTION('ref_axis',(1.,0.,0.));
#20687=DIRECTION('center_axis',(0.,0.,1.));
#20688=DIRECTION('ref_axis',(1.,0.,0.));
#20689=DIRECTION('center_axis',(0.,0.,1.));
#20690=DIRECTION('ref_axis',(0.939073012437622,-0.343717729119883,0.));
#20691=DIRECTION('center_axis',(0.,0.,-1.));
#20692=DIRECTION('ref_axis',(-1.,0.,0.));
#20693=DIRECTION('',(-0.999593826304735,-0.0284988142465338,0.));
#20694=DIRECTION('',(0.747414611328346,-0.664357884556884,0.));
#20695=DIRECTION('center_axis',(0.,0.,1.));
#20696=DIRECTION('ref_axis',(1.,0.,0.));
#20697=DIRECTION('',(-0.989356517167622,0.145511793123284,0.));
#20698=DIRECTION('',(0.620695167978805,-0.78405198070521,0.));
#20699=DIRECTION('center_axis',(0.,0.,1.));
#20700=DIRECTION('ref_axis',(1.,0.,0.));
#20701=DIRECTION('',(-0.949058110894924,0.315101098291577,0.));
#20702=DIRECTION('',(0.475116216037135,-0.879923054169258,0.));
#20703=DIRECTION('center_axis',(0.,0.,1.));
#20704=DIRECTION('ref_axis',(1.,0.,0.));
#20705=DIRECTION('',(-0.87992305416926,0.475116216037131,0.));
#20706=DIRECTION('',(0.315101098291577,-0.949058110894924,0.));
#20707=DIRECTION('center_axis',(0.,0.,1.));
#20708=DIRECTION('ref_axis',(1.,0.,0.));
#20709=DIRECTION('',(-0.78405198070521,0.620695167978805,0.));
#20710=DIRECTION('',(0.145511793123284,-0.989356517167622,0.));
#20711=DIRECTION('center_axis',(0.,0.,1.));
#20712=DIRECTION('ref_axis',(1.,0.,0.));
#20713=DIRECTION('',(-0.66435788455688,0.747414611328349,0.));
#20714=DIRECTION('',(-0.028498814246539,-0.999593826304735,0.));
#20715=DIRECTION('center_axis',(0.,0.,1.));
#20716=DIRECTION('ref_axis',(1.,0.,0.));
#20717=DIRECTION('',(-0.524477610267605,0.851424239922721,0.));
#20718=DIRECTION('',(-0.201643499566573,-0.979458982848463,0.));
#20719=DIRECTION('center_axis',(0.,0.,1.));
#20720=DIRECTION('ref_axis',(1.,0.,0.));
#20721=DIRECTION('',(-0.368661349188821,0.929563773828498,0.));
#20722=DIRECTION('',(-0.368661349188821,-0.929563773828498,0.));
#20723=DIRECTION('center_axis',(0.,0.,1.));
#20724=DIRECTION('ref_axis',(1.,0.,0.));
#20725=DIRECTION('',(-0.201643499566578,0.979458982848462,0.));
#20726=DIRECTION('',(-0.524477610267605,-0.85142423992272,0.));
#20727=DIRECTION('center_axis',(0.,0.,1.));
#20728=DIRECTION('ref_axis',(1.,0.,0.));
#20729=DIRECTION('',(-0.0284988142465341,0.999593826304735,0.));
#20730=DIRECTION('',(-0.664357884556884,-0.747414611328346,0.));
#20731=DIRECTION('center_axis',(0.,0.,1.));
#20732=DIRECTION('ref_axis',(1.,0.,0.));
#20733=DIRECTION('',(0.145511793123284,0.989356517167622,0.));
#20734=DIRECTION('',(-0.78405198070521,-0.620695167978805,0.));
#20735=DIRECTION('center_axis',(0.,0.,1.));
#20736=DIRECTION('ref_axis',(1.,0.,0.));
#20737=DIRECTION('',(0.315101098291578,0.949058110894924,0.));
#20738=DIRECTION('',(-0.879923054169259,-0.475116216037132,0.));
#20739=DIRECTION('center_axis',(0.,0.,1.));
#20740=DIRECTION('ref_axis',(1.,0.,0.));
#20741=DIRECTION('',(0.475116216037133,0.879923054169259,0.));
#20742=DIRECTION('',(-0.949058110894923,-0.315101098291581,0.));
#20743=DIRECTION('center_axis',(0.,0.,1.));
#20744=DIRECTION('ref_axis',(1.,0.,0.));
#20745=DIRECTION('',(0.620695167978803,0.784051980705211,0.));
#20746=DIRECTION('',(-0.989356517167622,-0.145511793123284,0.));
#20747=DIRECTION('center_axis',(0.,0.,1.));
#20748=DIRECTION('ref_axis',(1.,0.,0.));
#20749=DIRECTION('',(0.747414611328348,0.664357884556882,0.));
#20750=DIRECTION('',(-0.999593826304735,0.0284988142465371,0.));
#20751=DIRECTION('center_axis',(0.,0.,1.));
#20752=DIRECTION('ref_axis',(1.,0.,0.));
#20753=DIRECTION('',(0.851424239922722,0.524477610267603,0.));
#20754=DIRECTION('',(-0.979458982848462,0.201643499566578,0.));
#20755=DIRECTION('center_axis',(0.,0.,1.));
#20756=DIRECTION('ref_axis',(1.,0.,0.));
#20757=DIRECTION('',(0.929563773828499,0.368661349188818,0.));
#20758=DIRECTION('',(-0.929563773828499,0.368661349188818,0.));
#20759=DIRECTION('center_axis',(0.,0.,1.));
#20760=DIRECTION('ref_axis',(1.,0.,0.));
#20761=DIRECTION('',(0.979458982848462,0.201643499566576,0.));
#20762=DIRECTION('',(-0.85142423992272,0.524477610267605,0.));
#20763=DIRECTION('center_axis',(0.,0.,1.));
#20764=DIRECTION('ref_axis',(1.,0.,0.));
#20765=DIRECTION('',(0.999593826304735,0.0284988142465395,0.));
#20766=DIRECTION('',(-0.747414611328348,0.664357884556882,0.));
#20767=DIRECTION('center_axis',(0.,0.,1.));
#20768=DIRECTION('ref_axis',(1.,0.,0.));
#20769=DIRECTION('',(0.989356517167621,-0.145511793123287,0.));
#20770=DIRECTION('',(-0.620695167978801,0.784051980705213,0.));
#20771=DIRECTION('center_axis',(0.,0.,1.));
#20772=DIRECTION('ref_axis',(1.,0.,0.));
#20773=DIRECTION('',(0.949058110894924,-0.315101098291577,0.));
#20774=DIRECTION('',(-0.475116216037132,0.879923054169259,0.));
#20775=DIRECTION('center_axis',(0.,0.,1.));
#20776=DIRECTION('ref_axis',(1.,0.,0.));
#20777=DIRECTION('',(0.879923054169259,-0.475116216037133,0.));
#20778=DIRECTION('',(-0.31510109829158,0.949058110894923,0.));
#20779=DIRECTION('center_axis',(0.,0.,1.));
#20780=DIRECTION('ref_axis',(1.,0.,0.));
#20781=DIRECTION('',(0.784051980705213,-0.620695167978802,0.));
#20782=DIRECTION('',(-0.145511793123287,0.989356517167621,0.));
#20783=DIRECTION('center_axis',(0.,0.,1.));
#20784=DIRECTION('ref_axis',(1.,0.,0.));
#20785=DIRECTION('',(0.664357884556883,-0.747414611328346,0.));
#20786=DIRECTION('',(0.028498814246538,0.999593826304735,0.));
#20787=DIRECTION('center_axis',(0.,0.,1.));
#20788=DIRECTION('ref_axis',(1.,0.,0.));
#20789=DIRECTION('',(0.524477610267604,-0.851424239922721,0.));
#20790=DIRECTION('',(0.201643499566577,0.979458982848462,0.));
#20791=DIRECTION('center_axis',(0.,0.,1.));
#20792=DIRECTION('ref_axis',(1.,0.,0.));
#20793=DIRECTION('',(0.368661349188819,-0.929563773828498,0.));
#20794=DIRECTION('',(0.368661349188819,0.929563773828498,0.));
#20795=DIRECTION('center_axis',(0.,0.,1.));
#20796=DIRECTION('ref_axis',(1.,0.,0.));
#20797=DIRECTION('',(0.201643499566577,-0.979458982848462,0.));
#20798=DIRECTION('',(0.524477610267603,0.851424239922722,0.));
#20799=DIRECTION('center_axis',(0.,0.,1.));
#20800=DIRECTION('ref_axis',(1.,0.,0.));
#20801=DIRECTION('',(0.0284988142465383,-0.999593826304735,0.));
#20802=DIRECTION('',(0.664357884556882,0.747414611328348,0.));
#20803=DIRECTION('center_axis',(0.,0.,1.));
#20804=DIRECTION('ref_axis',(1.,0.,0.));
#20805=DIRECTION('',(-0.145511793123286,-0.989356517167621,0.));
#20806=DIRECTION('',(0.784051980705211,0.620695167978803,0.));
#20807=DIRECTION('center_axis',(0.,0.,1.));
#20808=DIRECTION('ref_axis',(1.,0.,0.));
#20809=DIRECTION('',(-0.31510109829158,-0.949058110894923,0.));
#20810=DIRECTION('',(0.879923054169259,0.475116216037132,0.));
#20811=DIRECTION('center_axis',(0.,0.,1.));
#20812=DIRECTION('ref_axis',(1.,0.,0.));
#20813=DIRECTION('',(-0.475116216037132,-0.87992305416926,0.));
#20814=DIRECTION('',(0.949058110894923,0.31510109829158,0.));
#20815=DIRECTION('center_axis',(0.,0.,1.));
#20816=DIRECTION('ref_axis',(1.,0.,0.));
#20817=DIRECTION('',(-0.620695167978802,-0.784051980705212,0.));
#20818=DIRECTION('',(0.989356517167621,0.145511793123286,0.));
#20819=DIRECTION('center_axis',(0.,0.,1.));
#20820=DIRECTION('ref_axis',(1.,0.,0.));
#20821=DIRECTION('',(-0.747414611328347,-0.664357884556883,0.));
#20822=DIRECTION('',(0.999593826304735,-0.0284988142465376,0.));
#20823=DIRECTION('center_axis',(0.,0.,1.));
#20824=DIRECTION('ref_axis',(1.,0.,0.));
#20825=DIRECTION('',(-0.851424239922721,-0.524477610267604,0.));
#20826=DIRECTION('',(0.979458982848462,-0.201643499566577,0.));
#20827=DIRECTION('center_axis',(0.,0.,1.));
#20828=DIRECTION('ref_axis',(1.,0.,0.));
#20829=DIRECTION('',(-0.929563773828498,-0.368661349188819,0.));
#20830=DIRECTION('',(0.929563773828498,-0.368661349188819,0.));
#20831=DIRECTION('center_axis',(0.,0.,1.));
#20832=DIRECTION('ref_axis',(1.,0.,0.));
#20833=DIRECTION('',(-0.979458982848462,-0.201643499566578,0.));
#20834=DIRECTION('',(0.85142423992272,-0.524477610267605,0.));
#20835=DIRECTION('center_axis',(0.,0.,1.));
#20836=DIRECTION('ref_axis',(1.,0.,0.));
#20837=DIRECTION('center_axis',(0.,0.,1.));
#20838=DIRECTION('ref_axis',(1.,0.,0.));
#20839=DIRECTION('',(-1.,1.60246890531964E-16,0.));
#20840=DIRECTION('center_axis',(0.,0.,1.));
#20841=DIRECTION('ref_axis',(1.,0.,0.));
#20842=DIRECTION('center_axis',(0.,0.,1.));
#20843=DIRECTION('ref_axis',(1.,0.,0.));
#20844=DIRECTION('',(-0.5,0.866025403784439,0.));
#20845=DIRECTION('center_axis',(0.,0.,1.));
#20846=DIRECTION('ref_axis',(1.,0.,0.));
#20847=DIRECTION('center_axis',(0.,0.,1.));
#20848=DIRECTION('ref_axis',(1.,0.,0.));
#20849=DIRECTION('',(0.5,0.866025403784439,0.));
#20850=DIRECTION('center_axis',(0.,0.,1.));
#20851=DIRECTION('ref_axis',(1.,0.,0.));
#20852=DIRECTION('center_axis',(0.,0.,1.));
#20853=DIRECTION('ref_axis',(1.,0.,0.));
#20854=DIRECTION('',(1.,-1.60246890531964E-16,0.));
#20855=DIRECTION('center_axis',(0.,0.,1.));
#20856=DIRECTION('ref_axis',(1.,0.,0.));
#20857=DIRECTION('center_axis',(0.,0.,1.));
#20858=DIRECTION('ref_axis',(1.,0.,0.));
#20859=DIRECTION('',(0.5,-0.866025403784439,0.));
#20860=DIRECTION('center_axis',(0.,0.,1.));
#20861=DIRECTION('ref_axis',(1.,0.,0.));
#20862=DIRECTION('center_axis',(0.,0.,1.));
#20863=DIRECTION('ref_axis',(1.,0.,0.));
#20864=DIRECTION('',(-0.5,-0.866025403784439,0.));
#20865=DIRECTION('center_axis',(0.,0.,1.));
#20866=DIRECTION('ref_axis',(1.,0.,0.));
#20867=DIRECTION('center_axis',(0.,0.,1.));
#20868=DIRECTION('ref_axis',(1.,0.,0.));
#20869=DIRECTION('',(-0.85530665792059,-1.04744856091187E-16,0.518122110044255));
#20870=DIRECTION('center_axis',(0.,0.,-1.));
#20871=DIRECTION('ref_axis',(1.,0.,0.));
#20872=DIRECTION('center_axis',(0.,0.,-1.));
#20873=DIRECTION('ref_axis',(1.,0.,0.));
#20874=DIRECTION('center_axis',(0.,0.,-1.));
#20875=DIRECTION('ref_axis',(1.,0.,0.));
#20876=DIRECTION('center_axis',(0.,0.,-1.));
#20877=DIRECTION('ref_axis',(1.,0.,0.));
#20878=DIRECTION('center_axis',(0.,0.,-1.));
#20879=DIRECTION('ref_axis',(1.,0.,0.));
#20880=DIRECTION('center_axis',(0.,0.,-1.));
#20881=DIRECTION('ref_axis',(1.,0.,0.));
#20882=DIRECTION('center_axis',(0.,0.,-1.));
#20883=DIRECTION('ref_axis',(1.,0.,0.));
#20884=DIRECTION('center_axis',(-0.866025403784439,0.5,0.));
#20885=DIRECTION('ref_axis',(0.5,0.866025403784439,0.));
#20886=DIRECTION('',(0.,0.,-1.));
#20887=DIRECTION('',(0.5,0.866025403784439,0.));
#20888=DIRECTION('',(0.,0.,-1.));
#20889=DIRECTION('center_axis',(-0.866025403784439,0.5,0.));
#20890=DIRECTION('ref_axis',(0.5,0.866025403784439,0.));
#20891=DIRECTION('',(0.,0.,-1.));
#20892=DIRECTION('',(0.5,0.866025403784439,0.));
#20893=DIRECTION('center_axis',(1.60246890531964E-16,1.,0.));
#20894=DIRECTION('ref_axis',(1.,-1.60246890531964E-16,0.));
#20895=DIRECTION('',(0.,0.,-1.));
#20896=DIRECTION('',(1.,-1.60246890531964E-16,0.));
#20897=DIRECTION('center_axis',(1.60246890531964E-16,1.,0.));
#20898=DIRECTION('ref_axis',(1.,-1.60246890531964E-16,0.));
#20899=DIRECTION('',(1.,-1.60246890531964E-16,0.));
#20900=DIRECTION('',(0.,0.,-1.));
#20901=DIRECTION('center_axis',(1.60246890531964E-16,1.,0.));
#20902=DIRECTION('ref_axis',(1.,-1.60246890531964E-16,0.));
#20903=DIRECTION('',(0.,0.,-1.));
#20904=DIRECTION('',(1.,-1.60246890531964E-16,0.));
#20905=DIRECTION('center_axis',(-0.866025403784439,-0.5,0.));
#20906=DIRECTION('ref_axis',(-0.5,0.866025403784439,0.));
#20907=DIRECTION('',(-0.5,0.866025403784439,0.));
#20908=DIRECTION('',(0.,0.,-1.));
#20909=DIRECTION('center_axis',(-0.866025403784439,-0.5,0.));
#20910=DIRECTION('ref_axis',(-0.5,0.866025403784439,0.));
#20911=DIRECTION('',(0.,0.,-1.));
#20912=DIRECTION('',(-0.5,0.866025403784439,0.));
#20913=DIRECTION('center_axis',(0.866025403784439,0.5,0.));
#20914=DIRECTION('ref_axis',(0.5,-0.866025403784439,0.));
#20915=DIRECTION('',(0.,0.,-1.));
#20916=DIRECTION('',(0.5,-0.866025403784439,0.));
#20917=DIRECTION('center_axis',(0.866025403784439,0.5,0.));
#20918=DIRECTION('ref_axis',(0.5,-0.866025403784439,0.));
#20919=DIRECTION('',(0.5,-0.866025403784439,0.));
#20920=DIRECTION('',(0.,0.,-1.));
#20921=DIRECTION('center_axis',(0.866025403784439,0.5,0.));
#20922=DIRECTION('ref_axis',(0.5,-0.866025403784439,0.));
#20923=DIRECTION('',(0.5,-0.866025403784439,0.));
#20924=DIRECTION('center_axis',(0.,0.,-1.));
#20925=DIRECTION('ref_axis',(-1.,0.,0.));
#20926=DIRECTION('',(0.5,0.866025403784439,0.));
#20927=DIRECTION('center_axis',(0.,0.,-1.));
#20928=DIRECTION('ref_axis',(-1.,0.,0.));
#20929=DIRECTION('center_axis',(0.,0.,-1.));
#20930=DIRECTION('ref_axis',(-1.,0.,0.));
#20931=DIRECTION('',(-0.5,-0.866025403784439,0.));
#20932=DIRECTION('center_axis',(0.,0.,-1.));
#20933=DIRECTION('ref_axis',(-1.,0.,0.));
#20934=DIRECTION('',(-1.,1.60246890531964E-16,0.));
#20935=DIRECTION('',(-0.5,-0.866025403784439,0.));
#20936=DIRECTION('center_axis',(0.,0.,-1.));
#20937=DIRECTION('ref_axis',(-1.,0.,0.));
#20938=DIRECTION('',(-1.,1.60246890531964E-16,0.));
#20939=DIRECTION('center_axis',(0.,0.,-1.));
#20940=DIRECTION('ref_axis',(-1.,0.,0.));
#20941=DIRECTION('',(-0.5,0.866025403784439,0.));
#20942=DIRECTION('center_axis',(0.866025403784439,-0.5,0.));
#20943=DIRECTION('ref_axis',(-0.5,-0.866025403784439,0.));
#20944=DIRECTION('',(0.,0.,-1.));
#20945=DIRECTION('',(-0.5,-0.866025403784439,0.));
#20946=DIRECTION('center_axis',(0.866025403784439,-0.5,0.));
#20947=DIRECTION('ref_axis',(-0.5,-0.866025403784439,0.));
#20948=DIRECTION('',(0.,0.,-1.));
#20949=DIRECTION('center_axis',(0.866025403784439,-0.5,0.));
#20950=DIRECTION('ref_axis',(-0.5,-0.866025403784439,0.));
#20951=DIRECTION('center_axis',(-1.60246890531964E-16,-1.,0.));
#20952=DIRECTION('ref_axis',(-1.,1.60246890531964E-16,0.));
#20953=DIRECTION('center_axis',(-1.60246890531964E-16,-1.,0.));
#20954=DIRECTION('ref_axis',(-1.,1.60246890531964E-16,0.));
#20955=DIRECTION('',(-1.,1.60246890531964E-16,0.));
#20956=DIRECTION('center_axis',(-0.866025403784439,0.5,0.));
#20957=DIRECTION('ref_axis',(0.5,0.866025403784439,0.));
#20958=DIRECTION('center_axis',(-0.866025403784439,-0.5,0.));
#20959=DIRECTION('ref_axis',(-0.5,0.866025403784439,0.));
#20960=DIRECTION('center_axis',(-1.60246890531964E-16,-1.,0.));
#20961=DIRECTION('ref_axis',(-1.,1.60246890531964E-16,0.));
#20962=DIRECTION('center_axis',(-0.0284988142465338,0.999593826304735,0.));
#20963=DIRECTION('ref_axis',(0.999593826304735,0.0284988142465338,0.));
#20964=DIRECTION('',(0.,0.,-1.));
#20965=DIRECTION('',(0.,0.,-1.));
#20966=DIRECTION('center_axis',(-0.664357884556884,-0.747414611328346,0.));
#20967=DIRECTION('ref_axis',(-0.747414611328346,0.664357884556884,0.));
#20968=DIRECTION('',(0.,0.,1.));
#20969=DIRECTION('center_axis',(0.315101098291577,0.949058110894924,0.));
#20970=DIRECTION('ref_axis',(0.949058110894924,-0.315101098291577,0.));
#20971=DIRECTION('',(0.,0.,-1.));
#20972=DIRECTION('',(0.,0.,-1.));
#20973=DIRECTION('center_axis',(-0.879923054169258,-0.475116216037135,0.));
#20974=DIRECTION('ref_axis',(-0.475116216037135,0.879923054169258,0.));
#20975=DIRECTION('',(0.,0.,1.));
#20976=DIRECTION('center_axis',(0.620695167978805,0.78405198070521,0.));
#20977=DIRECTION('ref_axis',(0.78405198070521,-0.620695167978805,0.));
#20978=DIRECTION('',(0.,0.,-1.));
#20979=DIRECTION('',(0.,0.,-1.));
#20980=DIRECTION('center_axis',(-0.989356517167622,-0.145511793123284,0.));
#20981=DIRECTION('ref_axis',(-0.145511793123284,0.989356517167622,0.));
#20982=DIRECTION('',(0.,0.,1.));
#20983=DIRECTION('center_axis',(0.851424239922721,0.524477610267605,0.));
#20984=DIRECTION('ref_axis',(0.524477610267605,-0.851424239922721,0.));
#20985=DIRECTION('',(0.,0.,-1.));
#20986=DIRECTION('',(0.,0.,-1.));
#20987=DIRECTION('center_axis',(-0.979458982848463,0.201643499566573,0.));
#20988=DIRECTION('ref_axis',(0.201643499566573,0.979458982848463,0.));
#20989=DIRECTION('',(0.,0.,1.));
#20990=DIRECTION('center_axis',(0.979458982848462,0.201643499566578,0.));
#20991=DIRECTION('ref_axis',(0.201643499566578,-0.979458982848462,0.));
#20992=DIRECTION('',(0.,0.,-1.));
#20993=DIRECTION('',(0.,0.,-1.));
#20994=DIRECTION('center_axis',(-0.85142423992272,0.524477610267605,0.));
#20995=DIRECTION('ref_axis',(0.524477610267605,0.85142423992272,0.));
#20996=DIRECTION('',(0.,0.,1.));
#20997=DIRECTION('center_axis',(0.989356517167622,-0.145511793123284,0.));
#20998=DIRECTION('ref_axis',(-0.145511793123284,-0.989356517167622,0.));
#20999=DIRECTION('',(0.,0.,-1.));
#21000=DIRECTION('',(0.,0.,-1.));
#21001=DIRECTION('center_axis',(-0.620695167978805,0.78405198070521,0.));
#21002=DIRECTION('ref_axis',(0.78405198070521,0.620695167978805,0.));
#21003=DIRECTION('',(0.,0.,1.));
#21004=DIRECTION('center_axis',(0.879923054169259,-0.475116216037133,0.));
#21005=DIRECTION('ref_axis',(-0.475116216037133,-0.879923054169259,0.));
#21006=DIRECTION('',(0.,0.,-1.));
#21007=DIRECTION('',(0.,0.,-1.));
#21008=DIRECTION('center_axis',(-0.315101098291581,0.949058110894923,0.));
#21009=DIRECTION('ref_axis',(0.949058110894923,0.315101098291581,0.));
#21010=DIRECTION('',(0.,0.,1.));
#21011=DIRECTION('center_axis',(0.664357884556882,-0.747414611328348,0.));
#21012=DIRECTION('ref_axis',(-0.747414611328348,-0.664357884556882,0.));
#21013=DIRECTION('',(0.,0.,-1.));
#21014=DIRECTION('',(0.,0.,-1.));
#21015=DIRECTION('center_axis',(0.0284988142465371,0.999593826304735,0.));
#21016=DIRECTION('ref_axis',(0.999593826304735,-0.0284988142465371,0.));
#21017=DIRECTION('',(0.,0.,1.));
#21018=DIRECTION('center_axis',(0.368661349188818,-0.929563773828499,0.));
#21019=DIRECTION('ref_axis',(-0.929563773828499,-0.368661349188818,0.));
#21020=DIRECTION('',(0.,0.,-1.));
#21021=DIRECTION('',(0.,0.,-1.));
#21022=DIRECTION('center_axis',(0.368661349188818,0.929563773828499,0.));
#21023=DIRECTION('ref_axis',(0.929563773828499,-0.368661349188818,0.));
#21024=DIRECTION('',(0.,0.,1.));
#21025=DIRECTION('center_axis',(0.201643499566576,-0.979458982848462,0.));
#21026=DIRECTION('ref_axis',(-0.979458982848462,-0.201643499566576,0.));
#21027=DIRECTION('',(0.,0.,-1.));
#21028=DIRECTION('',(0.,0.,-1.));
#21029=DIRECTION('center_axis',(0.524477610267605,0.85142423992272,0.));
#21030=DIRECTION('ref_axis',(0.85142423992272,-0.524477610267605,0.));
#21031=DIRECTION('',(0.,0.,1.));
#21032=DIRECTION('center_axis',(-0.145511793123287,-0.989356517167621,0.));
#21033=DIRECTION('ref_axis',(-0.989356517167621,0.145511793123287,0.));
#21034=DIRECTION('',(0.,0.,-1.));
#21035=DIRECTION('',(0.,0.,-1.));
#21036=DIRECTION('center_axis',(0.784051980705213,0.620695167978801,0.));
#21037=DIRECTION('ref_axis',(0.620695167978801,-0.784051980705213,0.));
#21038=DIRECTION('',(0.,0.,1.));
#21039=DIRECTION('center_axis',(-0.475116216037133,-0.879923054169259,0.));
#21040=DIRECTION('ref_axis',(-0.879923054169259,0.475116216037133,0.));
#21041=DIRECTION('',(0.,0.,-1.));
#21042=DIRECTION('',(0.,0.,-1.));
#21043=DIRECTION('center_axis',(0.949058110894923,0.31510109829158,0.));
#21044=DIRECTION('ref_axis',(0.31510109829158,-0.949058110894923,0.));
#21045=DIRECTION('',(0.,0.,1.));
#21046=DIRECTION('center_axis',(-0.747414611328346,-0.664357884556883,0.));
#21047=DIRECTION('ref_axis',(-0.664357884556883,0.747414611328346,0.));
#21048=DIRECTION('',(0.,0.,-1.));
#21049=DIRECTION('',(0.,0.,-1.));
#21050=DIRECTION('center_axis',(0.999593826304735,-0.028498814246538,0.));
#21051=DIRECTION('ref_axis',(-0.028498814246538,-0.999593826304735,0.));
#21052=DIRECTION('',(0.,0.,1.));
#21053=DIRECTION('center_axis',(-0.929563773828498,-0.368661349188819,0.));
#21054=DIRECTION('ref_axis',(-0.368661349188819,0.929563773828498,0.));
#21055=DIRECTION('',(0.,0.,-1.));
#21056=DIRECTION('',(0.,0.,-1.));
#21057=DIRECTION('center_axis',(0.929563773828498,-0.368661349188819,0.));
#21058=DIRECTION('ref_axis',(-0.368661349188819,-0.929563773828498,0.));
#21059=DIRECTION('',(0.,0.,1.));
#21060=DIRECTION('center_axis',(-0.999593826304735,-0.0284988142465383,
0.));
#21061=DIRECTION('ref_axis',(-0.0284988142465383,0.999593826304735,0.));
#21062=DIRECTION('',(0.,0.,-1.));
#21063=DIRECTION('',(0.,0.,-1.));
#21064=DIRECTION('center_axis',(0.747414611328348,-0.664357884556882,0.));
#21065=DIRECTION('ref_axis',(-0.664357884556882,-0.747414611328348,0.));
#21066=DIRECTION('',(0.,0.,1.));
#21067=DIRECTION('center_axis',(-0.949058110894923,0.31510109829158,0.));
#21068=DIRECTION('ref_axis',(0.31510109829158,0.949058110894923,0.));
#21069=DIRECTION('',(0.,0.,-1.));
#21070=DIRECTION('',(0.,0.,-1.));
#21071=DIRECTION('center_axis',(0.475116216037132,-0.879923054169259,0.));
#21072=DIRECTION('ref_axis',(-0.879923054169259,-0.475116216037132,0.));
#21073=DIRECTION('',(0.,0.,1.));
#21074=DIRECTION('center_axis',(-0.784051980705212,0.620695167978802,0.));
#21075=DIRECTION('ref_axis',(0.620695167978802,0.784051980705212,0.));
#21076=DIRECTION('',(0.,0.,-1.));
#21077=DIRECTION('',(0.,0.,-1.));
#21078=DIRECTION('center_axis',(0.145511793123286,-0.989356517167621,0.));
#21079=DIRECTION('ref_axis',(-0.989356517167621,-0.145511793123286,0.));
#21080=DIRECTION('',(0.,0.,1.));
#21081=DIRECTION('center_axis',(-0.524477610267604,0.851424239922721,0.));
#21082=DIRECTION('ref_axis',(0.851424239922721,0.524477610267604,0.));
#21083=DIRECTION('',(0.,0.,-1.));
#21084=DIRECTION('',(0.,0.,-1.));
#21085=DIRECTION('center_axis',(-0.201643499566577,-0.979458982848462,0.));
#21086=DIRECTION('ref_axis',(-0.979458982848462,0.201643499566577,0.));
#21087=DIRECTION('',(0.,0.,1.));
#21088=DIRECTION('center_axis',(-0.664357884556883,0.747414611328347,0.));
#21089=DIRECTION('ref_axis',(0.747414611328347,0.664357884556883,0.));
#21090=DIRECTION('',(0.,0.,-1.));
#21091=DIRECTION('',(0.,0.,-1.));
#21092=DIRECTION('center_axis',(-0.0284988142465376,-0.999593826304735,
0.));
#21093=DIRECTION('ref_axis',(-0.999593826304735,0.0284988142465376,0.));
#21094=DIRECTION('',(0.,0.,1.));
#21095=DIRECTION('center_axis',(-0.87992305416926,0.475116216037132,0.));
#21096=DIRECTION('ref_axis',(0.475116216037132,0.87992305416926,0.));
#21097=DIRECTION('',(0.,0.,-1.));
#21098=DIRECTION('',(0.,0.,-1.));
#21099=DIRECTION('center_axis',(0.31510109829158,-0.949058110894923,0.));
#21100=DIRECTION('ref_axis',(-0.949058110894923,-0.31510109829158,0.));
#21101=DIRECTION('',(0.,0.,1.));
#21102=DIRECTION('center_axis',(-0.989356517167621,0.145511793123286,0.));
#21103=DIRECTION('ref_axis',(0.145511793123286,0.989356517167621,0.));
#21104=DIRECTION('',(0.,0.,-1.));
#21105=DIRECTION('',(0.,0.,-1.));
#21106=DIRECTION('center_axis',(0.620695167978803,-0.784051980705211,0.));
#21107=DIRECTION('ref_axis',(-0.784051980705211,-0.620695167978803,0.));
#21108=DIRECTION('',(0.,0.,1.));
#21109=DIRECTION('center_axis',(-0.979458982848462,-0.201643499566577,0.));
#21110=DIRECTION('ref_axis',(-0.201643499566577,0.979458982848462,0.));
#21111=DIRECTION('',(0.,0.,-1.));
#21112=DIRECTION('',(0.,0.,-1.));
#21113=DIRECTION('center_axis',(0.851424239922722,-0.524477610267603,0.));
#21114=DIRECTION('ref_axis',(-0.524477610267603,-0.851424239922722,0.));
#21115=DIRECTION('',(0.,0.,1.));
#21116=DIRECTION('center_axis',(-0.851424239922721,-0.524477610267604,0.));
#21117=DIRECTION('ref_axis',(-0.524477610267604,0.851424239922721,0.));
#21118=DIRECTION('',(0.,0.,-1.));
#21119=DIRECTION('',(0.,0.,-1.));
#21120=DIRECTION('center_axis',(0.979458982848462,-0.201643499566577,0.));
#21121=DIRECTION('ref_axis',(-0.201643499566577,-0.979458982848462,0.));
#21122=DIRECTION('',(0.,0.,1.));
#21123=DIRECTION('center_axis',(-0.620695167978802,-0.784051980705213,0.));
#21124=DIRECTION('ref_axis',(-0.784051980705213,0.620695167978802,0.));
#21125=DIRECTION('',(0.,0.,-1.));
#21126=DIRECTION('',(0.,0.,-1.));
#21127=DIRECTION('center_axis',(0.989356517167621,0.145511793123287,0.));
#21128=DIRECTION('ref_axis',(0.145511793123287,-0.989356517167621,0.));
#21129=DIRECTION('',(0.,0.,1.));
#21130=DIRECTION('center_axis',(-0.315101098291577,-0.949058110894924,0.));
#21131=DIRECTION('ref_axis',(-0.949058110894924,0.315101098291577,0.));
#21132=DIRECTION('',(0.,0.,-1.));
#21133=DIRECTION('',(0.,0.,-1.));
#21134=DIRECTION('center_axis',(0.879923054169259,0.475116216037132,0.));
#21135=DIRECTION('ref_axis',(0.475116216037132,-0.879923054169259,0.));
#21136=DIRECTION('',(0.,0.,1.));
#21137=DIRECTION('center_axis',(0.0284988142465395,-0.999593826304735,0.));
#21138=DIRECTION('ref_axis',(-0.999593826304735,-0.0284988142465395,0.));
#21139=DIRECTION('',(0.,0.,-1.));
#21140=DIRECTION('',(0.,0.,-1.));
#21141=DIRECTION('center_axis',(0.664357884556882,0.747414611328348,0.));
#21142=DIRECTION('ref_axis',(0.747414611328348,-0.664357884556882,0.));
#21143=DIRECTION('',(0.,0.,1.));
#21144=DIRECTION('center_axis',(-0.368661349188819,0.929563773828498,0.));
#21145=DIRECTION('ref_axis',(0.929563773828498,0.368661349188819,0.));
#21146=DIRECTION('',(0.,0.,-1.));
#21147=DIRECTION('',(0.,0.,-1.));
#21148=DIRECTION('center_axis',(-0.368661349188819,-0.929563773828498,0.));
#21149=DIRECTION('ref_axis',(-0.929563773828498,0.368661349188819,0.));
#21150=DIRECTION('',(0.,0.,1.));
#21151=DIRECTION('center_axis',(0.524477610267603,-0.851424239922722,0.));
#21152=DIRECTION('ref_axis',(-0.851424239922722,-0.524477610267603,0.));
#21153=DIRECTION('',(0.,0.,-1.));
#21154=DIRECTION('',(0.,0.,-1.));
#21155=DIRECTION('center_axis',(0.201643499566578,0.979458982848462,0.));
#21156=DIRECTION('ref_axis',(0.979458982848462,-0.201643499566578,0.));
#21157=DIRECTION('',(0.,0.,1.));
#21158=DIRECTION('center_axis',(0.784051980705211,-0.620695167978803,0.));
#21159=DIRECTION('ref_axis',(-0.620695167978803,-0.784051980705211,0.));
#21160=DIRECTION('',(0.,0.,-1.));
#21161=DIRECTION('',(0.,0.,-1.));
#21162=DIRECTION('center_axis',(-0.145511793123284,0.989356517167622,0.));
#21163=DIRECTION('ref_axis',(0.989356517167622,0.145511793123284,0.));
#21164=DIRECTION('',(0.,0.,1.));
#21165=DIRECTION('center_axis',(0.949058110894924,-0.315101098291578,0.));
#21166=DIRECTION('ref_axis',(-0.315101098291578,-0.949058110894924,0.));
#21167=DIRECTION('',(0.,0.,-1.));
#21168=DIRECTION('',(0.,0.,-1.));
#21169=DIRECTION('center_axis',(-0.475116216037132,0.879923054169259,0.));
#21170=DIRECTION('ref_axis',(0.879923054169259,0.475116216037132,0.));
#21171=DIRECTION('',(0.,0.,1.));
#21172=DIRECTION('center_axis',(0.999593826304735,0.0284988142465341,0.));
#21173=DIRECTION('ref_axis',(0.0284988142465341,-0.999593826304735,0.));
#21174=DIRECTION('',(0.,0.,-1.));
#21175=DIRECTION('',(0.,0.,-1.));
#21176=DIRECTION('center_axis',(-0.747414611328346,0.664357884556884,0.));
#21177=DIRECTION('ref_axis',(0.664357884556884,0.747414611328346,0.));
#21178=DIRECTION('',(0.,0.,1.));
#21179=DIRECTION('center_axis',(0.929563773828498,0.368661349188821,0.));
#21180=DIRECTION('ref_axis',(0.368661349188821,-0.929563773828498,0.));
#21181=DIRECTION('',(0.,0.,-1.));
#21182=DIRECTION('',(0.,0.,-1.));
#21183=DIRECTION('center_axis',(-0.929563773828498,0.368661349188821,0.));
#21184=DIRECTION('ref_axis',(0.368661349188821,0.929563773828498,0.));
#21185=DIRECTION('',(0.,0.,1.));
#21186=DIRECTION('center_axis',(0.747414611328349,0.66435788455688,0.));
#21187=DIRECTION('ref_axis',(0.66435788455688,-0.747414611328349,0.));
#21188=DIRECTION('',(0.,0.,-1.));
#21189=DIRECTION('',(0.,0.,-1.));
#21190=DIRECTION('center_axis',(-0.999593826304735,0.028498814246539,0.));
#21191=DIRECTION('ref_axis',(0.028498814246539,0.999593826304735,0.));
#21192=DIRECTION('',(0.,0.,1.));
#21193=DIRECTION('center_axis',(0.475116216037131,0.87992305416926,0.));
#21194=DIRECTION('ref_axis',(0.87992305416926,-0.475116216037131,0.));
#21195=DIRECTION('',(0.,0.,-1.));
#21196=DIRECTION('',(0.,0.,-1.));
#21197=DIRECTION('center_axis',(-0.949058110894924,-0.315101098291577,0.));
#21198=DIRECTION('ref_axis',(-0.315101098291577,0.949058110894924,0.));
#21199=DIRECTION('',(0.,0.,1.));
#21200=DIRECTION('center_axis',(0.145511793123284,0.989356517167622,0.));
#21201=DIRECTION('ref_axis',(0.989356517167622,-0.145511793123284,0.));
#21202=DIRECTION('',(0.,0.,-1.));
#21203=DIRECTION('',(0.,0.,-1.));
#21204=DIRECTION('center_axis',(-0.78405198070521,-0.620695167978805,0.));
#21205=DIRECTION('ref_axis',(-0.620695167978805,0.78405198070521,0.));
#21206=DIRECTION('',(0.,0.,1.));
#21207=DIRECTION('center_axis',(-0.201643499566578,0.979458982848462,0.));
#21208=DIRECTION('ref_axis',(0.979458982848462,0.201643499566578,0.));
#21209=DIRECTION('',(0.,0.,-1.));
#21210=DIRECTION('',(0.,0.,-1.));
#21211=DIRECTION('center_axis',(-0.524477610267605,-0.85142423992272,0.));
#21212=DIRECTION('ref_axis',(-0.85142423992272,0.524477610267605,0.));
#21213=DIRECTION('',(0.,0.,1.));
#21214=DIRECTION('center_axis',(0.,0.,1.));
#21215=DIRECTION('ref_axis',(1.,0.,0.));
#21216=DIRECTION('center_axis',(0.,0.,1.));
#21217=DIRECTION('ref_axis',(1.,0.,0.));
#21218=DIRECTION('center_axis',(0.,0.,1.));
#21219=DIRECTION('ref_axis',(1.,0.,0.));
#21220=DIRECTION('center_axis',(0.,0.,1.));
#21221=DIRECTION('ref_axis',(1.,0.,0.));
#21222=DIRECTION('center_axis',(0.,0.,1.));
#21223=DIRECTION('ref_axis',(1.,0.,0.));
#21224=DIRECTION('center_axis',(0.,0.,1.));
#21225=DIRECTION('ref_axis',(1.,0.,0.));
#21226=DIRECTION('center_axis',(0.,0.,1.));
#21227=DIRECTION('ref_axis',(1.,0.,0.));
#21228=DIRECTION('center_axis',(0.,0.,1.));
#21229=DIRECTION('ref_axis',(1.,0.,0.));
#21230=DIRECTION('center_axis',(0.,0.,1.));
#21231=DIRECTION('ref_axis',(1.,0.,0.));
#21232=DIRECTION('center_axis',(0.,0.,1.));
#21233=DIRECTION('ref_axis',(1.,0.,0.));
#21234=DIRECTION('center_axis',(0.,0.,1.));
#21235=DIRECTION('ref_axis',(1.,0.,0.));
#21236=DIRECTION('center_axis',(0.,0.,1.));
#21237=DIRECTION('ref_axis',(1.,0.,0.));
#21238=DIRECTION('center_axis',(0.,0.,1.));
#21239=DIRECTION('ref_axis',(1.,0.,0.));
#21240=DIRECTION('center_axis',(0.,0.,1.));
#21241=DIRECTION('ref_axis',(1.,0.,0.));
#21242=DIRECTION('center_axis',(0.,0.,1.));
#21243=DIRECTION('ref_axis',(1.,0.,0.));
#21244=DIRECTION('center_axis',(0.,0.,1.));
#21245=DIRECTION('ref_axis',(1.,0.,0.));
#21246=DIRECTION('center_axis',(0.,0.,1.));
#21247=DIRECTION('ref_axis',(1.,0.,0.));
#21248=DIRECTION('center_axis',(0.,0.,1.));
#21249=DIRECTION('ref_axis',(1.,0.,0.));
#21250=DIRECTION('center_axis',(0.,0.,1.));
#21251=DIRECTION('ref_axis',(1.,0.,0.));
#21252=DIRECTION('center_axis',(0.,0.,1.));
#21253=DIRECTION('ref_axis',(1.,0.,0.));
#21254=DIRECTION('center_axis',(0.,0.,1.));
#21255=DIRECTION('ref_axis',(1.,0.,0.));
#21256=DIRECTION('center_axis',(0.,0.,1.));
#21257=DIRECTION('ref_axis',(1.,0.,0.));
#21258=DIRECTION('center_axis',(0.,0.,1.));
#21259=DIRECTION('ref_axis',(1.,0.,0.));
#21260=DIRECTION('center_axis',(0.,0.,1.));
#21261=DIRECTION('ref_axis',(1.,0.,0.));
#21262=DIRECTION('center_axis',(0.,0.,1.));
#21263=DIRECTION('ref_axis',(1.,0.,0.));
#21264=DIRECTION('center_axis',(0.,0.,1.));
#21265=DIRECTION('ref_axis',(1.,0.,0.));
#21266=DIRECTION('center_axis',(0.,0.,1.));
#21267=DIRECTION('ref_axis',(1.,0.,0.));
#21268=DIRECTION('center_axis',(0.,0.,1.));
#21269=DIRECTION('ref_axis',(1.,0.,0.));
#21270=DIRECTION('center_axis',(0.,0.,1.));
#21271=DIRECTION('ref_axis',(1.,0.,0.));
#21272=DIRECTION('center_axis',(0.,0.,1.));
#21273=DIRECTION('ref_axis',(1.,0.,0.));
#21274=DIRECTION('center_axis',(0.,0.,1.));
#21275=DIRECTION('ref_axis',(1.,0.,0.));
#21276=DIRECTION('center_axis',(0.,0.,1.));
#21277=DIRECTION('ref_axis',(1.,0.,0.));
#21278=DIRECTION('center_axis',(0.,0.,1.));
#21279=DIRECTION('ref_axis',(1.,0.,0.));
#21280=DIRECTION('center_axis',(0.,0.,1.));
#21281=DIRECTION('ref_axis',(1.,0.,0.));
#21282=DIRECTION('center_axis',(0.,0.,1.));
#21283=DIRECTION('ref_axis',(1.,0.,0.));
#21284=DIRECTION('center_axis',(0.,0.,1.));
#21285=DIRECTION('ref_axis',(1.,0.,0.));
#21286=DIRECTION('center_axis',(0.,0.,1.));
#21287=DIRECTION('ref_axis',(1.,0.,0.));
#21288=DIRECTION('center_axis',(0.,0.,1.));
#21289=DIRECTION('ref_axis',(1.,0.,0.));
#21290=DIRECTION('center_axis',(0.,0.,1.));
#21291=DIRECTION('ref_axis',(1.,0.,0.));
#21292=DIRECTION('center_axis',(0.,0.,1.));
#21293=DIRECTION('ref_axis',(1.,0.,0.));
#21294=DIRECTION('center_axis',(0.,0.,1.));
#21295=DIRECTION('ref_axis',(1.,0.,0.));
#21296=DIRECTION('center_axis',(0.,0.,1.));
#21297=DIRECTION('ref_axis',(1.,0.,0.));
#21298=DIRECTION('center_axis',(0.,0.,1.));
#21299=DIRECTION('ref_axis',(1.,0.,0.));
#21300=DIRECTION('center_axis',(0.,0.,1.));
#21301=DIRECTION('ref_axis',(1.,0.,0.));
#21302=DIRECTION('center_axis',(0.,0.,1.));
#21303=DIRECTION('ref_axis',(1.,0.,0.));
#21304=DIRECTION('center_axis',(0.,0.,1.));
#21305=DIRECTION('ref_axis',(1.,0.,0.));
#21306=DIRECTION('center_axis',(0.,0.,1.));
#21307=DIRECTION('ref_axis',(1.,0.,0.));
#21308=DIRECTION('center_axis',(0.,0.,1.));
#21309=DIRECTION('ref_axis',(1.,0.,0.));
#21310=DIRECTION('center_axis',(0.,0.,1.));
#21311=DIRECTION('ref_axis',(1.,0.,0.));
#21312=DIRECTION('center_axis',(0.,0.,1.));
#21313=DIRECTION('ref_axis',(1.,0.,0.));
#21314=DIRECTION('center_axis',(0.,0.,1.));
#21315=DIRECTION('ref_axis',(1.,0.,0.));
#21316=DIRECTION('center_axis',(0.,0.,1.));
#21317=DIRECTION('ref_axis',(1.,0.,0.));
#21318=DIRECTION('center_axis',(0.,0.,1.));
#21319=DIRECTION('ref_axis',(1.,0.,0.));
#21320=DIRECTION('center_axis',(0.,0.,1.));
#21321=DIRECTION('ref_axis',(1.,0.,0.));
#21322=DIRECTION('center_axis',(0.,0.,1.));
#21323=DIRECTION('ref_axis',(1.,0.,0.));
#21324=DIRECTION('center_axis',(0.,0.,1.));
#21325=DIRECTION('ref_axis',(1.,0.,0.));
#21326=DIRECTION('center_axis',(0.,0.,1.));
#21327=DIRECTION('ref_axis',(1.,0.,0.));
#21328=DIRECTION('center_axis',(0.,0.,1.));
#21329=DIRECTION('ref_axis',(1.,0.,0.));
#21330=DIRECTION('center_axis',(0.,0.,1.));
#21331=DIRECTION('ref_axis',(1.,0.,0.));
#21332=DIRECTION('center_axis',(0.,0.,1.));
#21333=DIRECTION('ref_axis',(1.,0.,0.));
#21334=DIRECTION('center_axis',(0.,0.,1.));
#21335=DIRECTION('ref_axis',(1.,0.,0.));
#21336=DIRECTION('center_axis',(0.,0.,1.));
#21337=DIRECTION('ref_axis',(1.,0.,0.));
#21338=DIRECTION('center_axis',(0.,0.,1.));
#21339=DIRECTION('ref_axis',(1.,0.,0.));
#21340=DIRECTION('center_axis',(0.,0.,1.));
#21341=DIRECTION('ref_axis',(1.,0.,0.));
#21342=DIRECTION('center_axis',(0.,0.,1.));
#21343=DIRECTION('ref_axis',(1.,0.,0.));
#21344=DIRECTION('center_axis',(0.,0.,1.));
#21345=DIRECTION('ref_axis',(1.,0.,0.));
#21346=DIRECTION('center_axis',(0.,0.,1.));
#21347=DIRECTION('ref_axis',(1.,0.,0.));
#21348=DIRECTION('center_axis',(0.,0.,1.));
#21349=DIRECTION('ref_axis',(1.,0.,0.));
#21350=DIRECTION('center_axis',(0.,0.,1.));
#21351=DIRECTION('ref_axis',(1.,0.,0.));
#21352=DIRECTION('center_axis',(0.,0.,1.));
#21353=DIRECTION('ref_axis',(1.,0.,0.));
#21354=DIRECTION('center_axis',(0.,0.,1.));
#21355=DIRECTION('ref_axis',(1.,0.,0.));
#21356=DIRECTION('center_axis',(0.,0.,1.));
#21357=DIRECTION('ref_axis',(1.,0.,0.));
#21358=DIRECTION('center_axis',(0.,0.,-1.));
#21359=DIRECTION('ref_axis',(-1.,0.,0.));
#21360=DIRECTION('center_axis',(0.,0.,1.));
#21361=DIRECTION('ref_axis',(1.,0.,0.));
#21362=DIRECTION('center_axis',(0.,0.,1.));
#21363=DIRECTION('ref_axis',(1.,0.,0.));
#21364=DIRECTION('',(0.707106781186547,8.65956056235493E-17,-0.707106781186548));
#21365=DIRECTION('center_axis',(0.,0.,-1.));
#21366=DIRECTION('ref_axis',(1.,0.,0.));
#21367=DIRECTION('center_axis',(0.,0.,1.));
#21368=DIRECTION('ref_axis',(1.,0.,0.));
#21369=DIRECTION('',(-0.707106781186547,-8.65956056235493E-17,-0.707106781186548));
#21370=DIRECTION('center_axis',(0.,0.,1.));
#21371=DIRECTION('ref_axis',(1.,0.,0.));
#32268=CARTESIAN_POINT('',(0.,0.,0.));
#32269=CARTESIAN_POINT('Origin',(0.,0.,-0.78));
#32270=CARTESIAN_POINT('',(-0.195637724447267,0.00012546577000477,-1.54201303078758));
#32271=CARTESIAN_POINT('',(-0.195587655102992,0.000207352658957182,-1.55218696921242));
#32272=CARTESIAN_POINT('',(-0.1954,-2.39295984553393E-17,-0.78));
#32273=CARTESIAN_POINT('',(0.0862546635467556,0.175513015753855,-1.5646));
#32274=CARTESIAN_POINT('Ctrl Pts',(-0.195637724447267,0.00012546577000477,
-1.54201303078758));
#32275=CARTESIAN_POINT('Ctrl Pts',(-0.195682516033621,0.00666912291098706,
-1.54238744588469));
#32276=CARTESIAN_POINT('Ctrl Pts',(-0.195382767802269,0.0132083530144186,
-1.5427618609818));
#32277=CARTESIAN_POINT('Ctrl Pts',(-0.194724996523875,0.0197110274438995,
-1.54313627607892));
#32278=CARTESIAN_POINT('Ctrl Pts',(-0.188214434300664,0.084073926647727,
-1.54684220375794));
#32279=CARTESIAN_POINT('Ctrl Pts',(-0.146628833277563,0.144855515394664,
-1.55054813143696));
#32280=CARTESIAN_POINT('Ctrl Pts',(-0.0889996456239889,0.174295519526702,
-1.55425405911599));
#32281=CARTESIAN_POINT('Ctrl Pts',(-0.0353713128287438,0.201691677677969,
-1.55770270607733));
#32282=CARTESIAN_POINT('Ctrl Pts',(0.0321503086444766,0.201946916986755,
-1.56115135303866));
#32283=CARTESIAN_POINT('Ctrl Pts',(0.0863567411264609,0.175643900344955,
-1.5646));
#32284=CARTESIAN_POINT('',(-0.0861525859670576,0.175382131162752,-1.5646));
#32285=CARTESIAN_POINT('Origin',(0.,0.,-1.5646));
#32286=CARTESIAN_POINT('Ctrl Pts',(-0.0861525859670577,0.175382131162752,
-1.5646));
#32287=CARTESIAN_POINT('Ctrl Pts',(-0.144492275190264,0.146724051472584,
-1.56089407232098));
#32288=CARTESIAN_POINT('Ctrl Pts',(-0.186904019075789,0.0869180855456786,
-1.55718814464195));
#32289=CARTESIAN_POINT('Ctrl Pts',(-0.194378234588094,0.0227586785356969,
-1.55348221696293));
#32290=CARTESIAN_POINT('Ctrl Pts',(-0.195248998192385,0.015283957422126,
-1.55305046771276));
#32291=CARTESIAN_POINT('Ctrl Pts',(-0.195645561870275,0.00775014794319802,
-1.55261871846259));
#32292=CARTESIAN_POINT('Ctrl Pts',(-0.195587655102992,0.000207352658957182,
-1.55218696921242));
#32293=CARTESIAN_POINT('Origin',(0.,0.,-0.78));
#32294=CARTESIAN_POINT('',(-0.195133752959054,0.000103804320281162,-1.47201303078758));
#32295=CARTESIAN_POINT('',(-0.195118236033235,9.10413472694931E-5,-1.48218696921242));
#32296=CARTESIAN_POINT('',(-0.1954,-2.39295984553393E-17,-0.78));
#32297=CARTESIAN_POINT('Ctrl Pts',(-0.195133752959054,0.000103804320281162,
-1.47201303078758));
#32298=CARTESIAN_POINT('Ctrl Pts',(-0.195258187527039,0.0260059607083059,
-1.47348521314388));
#32299=CARTESIAN_POINT('Ctrl Pts',(-0.190466419891253,0.0518638912152906,
-1.47495739550018));
#32300=CARTESIAN_POINT('Ctrl Pts',(-0.180541931478085,0.0755732040417753,
-1.47642957785648));
#32301=CARTESIAN_POINT('Ctrl Pts',(-0.155558996345714,0.13525670607411,
-1.48013550553551));
#32302=CARTESIAN_POINT('Ctrl Pts',(-0.0980509865883601,0.181324826824306,
-1.48384143321453));
#32303=CARTESIAN_POINT('Ctrl Pts',(-0.0343538193840795,0.192681916213057,
-1.48754736089356));
#32304=CARTESIAN_POINT('Ctrl Pts',(0.0293433478202012,0.204039005601809,
-1.49125328857258));
#32305=CARTESIAN_POINT('Ctrl Pts',(0.0992296724714088,0.180685063629116,
-1.4949592162516));
#32306=CARTESIAN_POINT('Ctrl Pts',(0.143299710901451,0.133312212932569,
-1.49866514393063));
#32307=CARTESIAN_POINT('Ctrl Pts',(0.187369749331493,0.0859393622360219,
-1.50237107160965));
#32308=CARTESIAN_POINT('Ctrl Pts',(0.20562350154037,0.0145476028156198,
-1.50607699928868));
#32309=CARTESIAN_POINT('Ctrl Pts',(0.189702523682121,-0.0481630516398937,
-1.5097829269677));
#32310=CARTESIAN_POINT('Ctrl Pts',(0.173781545823872,-0.110873706095407,
-1.51348885464672));
#32311=CARTESIAN_POINT('Ctrl Pts',(0.123685837898497,-0.164903255586032,
-1.51719478232575));
#32312=CARTESIAN_POINT('Ctrl Pts',(0.0623551946746678,-0.185519277998796,
-1.52090071000477));
#32313=CARTESIAN_POINT('Ctrl Pts',(0.00102455145083888,-0.20613530041156,
-1.5246066376838));
#32314=CARTESIAN_POINT('Ctrl Pts',(-0.0715410270714442,-0.193337795746463,
-1.52831256536282));
#32315=CARTESIAN_POINT('Ctrl Pts',(-0.122106054620926,-0.152966938583555,
-1.53201849304185));
#32316=CARTESIAN_POINT('Ctrl Pts',(-0.167562426162996,-0.116674806024679,
-1.53535000562376));
#32317=CARTESIAN_POINT('Ctrl Pts',(-0.195239172853987,-0.0580994195644015,
-1.53868151820567));
#32318=CARTESIAN_POINT('Ctrl Pts',(-0.195637724447267,0.00012546577000477,
-1.54201303078758));
#32319=CARTESIAN_POINT('Ctrl Pts',(-0.195587655102992,0.000207352658957182,
-1.55218696921242));
#32320=CARTESIAN_POINT('Ctrl Pts',(-0.195148518061644,-0.0569935749705506,
-1.54891279078357));
#32321=CARTESIAN_POINT('Ctrl Pts',(-0.1685728979999,-0.11471127404357,-1.54563861235471));
#32322=CARTESIAN_POINT('Ctrl Pts',(-0.12446534008773,-0.151094701643577,
-1.54236443392585));
#32323=CARTESIAN_POINT('Ctrl Pts',(-0.0745415429359771,-0.19227582671981,
-1.53865850624683));
#32324=CARTESIAN_POINT('Ctrl Pts',(-0.00215726149338587,-0.206125228779217,
-1.53495257856781));
#32325=CARTESIAN_POINT('Ctrl Pts',(0.0594903019840149,-0.186442379139412,
-1.53124665088878));
#32326=CARTESIAN_POINT('Ctrl Pts',(0.121137865461415,-0.166759529499608,
-1.52754072320976));
#32327=CARTESIAN_POINT('Ctrl Pts',(0.172048710973626,-0.113544428160594,
-1.52383479553073));
#32328=CARTESIAN_POINT('Ctrl Pts',(0.188932843502802,-0.0510952853773085,
-1.52012886785171));
#32329=CARTESIAN_POINT('Ctrl Pts',(0.205816976031979,0.0113538574059772,
-1.51642294017269));
#32330=CARTESIAN_POINT('Ctrl Pts',(0.188674395578121,0.0830370416335339,
-1.51271701249366));
#32331=CARTESIAN_POINT('Ctrl Pts',(0.145342587498244,0.131088915832698,
-1.50901108481464));
#32332=CARTESIAN_POINT('Ctrl Pts',(0.102010779418367,0.179140790031861,
-1.50530515713561));
#32333=CARTESIAN_POINT('Ctrl Pts',(0.0324897437124708,0.203561354202632,
-1.50159922945659));
#32334=CARTESIAN_POINT('Ctrl Pts',(-0.0313760153042664,0.193186735136454,
-1.49789330177757));
#32335=CARTESIAN_POINT('Ctrl Pts',(-0.0952417743210041,0.182812116070276,
-1.49418737409854));
#32336=CARTESIAN_POINT('Ctrl Pts',(-0.153452256648582,0.137642313767148,
-1.49048144641952));
#32337=CARTESIAN_POINT('Ctrl Pts',(-0.179353177562788,0.078352807176984,
-1.48677551874049));
#32338=CARTESIAN_POINT('Ctrl Pts',(-0.190043047840084,0.0538827454230738,
-1.48524600223114));
#32339=CARTESIAN_POINT('Ctrl Pts',(-0.195229335108952,0.0270075453386261,
-1.48371648572178));
#32340=CARTESIAN_POINT('Ctrl Pts',(-0.195118236033235,9.10413472694931E-5,
-1.48218696921242));
#32341=CARTESIAN_POINT('Origin',(0.,0.,-0.78));
#32342=CARTESIAN_POINT('',(-0.195261827018658,-0.000164675523070867,-1.40201303078758));
#32343=CARTESIAN_POINT('',(-0.195289109418146,-0.000170586953657092,-1.41218696921242));
#32344=CARTESIAN_POINT('',(-0.1954,-2.39295984553393E-17,-0.78));
#32345=CARTESIAN_POINT('Ctrl Pts',(-0.195261827018658,-0.000164675523070867,
-1.40201303078758));
#32346=CARTESIAN_POINT('Ctrl Pts',(-0.194901371524036,0.0449773888177153,
-1.40458298040307));
#32347=CARTESIAN_POINT('Ctrl Pts',(-0.179326084199164,0.0903439266065276,
-1.40715293001856));
#32348=CARTESIAN_POINT('Ctrl Pts',(-0.150695208685029,0.124890480133385,
-1.40972287963405));
#32349=CARTESIAN_POINT('Ctrl Pts',(-0.109408814040175,0.174707421352147,
-1.41342880731307));
#32350=CARTESIAN_POINT('Ctrl Pts',(-0.0409742153629937,0.202024944228984,
-1.4171347349921));
#32351=CARTESIAN_POINT('Ctrl Pts',(0.0232684964003089,0.194332833555041,
-1.42084066267112));
#32352=CARTESIAN_POINT('Ctrl Pts',(0.0875112081636115,0.186640722881098,
-1.42454659035014));
#32353=CARTESIAN_POINT('Ctrl Pts',(0.147562033013035,0.143938978656375,
-1.42825251802917));
#32354=CARTESIAN_POINT('Ctrl Pts',(0.175920270422902,0.0857830967001064,
-1.43195844570819));
#32355=CARTESIAN_POINT('Ctrl Pts',(0.204278507832768,0.0276272147438382,
-1.43566437338722));
#32356=CARTESIAN_POINT('Ctrl Pts',(0.200944157803076,-0.0459828049439756,
-1.43937030106624));
#32357=CARTESIAN_POINT('Ctrl Pts',(0.167444229718402,-0.101336626764053,
-1.44307622874526));
#32358=CARTESIAN_POINT('Ctrl Pts',(0.133944301633728,-0.15669044858413,
-1.44678215642429));
#32359=CARTESIAN_POINT('Ctrl Pts',(0.0702787954940723,-0.19378807253647,
-1.45048808410331));
#32360=CARTESIAN_POINT('Ctrl Pts',(0.0056037295943023,-0.195640612534423,
-1.45419401178234));
#32361=CARTESIAN_POINT('Ctrl Pts',(-0.0590713363054679,-0.197493152532377,
-1.45789993946136));
#32362=CARTESIAN_POINT('Ctrl Pts',(-0.124755961965352,-0.164100608575943,
-1.46160586714039));
#32363=CARTESIAN_POINT('Ctrl Pts',(-0.1613693445416,-0.110754894940489,
-1.46531179481941));
#32364=CARTESIAN_POINT('Ctrl Pts',(-0.18343803534246,-0.0786008032686692,
-1.46754554014213));
#32365=CARTESIAN_POINT('Ctrl Pts',(-0.194944948132647,-0.0391975909399579,
-1.46977928546485));
#32366=CARTESIAN_POINT('Ctrl Pts',(-0.195133752959054,0.000103804320281162,
-1.47201303078758));
#32367=CARTESIAN_POINT('Ctrl Pts',(-0.195118236033235,9.10413472694931E-5,
-1.48218696921242));
#32368=CARTESIAN_POINT('Ctrl Pts',(-0.194960148645584,-0.038209545522401,
-1.48001055804276));
#32369=CARTESIAN_POINT('Ctrl Pts',(-0.184076125244741,-0.0765937628909216,
-1.47783414687309));
#32370=CARTESIAN_POINT('Ctrl Pts',(-0.163060241772941,-0.108251136057374,
-1.47565773570342));
#32371=CARTESIAN_POINT('Ctrl Pts',(-0.127275025568055,-0.162156361824368,
-1.4719518080244));
#32372=CARTESIAN_POINT('Ctrl Pts',(-0.0621132336574516,-0.196557602481156,
-1.46824588034537));
#32373=CARTESIAN_POINT('Ctrl Pts',(0.00258284575506351,-0.195703428168071,
-1.46453995266635));
#32374=CARTESIAN_POINT('Ctrl Pts',(0.0672789251675789,-0.194849253854986,
-1.46083402498732));
#32375=CARTESIAN_POINT('Ctrl Pts',(0.131509292082006,-0.158739664572028,
-1.4571280973083));
#32376=CARTESIAN_POINT('Ctrl Pts',(0.165859730099399,-0.103909795361192,
-1.45342216962928));
#32377=CARTESIAN_POINT('Ctrl Pts',(0.200210168116792,-0.0490799261503554,
-1.44971624195025));
#32378=CARTESIAN_POINT('Ctrl Pts',(0.204680677237152,0.0244702229883598,
-1.44601031427123));
#32379=CARTESIAN_POINT('Ctrl Pts',(0.177223681968522,0.0830570652693294,
-1.4423043865922));
#32380=CARTESIAN_POINT('Ctrl Pts',(0.149766686699892,0.141643907550299,
-1.43859845891318));
#32381=CARTESIAN_POINT('Ctrl Pts',(0.0903821870422722,0.185267442973523,
-1.43489253123416));
#32382=CARTESIAN_POINT('Ctrl Pts',(0.0262658688812991,0.193950386786294,
-1.43118660355513));
#32383=CARTESIAN_POINT('Ctrl Pts',(-0.037850449279674,0.202633330599066,
-1.42748067587611));
#32384=CARTESIAN_POINT('Ctrl Pts',(-0.106698585944001,0.176375682801386,
-1.42377474819708));
#32385=CARTESIAN_POINT('Ctrl Pts',(-0.14874913778196,0.127202096684771,
-1.42006882051806));
#32386=CARTESIAN_POINT('Ctrl Pts',(-0.178560494578678,0.0923409294319494,
-1.41744153674951));
#32387=CARTESIAN_POINT('Ctrl Pts',(-0.194903459622422,0.0459622751866913,
-1.41481425298097));
#32388=CARTESIAN_POINT('Ctrl Pts',(-0.195289109418146,-0.000170586953657092,
-1.41218696921242));
#32389=CARTESIAN_POINT('Origin',(0.,0.,-0.78));
#32390=CARTESIAN_POINT('',(-0.195719920316492,-1.24737763093352E-5,-1.33201303078758));
#32391=CARTESIAN_POINT('',(-0.195720657836488,6.2470732444266E-6,-1.34218696921242));
#32392=CARTESIAN_POINT('',(-0.1954,-2.39295984553393E-17,-0.78));
#32393=CARTESIAN_POINT('Ctrl Pts',(-0.195719920316492,-1.24737763093352E-5,
-1.33201303078758));
#32394=CARTESIAN_POINT('Ctrl Pts',(-0.195660878792609,0.0640228661772434,
-1.33568074766226));
#32395=CARTESIAN_POINT('Ctrl Pts',(-0.161227285905486,0.128112651091001,
-1.33934846453694));
#32396=CARTESIAN_POINT('Ctrl Pts',(-0.107775864067362,0.163373927248327,
-1.34301618141161));
#32397=CARTESIAN_POINT('Ctrl Pts',(-0.0537675775933861,0.199002560475527,
-1.34672210909064));
#32398=CARTESIAN_POINT('Ctrl Pts',(0.0196568629634197,0.205198876826011,
-1.35042803676966));
#32399=CARTESIAN_POINT('Ctrl Pts',(0.0788722285210952,0.179125231162566,
-1.35413396444869));
#32400=CARTESIAN_POINT('Ctrl Pts',(0.138087594078771,0.15305158549912,-1.35783989212771));
#32401=CARTESIAN_POINT('Ctrl Pts',(0.183093884637317,0.0947079778217447,
-1.36154581980673));
#32402=CARTESIAN_POINT('Ctrl Pts',(0.193280158649522,0.030813264537062,
-1.36525174748576));
#32403=CARTESIAN_POINT('Ctrl Pts',(0.203466432661727,-0.0330814487476208,
-1.36895767516478));
#32404=CARTESIAN_POINT('Ctrl Pts',(0.178832690127592,-0.102527267639611,
-1.37266360284381));
#32405=CARTESIAN_POINT('Ctrl Pts',(0.130660123857593,-0.145720997675018,
-1.37636953052283));
#32406=CARTESIAN_POINT('Ctrl Pts',(0.0824875575875941,-0.188914727710426,
-1.38007545820185));
#32407=CARTESIAN_POINT('Ctrl Pts',(0.0107761675817305,-0.20585636888925,
-1.38378138588088));
#32408=CARTESIAN_POINT('Ctrl Pts',(-0.0516333211096683,-0.188787384501775,
-1.3874873135599));
#32409=CARTESIAN_POINT('Ctrl Pts',(-0.114042809801067,-0.171718400114301,
-1.39119324123893));
#32410=CARTESIAN_POINT('Ctrl Pts',(-0.167150397178,-0.120638790160527,-1.39489916891795));
#32411=CARTESIAN_POINT('Ctrl Pts',(-0.186635095560204,-0.0589408054032964,
-1.39860509659698));
#32412=CARTESIAN_POINT('Ctrl Pts',(-0.192607740429136,-0.0400285212685705,
-1.39974107466051));
#32413=CARTESIAN_POINT('Ctrl Pts',(-0.195421156809523,-0.0201185277405092,
-1.40087705272404));
#32414=CARTESIAN_POINT('Ctrl Pts',(-0.195261827018658,-0.000164675523070867,
-1.40201303078758));
#32415=CARTESIAN_POINT('Ctrl Pts',(-0.195289109418146,-0.000170586953657092,
-1.41218696921242));
#32416=CARTESIAN_POINT('Ctrl Pts',(-0.195447439785316,-0.0191106540360297,
-1.41110832530195));
#32417=CARTESIAN_POINT('Ctrl Pts',(-0.192916081248045,-0.0380092915742028,
-1.41002968139147));
#32418=CARTESIAN_POINT('Ctrl Pts',(-0.1875227974271,-0.0560524670743356,
-1.40895103748099));
#32419=CARTESIAN_POINT('Ctrl Pts',(-0.16899293822269,-0.118043920281279,
-1.40524510980196));
#32420=CARTESIAN_POINT('Ctrl Pts',(-0.116680252802278,-0.169937302259617,
-1.40153918212294));
#32421=CARTESIAN_POINT('Ctrl Pts',(-0.0545417173908017,-0.187967740762588,
-1.39783325444391));
#32422=CARTESIAN_POINT('Ctrl Pts',(0.00759681802067429,-0.205998179265559,
-1.39412732676489));
#32423=CARTESIAN_POINT('Ctrl Pts',(0.0795612034232148,-0.190165674293162,
-1.39042139908587));
#32424=CARTESIAN_POINT('Ctrl Pts',(0.12839486296272,-0.147720799161269,
-1.38671547140684));
#32425=CARTESIAN_POINT('Ctrl Pts',(0.177228522502225,-0.105275924029376,
-1.38300954372782));
#32426=CARTESIAN_POINT('Ctrl Pts',(0.202931456178694,-0.0362186787379851,
-1.37930361604879));
#32427=CARTESIAN_POINT('Ctrl Pts',(0.193732822369028,0.0278256781203122,
-1.37559768836977));
#32428=CARTESIAN_POINT('Ctrl Pts',(0.184534188559362,0.0918700349786089,
-1.37189176069075));
#32429=CARTESIAN_POINT('Ctrl Pts',(0.140433987263561,0.150901503403812,
-1.36818583301172));
#32430=CARTESIAN_POINT('Ctrl Pts',(0.0816282130105867,0.177886223817467,
-1.3644799053327));
#32431=CARTESIAN_POINT('Ctrl Pts',(0.0228224387576129,0.204870944231122,
-1.36077397765367));
#32432=CARTESIAN_POINT('Ctrl Pts',(-0.0506889084525334,0.199808916633229,
-1.35706804997465));
#32433=CARTESIAN_POINT('Ctrl Pts',(-0.105240801513869,0.165018326909214,
-1.35336212229563));
#32434=CARTESIAN_POINT('Ctrl Pts',(-0.159792694575205,0.130227737185199,
-1.3496561946166));
#32435=CARTESIAN_POINT('Ctrl Pts',(-0.19538513348773,0.0657085853350611,
-1.34595026693758));
#32436=CARTESIAN_POINT('Ctrl Pts',(-0.195718314413653,0.00100786455706464,
-1.34224433925855));
#32437=CARTESIAN_POINT('Ctrl Pts',(-0.195720033695728,0.000673995536311298,
-1.34222521590984));
#32438=CARTESIAN_POINT('Ctrl Pts',(-0.195720814104094,0.000340121680791084,
-1.34220609256113));
#32439=CARTESIAN_POINT('Ctrl Pts',(-0.195720657836488,6.2470732444266E-6,
-1.34218696921242));
#32440=CARTESIAN_POINT('Origin',(0.,0.,-0.78));
#32441=CARTESIAN_POINT('',(-0.195298460177798,0.000172226659408109,-1.26201303078758));
#32442=CARTESIAN_POINT('',(-0.195270769970525,0.000166810798610398,-1.27218696921243));
#32443=CARTESIAN_POINT('',(-0.1954,-2.39295984553393E-17,-0.78));
#32444=CARTESIAN_POINT('Ctrl Pts',(-0.195298460177798,0.000172226659408109,
-1.26201303078758));
#32445=CARTESIAN_POINT('Ctrl Pts',(-0.195456041364949,0.018774870840142,
-1.26307258724242));
#32446=CARTESIAN_POINT('Ctrl Pts',(-0.193015100352074,0.0373369952455141,
-1.26413214369726));
#32447=CARTESIAN_POINT('Ctrl Pts',(-0.187808421048084,0.0550878746418882,
-1.26519170015211));
#32448=CARTESIAN_POINT('Ctrl Pts',(-0.16959742638116,0.117173736118483,
-1.26889762783113));
#32449=CARTESIAN_POINT('Ctrl Pts',(-0.117552165740612,0.169335347172546,
-1.27260355551016));
#32450=CARTESIAN_POINT('Ctrl Pts',(-0.0555071253652898,0.187684938084193,
-1.27630948318918));
#32451=CARTESIAN_POINT('Ctrl Pts',(0.00653791501003281,0.206034528995841,
-1.2800154108682));
#32452=CARTESIAN_POINT('Ctrl Pts',(0.07858273512013,0.190572099765074,-1.28372133854723));
#32453=CARTESIAN_POINT('Ctrl Pts',(0.127633912468266,0.148378776567857,
-1.28742726622625));
#32454=CARTESIAN_POINT('Ctrl Pts',(0.176685089816403,0.106185453370639,
-1.29113319390528));
#32455=CARTESIAN_POINT('Ctrl Pts',(0.202742624402578,0.0372612362069706,
-1.2948391215843));
#32456=CARTESIAN_POINT('Ctrl Pts',(0.193873288453785,-0.0268295541039423,
-1.29854504926333));
#32457=CARTESIAN_POINT('Ctrl Pts',(0.185003952504992,-0.0909203444148546,
-1.30225097694235));
#32458=CARTESIAN_POINT('Ctrl Pts',(0.14120774602123,-0.150177707873012,
-1.30595690462137));
#32459=CARTESIAN_POINT('Ctrl Pts',(0.082541443977279,-0.177464325937285,
-1.3096628323004));
#32460=CARTESIAN_POINT('Ctrl Pts',(0.0238751419333269,-0.204750944001557,
-1.31336875997942));
#32461=CARTESIAN_POINT('Ctrl Pts',(-0.0496612556708159,-0.200066816671946,
-1.31707468765845));
#32462=CARTESIAN_POINT('Ctrl Pts',(-0.104391248147666,-0.165557072481202,
-1.32078061533747));
#32463=CARTESIAN_POINT('Ctrl Pts',(-0.159121240624516,-0.131047328290458,
-1.32448654301649));
#32464=CARTESIAN_POINT('Ctrl Pts',(-0.195044827974074,-0.066711967238583,
-1.32819247069552));
#32465=CARTESIAN_POINT('Ctrl Pts',(-0.195710555453279,-0.00201381166068659,
-1.33189839837454));
#32466=CARTESIAN_POINT('Ctrl Pts',(-0.195717419586813,-0.00134672671505401,
-1.33193660917889));
#32467=CARTESIAN_POINT('Ctrl Pts',(-0.195720535419619,-0.000679603200347981,
-1.33197481998323));
#32468=CARTESIAN_POINT('Ctrl Pts',(-0.195719920316492,-1.24737763093352E-5,
-1.33201303078758));
#32469=CARTESIAN_POINT('Ctrl Pts',(-0.195720657836488,6.2470732444266E-6,
-1.34218696921242));
#32470=CARTESIAN_POINT('Ctrl Pts',(-0.195690530890782,-0.0643616817659535,
-1.33850016488211));
#32471=CARTESIAN_POINT('Ctrl Pts',(-0.160845783143528,-0.128757562123285,
-1.33481336055179));
#32472=CARTESIAN_POINT('Ctrl Pts',(-0.106934721662748,-0.163925713548613,
-1.33112655622148));
#32473=CARTESIAN_POINT('Ctrl Pts',(-0.0527440250466008,-0.199276281170437,
-1.32742062854246));
#32474=CARTESIAN_POINT('Ctrl Pts',(0.0207112911250145,-0.205095126708231,
-1.32371470086343));
#32475=CARTESIAN_POINT('Ctrl Pts',(0.0797918581805011,-0.178717469031425,
-1.32000877318441));
#32476=CARTESIAN_POINT('Ctrl Pts',(0.138872425235988,-0.152339811354619,
-1.31630284550538));
#32477=CARTESIAN_POINT('Ctrl Pts',(0.183578243175345,-0.0937656504632113,
-1.31259691782636));
#32478=CARTESIAN_POINT('Ctrl Pts',(0.19343597406848,-0.0298194278652247,
-1.30889099014733));
#32479=CARTESIAN_POINT('Ctrl Pts',(0.203293704961615,0.0341267947327626,
-1.30518506246831));
#32480=CARTESIAN_POINT('Ctrl Pts',(0.178303348808527,0.103445079037329,
-1.30147913478929));
#32481=CARTESIAN_POINT('Ctrl Pts',(0.129909411714146,0.146390638618789,
-1.29777320711026));
#32482=CARTESIAN_POINT('Ctrl Pts',(0.0815154746197661,0.189336198200248,
-1.29406727943124));
#32483=CARTESIAN_POINT('Ctrl Pts',(0.00971795658409383,0.205909033058599,
-1.29036135175221));
#32484=CARTESIAN_POINT('Ctrl Pts',(-0.0526029736186762,0.188519499016706,
-1.28665542407319));
#32485=CARTESIAN_POINT('Ctrl Pts',(-0.114923903821446,0.171129964974812,
-1.28294949639417));
#32486=CARTESIAN_POINT('Ctrl Pts',(-0.167768246191313,0.119778062032674,
-1.27924356871514));
#32487=CARTESIAN_POINT('Ctrl Pts',(-0.186935569481251,0.0579807485361383,
-1.27553764103612));
#32488=CARTESIAN_POINT('Ctrl Pts',(-0.192712207671533,0.039356305477451,
-1.27442075042822));
#32489=CARTESIAN_POINT('Ctrl Pts',(-0.195429975714095,0.0197831099638719,
-1.27330385982032));
#32490=CARTESIAN_POINT('Ctrl Pts',(-0.195270769970525,0.000166810798610398,
-1.27218696921243));
#32491=CARTESIAN_POINT('Origin',(0.,0.,-0.78));
#32492=CARTESIAN_POINT('',(-0.195114271280109,-8.4684676887617E-5,-1.19201303078758));
#32493=CARTESIAN_POINT('',(-0.19512853689889,-9.89862712037332E-5,-1.20218696921242));
#32494=CARTESIAN_POINT('',(-0.1954,-2.39295984553393E-17,-0.78));
#32495=CARTESIAN_POINT('Ctrl Pts',(-0.195114271280109,-8.4684676887617E-5,
-1.19201303078758));
#32496=CARTESIAN_POINT('Ctrl Pts',(-0.194966032011016,0.0378815244295202,
-1.19417035450161));
#32497=CARTESIAN_POINT('Ctrl Pts',(-0.184284351240505,0.0759248070606531,
-1.19632767821564));
#32498=CARTESIAN_POINT('Ctrl Pts',(-0.163614190118679,0.107410771065998,
-1.19848500192967));
#32499=CARTESIAN_POINT('Ctrl Pts',(-0.128106249547212,0.161498483887772,
-1.2021909296087));
#32500=CARTESIAN_POINT('Ctrl Pts',(-0.0631227082835343,0.196235815207334,
-1.20589685728772));
#32501=CARTESIAN_POINT('Ctrl Pts',(0.0015767725456126,0.195714564449213,
-1.20960278496675));
#32502=CARTESIAN_POINT('Ctrl Pts',(0.0662762533747604,0.195193313691093,
-1.21330871264577));
#32503=CARTESIAN_POINT('Ctrl Pts',(0.130691673769378,0.159413480855288,
-1.21701464032479));
#32504=CARTESIAN_POINT('Ctrl Pts',(0.165323547474987,0.104760687280339,
-1.22072056800382));
#32505=CARTESIAN_POINT('Ctrl Pts',(0.199955421180597,0.0501078937053893,
-1.22442649568284));
#32506=CARTESIAN_POINT('Ctrl Pts',(0.204803748197199,-0.0234178606087051,
-1.22813242336187));
#32507=CARTESIAN_POINT('Ctrl Pts',(0.177648203712596,-0.0821449491256642,
-1.23183835104089));
#32508=CARTESIAN_POINT('Ctrl Pts',(0.150492659227993,-0.140872037642623,
-1.23554427871991));
#32509=CARTESIAN_POINT('Ctrl Pts',(0.0913332432421869,-0.184800460362446,
-1.23925020639894));
#32510=CARTESIAN_POINT('Ctrl Pts',(0.0272624185229523,-0.193812892980807,
-1.24295613407796));
#32511=CARTESIAN_POINT('Ctrl Pts',(-0.0368084061962824,-0.202825325599168,
-1.24666206175699));
#32512=CARTESIAN_POINT('Ctrl Pts',(-0.105790639648945,-0.176921768116067,
-1.25036798943601));
#32513=CARTESIAN_POINT('Ctrl Pts',(-0.148093392028626,-0.127964933424953,
-1.25407391711504));
#32514=CARTESIAN_POINT('Ctrl Pts',(-0.178301425292436,-0.0930052769570597,
-1.25672028833922));
#32515=CARTESIAN_POINT('Ctrl Pts',(-0.194904881980768,-0.0462901416537951,
-1.2593666595634));
#32516=CARTESIAN_POINT('Ctrl Pts',(-0.195298460177798,0.000172226659408109,
-1.26201303078758));
#32517=CARTESIAN_POINT('Ctrl Pts',(-0.195270769970525,0.000166810798610398,
-1.27218696921243));
#32518=CARTESIAN_POINT('Ctrl Pts',(-0.194901718991742,-0.0453052572607288,
-1.2695979321413));
#32519=CARTESIAN_POINT('Ctrl Pts',(-0.179073320323297,-0.0910089417293884,
-1.26700889507017));
#32520=CARTESIAN_POINT('Ctrl Pts',(-0.150051297428642,-0.125663369668722,
-1.26441985799905));
#32521=CARTESIAN_POINT('Ctrl Pts',(-0.108509397876086,-0.175267450326114,
-1.26071393032002));
#32522=CARTESIAN_POINT('Ctrl Pts',(-0.0399352945609637,-0.202232887589962,
-1.257008002641));
#32523=CARTESIAN_POINT('Ctrl Pts',(0.0242670287275284,-0.194210673382068,
-1.25330207496197));
#32524=CARTESIAN_POINT('Ctrl Pts',(0.0884693520160203,-0.186188459174174,
-1.24959614728295));
#32525=CARTESIAN_POINT('Ctrl Pts',(0.148299895277882,-0.143178593494537,
-1.24589021960393));
#32526=CARTESIAN_POINT('Ctrl Pts',(0.176358848375927,-0.0848777411188696,
-1.2421842919249));
#32527=CARTESIAN_POINT('Ctrl Pts',(0.204417801473971,-0.0265768887432019,
-1.23847836424588));
#32528=CARTESIAN_POINT('Ctrl Pts',(0.200705164408199,0.0470149503284963,
-1.23477243656685));
#32529=CARTESIAN_POINT('Ctrl Pts',(0.166921164942484,0.102195885592478,
-1.23106650888783));
#32530=CARTESIAN_POINT('Ctrl Pts',(0.13313716547677,0.157376820856459,-1.2273605812088));
#32531=CARTESIAN_POINT('Ctrl Pts',(0.0692818036111139,0.194146852312723,
-1.22365465352978));
#32532=CARTESIAN_POINT('Ctrl Pts',(0.00459808293143662,0.195666890330114,
-1.21994872585076));
#32533=CARTESIAN_POINT('Ctrl Pts',(-0.0600856377482409,0.197186928347506,
-1.21624279817173));
#32534=CARTESIAN_POINT('Ctrl Pts',(-0.125597717241939,0.163456972926025,
-1.21253687049271));
#32535=CARTESIAN_POINT('Ctrl Pts',(-0.161936446693071,0.109923889898341,
-1.20883094281368));
#32536=CARTESIAN_POINT('Ctrl Pts',(-0.183652427151724,0.0779325846854268,
-1.2066162849466));
#32537=CARTESIAN_POINT('Ctrl Pts',(-0.194949895274585,0.0388691013047168,
-1.20440162707951));
#32538=CARTESIAN_POINT('Ctrl Pts',(-0.19512853689889,-9.89862712037332E-5,
-1.20218696921242));
#32539=CARTESIAN_POINT('Origin',(0.,0.,-0.78));
#32540=CARTESIAN_POINT('',(-0.195608501695121,-0.000129687756530023,-1.12201303078758));
#32541=CARTESIAN_POINT('',(-0.195632543296128,-0.000116579743955739,-1.13218696921242));
#32542=CARTESIAN_POINT('',(-0.1954,-2.39295984553393E-17,-0.78));
#32543=CARTESIAN_POINT('Ctrl Pts',(-0.195608501695121,-0.000129687756530023,
-1.12201303078758));
#32544=CARTESIAN_POINT('Ctrl Pts',(-0.195172766225982,0.0567872732702236,
-1.1252681217608));
#32545=CARTESIAN_POINT('Ctrl Pts',(-0.168902158860677,0.114054537459704,
-1.12852321273402));
#32546=CARTESIAN_POINT('Ctrl Pts',(-0.125226675603983,0.150415945518958,
-1.13177830370724));
#32547=CARTESIAN_POINT('Ctrl Pts',(-0.0755020492794521,0.191813482387723,
-1.13548423138626));
#32548=CARTESIAN_POINT('Ctrl Pts',(-0.00321745133242834,0.206113123012647,
-1.13919015906529));
#32549=CARTESIAN_POINT('Ctrl Pts',(0.0585238878228583,0.186766248297933,
-1.14289608674431));
#32550=CARTESIAN_POINT('Ctrl Pts',(0.120265226978144,0.16741937358322,-1.14660201442334));
#32551=CARTESIAN_POINT('Ctrl Pts',(0.171463307341694,0.114425983528869,
-1.15030794210236));
#32552=CARTESIAN_POINT('Ctrl Pts',(0.188671614729629,0.052054766779819,
-1.15401386978138));
#32553=CARTESIAN_POINT('Ctrl Pts',(0.205879922117565,-0.0103164499692322,
-1.15771979746041));
#32554=CARTESIAN_POINT('Ctrl Pts',(0.189098456529886,-0.0820654934129837,
-1.16142572513943));
#32555=CARTESIAN_POINT('Ctrl Pts',(0.146012405929378,-0.13033439401747,
-1.16513165281846));
#32556=CARTESIAN_POINT('Ctrl Pts',(0.10292635532887,-0.178603294621956,
-1.16883758049748));
#32557=CARTESIAN_POINT('Ctrl Pts',(0.0335357197155342,-0.203392052387178,
-1.1725435081765));
#32558=CARTESIAN_POINT('Ctrl Pts',(-0.0303815805162766,-0.193348484645014,
-1.17624943585553));
#32559=CARTESIAN_POINT('Ctrl Pts',(-0.0942988807480878,-0.183304916902849,
-1.17995536353455));
#32560=CARTESIAN_POINT('Ctrl Pts',(-0.152742845598374,-0.138429023653299,
-1.18366129121358));
#32561=CARTESIAN_POINT('Ctrl Pts',(-0.178948658083888,-0.0792720298665307,
-1.1873672188926));
#32562=CARTESIAN_POINT('Ctrl Pts',(-0.189899337275662,-0.0545519697170222,
-1.18891582285759));
#32563=CARTESIAN_POINT('Ctrl Pts',(-0.195220682718685,-0.0273381847313685,
-1.19046442682259));
#32564=CARTESIAN_POINT('Ctrl Pts',(-0.195114271280109,-8.4684676887617E-5,
-1.19201303078758));
#32565=CARTESIAN_POINT('Ctrl Pts',(-0.19512853689889,-9.89862712037332E-5,
-1.20218696921242));
#32566=CARTESIAN_POINT('Ctrl Pts',(-0.195248827651444,-0.026338674800327,
-1.20069569940049));
#32567=CARTESIAN_POINT('Ctrl Pts',(-0.190327637582909,-0.0525351091137002,
-1.19920442958855));
#32568=CARTESIAN_POINT('Ctrl Pts',(-0.180151149975641,-0.0764999183032752,
-1.19771315977661));
#32569=CARTESIAN_POINT('Ctrl Pts',(-0.154861744398516,-0.136054432843319,
-1.19400723209759));
#32570=CARTESIAN_POINT('Ctrl Pts',(-0.0971175538357005,-0.181827251289521,
-1.19030130441856));
#32571=CARTESIAN_POINT('Ctrl Pts',(-0.0333629288067565,-0.192856395588613,
-1.18659537673954));
#32572=CARTESIAN_POINT('Ctrl Pts',(0.0303916962221866,-0.203885539887706,
-1.18288944906052));
#32573=CARTESIAN_POINT('Ctrl Pts',(0.100156755717259,-0.180171010039691,
-1.17918352138149));
#32574=CARTESIAN_POINT('Ctrl Pts',(0.143982859283783,-0.132573038625658,
-1.17547759370247));
#32575=CARTESIAN_POINT('Ctrl Pts',(0.187808962850309,-0.0849750672116236,
-1.17177166602344));
#32576=CARTESIAN_POINT('Ctrl Pts',(0.205696110488285,-0.0134936542315703,
-1.16806573834442));
#32577=CARTESIAN_POINT('Ctrl Pts',(0.189452759510499,0.049135793998185,
-1.16435981066539));
#32578=CARTESIAN_POINT('Ctrl Pts',(0.173209408532712,0.11176524222794,-1.16065388298637));
#32579=CARTESIAN_POINT('Ctrl Pts',(0.122835558939162,0.165542725707396,
-1.15694795530735));
#32580=CARTESIAN_POINT('Ctrl Pts',(0.0614002627451628,0.185840474797084,
-1.15324202762832));
#32581=CARTESIAN_POINT('Ctrl Pts',(-3.50334488365758E-5,0.206138223886772,
-1.1495360999493));
#32582=CARTESIAN_POINT('Ctrl Pts',(-0.0725317762432855,0.192956238586691,
-1.14583017227027));
#32583=CARTESIAN_POINT('Ctrl Pts',(-0.122889582027208,0.152331300024504,
-1.14212424459125));
#32584=CARTESIAN_POINT('Ctrl Pts',(-0.167900298811259,0.116019995837856,
-1.13881181946497));
#32585=CARTESIAN_POINT('Ctrl Pts',(-0.195223980988476,0.0577842214822079,
-1.1354993943387));
#32586=CARTESIAN_POINT('Ctrl Pts',(-0.195632543296128,-0.000116579743955739,
-1.13218696921242));
#32587=CARTESIAN_POINT('Origin',(0.,0.,-0.78));
#32588=CARTESIAN_POINT('',(-0.195514202958888,0.000163480152566932,-1.05201303078758));
#32589=CARTESIAN_POINT('',(-0.195484338171094,0.0001698553111729,-1.06218696921242));
#32590=CARTESIAN_POINT('',(-0.1954,-2.39295984553393E-17,-0.78));
#32591=CARTESIAN_POINT('Ctrl Pts',(-0.195514202958888,0.000163480152566932,
-1.05201303078758));
#32592=CARTESIAN_POINT('Ctrl Pts',(-0.195615708286294,0.0114895985054695,
-1.05265996134096));
#32593=CARTESIAN_POINT('Ctrl Pts',(-0.194716269514434,0.0227996078840509,
-1.05330689189435));
#32594=CARTESIAN_POINT('Ctrl Pts',(-0.192758608403307,0.0339233818421437,
-1.05395382244773));
#32595=CARTESIAN_POINT('Ctrl Pts',(-0.181544189081305,0.0976456803033987,
-1.05765975012676));
#32596=CARTESIAN_POINT('Ctrl Pts',(-0.135603712275178,0.15525657695664,
-1.06136567780578));
#32597=CARTESIAN_POINT('Ctrl Pts',(-0.0759759363407144,0.180372764147859,
-1.0650716054848));
#32598=CARTESIAN_POINT('Ctrl Pts',(-0.0163481604062512,0.205488951339078,
-1.06877753316383));
#32599=CARTESIAN_POINT('Ctrl Pts',(0.0569669146565482,0.198110429068274,
-1.07248346084285));
#32600=CARTESIAN_POINT('Ctrl Pts',(0.110394144327698,0.161616242523277,
-1.07618938852188));
#32601=CARTESIAN_POINT('Ctrl Pts',(0.163821373998849,0.125122055978279,
-1.0798953162009));
#32602=CARTESIAN_POINT('Ctrl Pts',(0.197360758278349,0.0595122051590866,
-1.08360124387992));
#32603=CARTESIAN_POINT('Ctrl Pts',(0.195652704704064,-0.00516682602492472,
-1.08730717155895));
#32604=CARTESIAN_POINT('Ctrl Pts',(0.193944651129778,-0.0698458572089361,
-1.09101309923797));
#32605=CARTESIAN_POINT('Ctrl Pts',(0.156989159701705,-0.133594068757766,
-1.094719026917));
#32606=CARTESIAN_POINT('Ctrl Pts',(0.101710252722787,-0.167217527311745,
-1.09842495459602));
#32607=CARTESIAN_POINT('Ctrl Pts',(0.0464313457438697,-0.200840985865723,
-1.10213088227505));
#32608=CARTESIAN_POINT('Ctrl Pts',(-0.0271709767858934,-0.20433969142485,
-1.10583680995407));
#32609=CARTESIAN_POINT('Ctrl Pts',(-0.0853900233869303,-0.176111387636254,
-1.10954273763309));
#32610=CARTESIAN_POINT('Ctrl Pts',(-0.143609069987967,-0.147883083847658,
-1.11324866531212));
#32611=CARTESIAN_POINT('Ctrl Pts',(-0.186444840660277,-0.0879277707113403,
-1.11695459299114));
#32612=CARTESIAN_POINT('Ctrl Pts',(-0.194280398645414,-0.0237023975868779,
-1.12066052067017));
#32613=CARTESIAN_POINT('Ctrl Pts',(-0.195233616693933,-0.0158891971803149,
-1.12111135737597));
#32614=CARTESIAN_POINT('Ctrl Pts',(-0.195668851941896,-0.0080128023683071,
-1.12156219408177));
#32615=CARTESIAN_POINT('Ctrl Pts',(-0.195608501695121,-0.000129687756530023,
-1.12201303078758));
#32616=CARTESIAN_POINT('Ctrl Pts',(-0.195632543296128,-0.000116579743955739,
-1.13218696921242));
#32617=CARTESIAN_POINT('Ctrl Pts',(-0.19568107882671,-0.00699495803785087,
-1.13179346665968));
#32618=CARTESIAN_POINT('Ctrl Pts',(-0.195349775591712,-0.0138686090342038,
-1.13139996410693));
#32619=CARTESIAN_POINT('Ctrl Pts',(-0.19462316267436,-0.0207002146995433,
-1.13100646155418));
#32620=CARTESIAN_POINT('Ctrl Pts',(-0.187780068764195,-0.0850388990371081,
-1.12730053387515));
#32621=CARTESIAN_POINT('Ctrl Pts',(-0.145875012170469,-0.145648375887944,
-1.12359460619613));
#32622=CARTESIAN_POINT('Ctrl Pts',(-0.0880987027171473,-0.174772117105487,
-1.11988867851711));
#32623=CARTESIAN_POINT('Ctrl Pts',(-0.0303223932638255,-0.20389585832303,
-1.11618275083808));
#32624=CARTESIAN_POINT('Ctrl Pts',(0.0433251690490918,-0.20153386390728,
-1.11247682315906));
#32625=CARTESIAN_POINT('Ctrl Pts',(0.0991165748711698,-0.168767825499369,
-1.10877089548003));
#32626=CARTESIAN_POINT('Ctrl Pts',(0.154907980693247,-0.136001787091459,
-1.10506496780101));
#32627=CARTESIAN_POINT('Ctrl Pts',(0.192843230024486,-0.0728317046913883,
-1.10135904012198));
#32628=CARTESIAN_POINT('Ctrl Pts',(0.195549613669579,-0.00818675342589603,
-1.09765311244296));
#32629=CARTESIAN_POINT('Ctrl Pts',(0.198255997314672,0.0564581978395958,
-1.09394718476394));
#32630=CARTESIAN_POINT('Ctrl Pts',(0.165733515273621,0.122578017970509,
-1.09024125708491));
#32631=CARTESIAN_POINT('Ctrl Pts',(0.112876062611548,0.159892679092233,
-1.08653532940589));
#32632=CARTESIAN_POINT('Ctrl Pts',(0.060018609949475,0.197207340213956,
-1.08282940172686));
#32633=CARTESIAN_POINT('Ctrl Pts',(-0.0131738133336202,0.205716842326488,
-1.07912347404784));
#32634=CARTESIAN_POINT('Ctrl Pts',(-0.0731822319466,0.181524200219397,-1.07541754636881));
#32635=CARTESIAN_POINT('Ctrl Pts',(-0.133190650559579,0.157331558112307,
-1.07171161868979));
#32636=CARTESIAN_POINT('Ctrl Pts',(-0.180015064502443,0.100436771785593,
-1.06800569101077));
#32637=CARTESIAN_POINT('Ctrl Pts',(-0.192211910308214,0.0368952012278665,
-1.06429976333174));
#32638=CARTESIAN_POINT('Ctrl Pts',(-0.194529766665614,0.0248199290122665,
-1.0635954986253));
#32639=CARTESIAN_POINT('Ctrl Pts',(-0.195597076185699,0.012504613517696,
-1.06289123391886));
#32640=CARTESIAN_POINT('Ctrl Pts',(-0.195484338171094,0.0001698553111729,
-1.06218696921242));
#32641=CARTESIAN_POINT('Origin',(0.,0.,-0.78));
#32642=CARTESIAN_POINT('',(-0.195083431151666,3.11826631982926E-5,-0.982013030787577));
#32643=CARTESIAN_POINT('',(-0.19507989431385,1.47260064652817E-5,-0.992186969212424));
#32644=CARTESIAN_POINT('',(-0.1954,-2.39295984553393E-17,-0.78));
#32645=CARTESIAN_POINT('Ctrl Pts',(-0.195083431151666,3.11826631982926E-5,
-0.982013030787577));
#32646=CARTESIAN_POINT('Ctrl Pts',(-0.195127180458594,0.0307478132193151,
-0.98375772860015));
#32647=CARTESIAN_POINT('Ctrl Pts',(-0.188305349657826,0.0614460671203186,
-0.985502426412724));
#32648=CARTESIAN_POINT('Ctrl Pts',(-0.174515300359914,0.0886063591932106,
-0.987247124225297));
#32649=CARTESIAN_POINT('Ctrl Pts',(-0.145223737649203,0.14629776995668,
-0.990953051904321));
#32650=CARTESIAN_POINT('Ctrl Pts',(-0.0844927056335577,0.188026471981535,
-0.994658979583346));
#32651=CARTESIAN_POINT('Ctrl Pts',(-0.0201343994860245,0.194682518235522,
-0.99836490726237));
#32652=CARTESIAN_POINT('Ctrl Pts',(0.0442239066615097,0.201338564489509,
-1.00207083494139));
#32653=CARTESIAN_POINT('Ctrl Pts',(0.112209486940932,0.172921954972627,
-1.00577676262042));
#32654=CARTESIAN_POINT('Ctrl Pts',(0.152687875743341,0.12244627209586,-1.00948269029944));
#32655=CARTESIAN_POINT('Ctrl Pts',(0.19316626454575,0.0719705892190932,
-1.01318861797847));
#32656=CARTESIAN_POINT('Ctrl Pts',(0.206137461871147,-0.000564167017557592,
-1.01689454565749));
#32657=CARTESIAN_POINT('Ctrl Pts',(0.185661218399396,-0.0619402044849644,
-1.02060047333651));
#32658=CARTESIAN_POINT('Ctrl Pts',(0.165184974927645,-0.123316241952371,
-1.02430640101554));
#32659=CARTESIAN_POINT('Ctrl Pts',(0.111261290658746,-0.173533560650533,
-1.02801232869456));
#32660=CARTESIAN_POINT('Ctrl Pts',(0.0485848888924792,-0.189594792967773,
-1.03171825637359));
#32661=CARTESIAN_POINT('Ctrl Pts',(-0.0140915128737879,-0.205656025285014,
-1.03542418405261));
#32662=CARTESIAN_POINT('Ctrl Pts',(-0.0855206321374236,-0.187561171221331,
-1.03913011173164));
#32663=CARTESIAN_POINT('Ctrl Pts',(-0.132991010850304,-0.143596894054857,
-1.04283603941066));
#32664=CARTESIAN_POINT('Ctrl Pts',(-0.172174655166304,-0.107307303665854,
-1.0458950365363));
#32665=CARTESIAN_POINT('Ctrl Pts',(-0.195034237214269,-0.053391825443827,
-1.04895403366194));
#32666=CARTESIAN_POINT('Ctrl Pts',(-0.195514202958888,0.000163480152566932,
-1.05201303078758));
#32667=CARTESIAN_POINT('Ctrl Pts',(-0.195484338171094,0.0001698553111729,
-1.06218696921242));
#32668=CARTESIAN_POINT('Ctrl Pts',(-0.195003834858986,-0.0524024043033798,
-1.05918530623984));
#32669=CARTESIAN_POINT('Ctrl Pts',(-0.173086948518685,-0.105327854283802,
-1.05618364326725));
#32670=CARTESIAN_POINT('Ctrl Pts',(-0.135192047384276,-0.141526621743139,
-1.05318198029467));
#32671=CARTESIAN_POINT('Ctrl Pts',(-0.088406060985887,-0.186218519367677,
-1.04947605261565));
#32672=CARTESIAN_POINT('Ctrl Pts',(-0.0172648105204307,-0.205413959828011,
-1.04577012493662));
#32673=CARTESIAN_POINT('Ctrl Pts',(0.0456520774664714,-0.190322258711306,
-1.0420641972576));
#32674=CARTESIAN_POINT('Ctrl Pts',(0.108568965453373,-0.1752305575946,-1.03835826957857));
#32675=CARTESIAN_POINT('Ctrl Pts',(0.163261490961722,-0.125851714900854,
-1.03465234189955));
#32676=CARTESIAN_POINT('Ctrl Pts',(0.184682834540907,-0.0647991123697999,
-1.03094641422053));
#32677=CARTESIAN_POINT('Ctrl Pts',(0.206104178120092,-0.00374650983874577,
-1.0272404865415));
#32678=CARTESIAN_POINT('Ctrl Pts',(0.194254339770113,0.068979852529617,
-1.02353455886248));
#32679=CARTESIAN_POINT('Ctrl Pts',(0.154560034730616,0.120074435256005,
-1.01982863118345));
#32680=CARTESIAN_POINT('Ctrl Pts',(0.114865729691119,0.171169017982394,
-1.01612270350443));
#32681=CARTESIAN_POINT('Ctrl Pts',(0.0473269579621042,0.200631821066808,
-1.0124167758254));
#32682=CARTESIAN_POINT('Ctrl Pts',(-0.0171264339062948,0.194970150534976,
-1.00871084814638));
#32683=CARTESIAN_POINT('Ctrl Pts',(-0.0815798257746925,0.189308480003144,
-1.00500492046736));
#32684=CARTESIAN_POINT('Ctrl Pts',(-0.142947837782473,0.148522335855069,
-1.00129899278833));
#32685=CARTESIAN_POINT('Ctrl Pts',(-0.173126565373849,0.091290014239414,
-0.997593065109308));
#32686=CARTESIAN_POINT('Ctrl Pts',(-0.187801172250139,0.0634604174552492,
-0.99579103314368));
#32687=CARTESIAN_POINT('Ctrl Pts',(-0.195101212356669,0.0317421955836092,
-0.993989001178052));
#32688=CARTESIAN_POINT('Ctrl Pts',(-0.19507989431385,1.47260064652817E-5,
-0.992186969212424));
#32689=CARTESIAN_POINT('Origin',(0.,0.,-0.78));
#32690=CARTESIAN_POINT('',(-0.195399668261945,-0.000178796749683685,-0.912013030787577));
#32691=CARTESIAN_POINT('',(-0.195430231275111,-0.000177069784595039,-0.922186969212424));
#32692=CARTESIAN_POINT('',(-0.1954,-2.39295984553393E-17,-0.78));
#32693=CARTESIAN_POINT('Ctrl Pts',(-0.195399668261945,-0.000178796749683685,
-0.912013030787577));
#32694=CARTESIAN_POINT('Ctrl Pts',(-0.1949414362207,0.0496606202826749,
-0.914855495859339));
#32695=CARTESIAN_POINT('Ctrl Pts',(-0.175516129708998,0.099817575153293,
-0.917697960931101));
#32696=CARTESIAN_POINT('Ctrl Pts',(-0.141133053901595,0.135602868869345,
-0.920540426002863));
#32697=CARTESIAN_POINT('Ctrl Pts',(-0.0963053465744313,0.182258749288699,
-0.924246353681887));
#32698=CARTESIAN_POINT('Ctrl Pts',(-0.0260520845428951,0.20448535488409,
-0.927952281360912));
#32699=CARTESIAN_POINT('Ctrl Pts',(0.0374537660780799,0.192103858253175,
-0.931658209039936));
#32700=CARTESIAN_POINT('Ctrl Pts',(0.100959616699055,0.17972236162226,-0.93536413671896));
#32701=CARTESIAN_POINT('Ctrl Pts',(0.157718055909468,0.132732762765039,
-0.939070064397983));
#32702=CARTESIAN_POINT('Ctrl Pts',(0.181736164823455,0.0726542727198421,
-0.942775992077008));
#32703=CARTESIAN_POINT('Ctrl Pts',(0.205754273737442,0.0125757826746453,
-0.946481919756032));
#32704=CARTESIAN_POINT('Ctrl Pts',(0.197032052355003,-0.0605915985585276,
-0.950187847435057));
#32705=CARTESIAN_POINT('Ctrl Pts',(0.159563902144046,-0.113340363868098,
-0.953893775114081));
#32706=CARTESIAN_POINT('Ctrl Pts',(0.122095751933089,-0.166089129177668,
-0.957599702793105));
#32707=CARTESIAN_POINT('Ctrl Pts',(0.0558816728936141,-0.198419278563635,
-0.961305630472128));
#32708=CARTESIAN_POINT('Ctrl Pts',(-0.00875514058217604,-0.195524997027423,
-0.965011558151153));
#32709=CARTESIAN_POINT('Ctrl Pts',(-0.0733919540579662,-0.19263071549121,
-0.968717485830177));
#32710=CARTESIAN_POINT('Ctrl Pts',(-0.136451501970072,-0.154512003032818,
-0.972423413509202));
#32711=CARTESIAN_POINT('Ctrl Pts',(-0.169055229223237,-0.0986255870525807,
-0.976129341188226));
#32712=CARTESIAN_POINT('Ctrl Pts',(-0.186309587425756,-0.0690496973854128,
-0.978090571054676));
#32713=CARTESIAN_POINT('Ctrl Pts',(-0.195034252178227,-0.0344976468047085,
-0.980051800921127));
#32714=CARTESIAN_POINT('Ctrl Pts',(-0.195083431151666,3.11826631982926E-5,
-0.982013030787577));
#32715=CARTESIAN_POINT('Ctrl Pts',(-0.19507989431385,1.47260064652817E-5,
-0.992186969212424));
#32716=CARTESIAN_POINT('Ctrl Pts',(-0.195057371222631,-0.0335062072938361,
-0.990283073499028));
#32717=CARTESIAN_POINT('Ctrl Pts',(-0.186862384746915,-0.067037463342061,
-0.988379177785632));
#32718=CARTESIAN_POINT('Ctrl Pts',(-0.17055768636991,-0.0960039059524206,
-0.986475282072236));
#32719=CARTESIAN_POINT('Ctrl Pts',(-0.138820636599626,-0.152387005445362,
-0.982769354393212));
#32720=CARTESIAN_POINT('Ctrl Pts',(-0.0763570938840897,-0.191474705348008,
-0.979063426714187));
#32721=CARTESIAN_POINT('Ctrl Pts',(-0.011772668626182,-0.195366523773639,
-0.975357499035163));
#32722=CARTESIAN_POINT('Ctrl Pts',(0.0528117566317258,-0.19925834219927,
-0.971651571356139));
#32723=CARTESIAN_POINT('Ctrl Pts',(0.119517064432005,-0.167954279147886,
-0.967945643677115));
#32724=CARTESIAN_POINT('Ctrl Pts',(0.157795098781825,-0.115790246300853,
-0.964239715998091));
#32725=CARTESIAN_POINT('Ctrl Pts',(0.196073133131644,-0.0636262134538189,
-0.960533788319067));
#32726=CARTESIAN_POINT('Ctrl Pts',(0.205923894031003,0.00939778918886471,
-0.956827860640042));
#32727=CARTESIAN_POINT('Ctrl Pts',(0.182836157552975,0.0698399157304871,
-0.953121932961018));
#32728=CARTESIAN_POINT('Ctrl Pts',(0.159748421074947,0.13028204227211,-0.949416005281994));
#32729=CARTESIAN_POINT('Ctrl Pts',(0.103722187219531,0.178142292712671,
-0.945710077602971));
#32730=CARTESIAN_POINT('Ctrl Pts',(0.0404150563778447,0.191502735113506,
-0.942004149923947));
#32731=CARTESIAN_POINT('Ctrl Pts',(-0.0228920744638412,0.20486317751434,
-0.938298222244923));
#32732=CARTESIAN_POINT('Ctrl Pts',(-0.0934801022917972,0.183723811875449,
-0.934592294565898));
#32733=CARTESIAN_POINT('Ctrl Pts',(-0.139022752684639,0.137765556558828,
-0.930886366886874));
#32734=CARTESIAN_POINT('Ctrl Pts',(-0.174658780622462,0.101804327769778,
-0.927986567662057));
#32735=CARTESIAN_POINT('Ctrl Pts',(-0.194960310669972,0.0506472724299381,
-0.925086768437241));
#32736=CARTESIAN_POINT('Ctrl Pts',(-0.195430231275111,-0.000177069784595039,
-0.922186969212424));
#32737=CARTESIAN_POINT('Origin',(0.,0.,-0.78));
#32738=CARTESIAN_POINT('',(-0.195686871268044,7.38626216447175E-5,-0.842013030787577));
#32739=CARTESIAN_POINT('',(-0.195669687271611,9.02064299060124E-5,-0.852186969212425));
#32740=CARTESIAN_POINT('',(-0.1954,-2.39295984553393E-17,-0.78));
#32741=CARTESIAN_POINT('Ctrl Pts',(-0.195686871268044,7.38626216447175E-5,
-0.842013030787577));
#32742=CARTESIAN_POINT('Ctrl Pts',(-0.195706672219619,0.00416647744429093,
-0.842247335439503));
#32743=CARTESIAN_POINT('Ctrl Pts',(-0.195589410136118,0.00825793637018049,
-0.84248164009143));
#32744=CARTESIAN_POINT('Ctrl Pts',(-0.195331484399924,0.0123405085514971,
-0.842715944743357));
#32745=CARTESIAN_POINT('Ctrl Pts',(-0.191251948987234,0.0769133504645765,
-0.846421872422381));
#32746=CARTESIAN_POINT('Ctrl Pts',(-0.151982844548713,0.139263011722367,
-0.850127800101405));
#32747=CARTESIAN_POINT('Ctrl Pts',(-0.0955077284300276,0.170836034721377,
-0.853833727780429));
#32748=CARTESIAN_POINT('Ctrl Pts',(-0.0390326123113426,0.202409057720386,
-0.857539655459453));
#32749=CARTESIAN_POINT('Ctrl Pts',(0.0346485154875061,0.203205442460615,
-0.861245583138477));
#32750=CARTESIAN_POINT('Ctrl Pts',(0.0917928740701902,0.172860479054993,
-0.864951510817501));
#32751=CARTESIAN_POINT('Ctrl Pts',(0.148937232652874,0.142515515649371,
-0.868657438496525));
#32752=CARTESIAN_POINT('Ctrl Pts',(0.189544822019393,0.0810292040978983,
-0.872363366175549));
#32753=CARTESIAN_POINT('Ctrl Pts',(0.195019116415376,0.0165596250486992,
-0.876069293854573));
#32754=CARTESIAN_POINT('Ctrl Pts',(0.200493410811359,-0.0479099540005018,
-0.879775221533598));
#32755=CARTESIAN_POINT('Ctrl Pts',(0.170834410236803,-0.11536280054743,
-0.883481149212622));
#32756=CARTESIAN_POINT('Ctrl Pts',(0.11962465866041,-0.154908418071994,
-0.887187076891646));
#32757=CARTESIAN_POINT('Ctrl Pts',(0.0684149070840171,-0.194454035596558,
-0.89089300457067));
#32758=CARTESIAN_POINT('Ctrl Pts',(-0.00434559549421255,-0.206092424098759,
-0.894598932249694));
#32759=CARTESIAN_POINT('Ctrl Pts',(-0.0653356748503108,-0.184493703255807,
-0.898304859928718));
#32760=CARTESIAN_POINT('Ctrl Pts',(-0.126325754206408,-0.162894982412855,
-0.902010787607742));
#32761=CARTESIAN_POINT('Ctrl Pts',(-0.175545410340374,-0.10805915222475,
-0.905716715286767));
#32762=CARTESIAN_POINT('Ctrl Pts',(-0.190454162095962,-0.0450986595090393,
-0.909422642965791));
#32763=CARTESIAN_POINT('Ctrl Pts',(-0.193927826661724,-0.030429179717916,
-0.910286105573053));
#32764=CARTESIAN_POINT('Ctrl Pts',(-0.195538866536356,-0.0153186390656704,
-0.911149568180315));
#32765=CARTESIAN_POINT('Ctrl Pts',(-0.195399668261945,-0.000178796749683685,
-0.912013030787577));
#32766=CARTESIAN_POINT('Ctrl Pts',(-0.195430231275111,-0.000177069784595039,
-0.922186969212424));
#32767=CARTESIAN_POINT('Ctrl Pts',(-0.195560866654202,-0.0143059612177976,
-0.921380840758217));
#32768=CARTESIAN_POINT('Ctrl Pts',(-0.194158895742392,-0.0284091402533054,
-0.920574712304009));
#32769=CARTESIAN_POINT('Ctrl Pts',(-0.191127703969788,-0.0421529964915287,
-0.919768583849801));
#32770=CARTESIAN_POINT('Ctrl Pts',(-0.177192731904368,-0.105336149230912,
-0.916062656170777));
#32771=CARTESIAN_POINT('Ctrl Pts',(-0.1288255148158,-0.160925309715328,
-0.912356728491753));
#32772=CARTESIAN_POINT('Ctrl Pts',(-0.0681761535174188,-0.18346303831984,
-0.908650800812729));
#32773=CARTESIAN_POINT('Ctrl Pts',(-0.00752679221903582,-0.206000766924353,
-0.904944873133705));
#32774=CARTESIAN_POINT('Ctrl Pts',(0.0654047132891616,-0.195487063648961,
-0.901238945454681));
#32775=CARTESIAN_POINT('Ctrl Pts',(0.117218876811456,-0.156736751456187,
-0.897533017775657));
#32776=CARTESIAN_POINT('Ctrl Pts',(0.169033040333749,-0.117986439263414,
-0.893827090096633));
#32777=CARTESIAN_POINT('Ctrl Pts',(0.19972986187014,-0.0509995181532625,
-0.890121162417608));
#32778=CARTESIAN_POINT('Ctrl Pts',(0.195251520181195,0.0135468891229706,
-0.886415234738584));
#32779=CARTESIAN_POINT('Ctrl Pts',(0.190773178492251,0.0780932963992041,
-0.88270930705956));
#32780=CARTESIAN_POINT('Ctrl Pts',(0.15111967357797,0.140199189841518,-0.879003379380536));
#32781=CARTESIAN_POINT('Ctrl Pts',(0.0944506016343666,0.171422746999586,
-0.875297451701512));
#32782=CARTESIAN_POINT('Ctrl Pts',(0.0377815296907636,0.202646304157653,
-0.871591524022488));
#32783=CARTESIAN_POINT('Ctrl Pts',(-0.0359031092821614,0.202987525031474,
-0.867885596343463));
#32784=CARTESIAN_POINT('Ctrl Pts',(-0.0928589264216835,0.172290145167361,
-0.864179668664439));
#32785=CARTESIAN_POINT('Ctrl Pts',(-0.149814743561206,0.141592765303247,
-0.860473740985415));
#32786=CARTESIAN_POINT('Ctrl Pts',(-0.190041738867325,0.079856784701199,
-0.856767813306392));
#32787=CARTESIAN_POINT('Ctrl Pts',(-0.195117682261837,0.0153546216738394,
-0.853061885627368));
#32788=CARTESIAN_POINT('Ctrl Pts',(-0.195517134759009,0.0102786095728853,
-0.852770246822387));
#32789=CARTESIAN_POINT('Ctrl Pts',(-0.195698898966946,0.00518546667535099,
-0.852478608017406));
#32790=CARTESIAN_POINT('Ctrl Pts',(-0.195669687271611,9.02064299060124E-5,
-0.852186969212425));
#32791=CARTESIAN_POINT('Origin',(0.,0.,-0.78));
#32792=CARTESIAN_POINT('',(-0.195179502128291,0.000133953588564106,-0.772013030787577));
#32793=CARTESIAN_POINT('',(-0.195159317916871,0.00012225950549708,-0.782186969212424));
#32794=CARTESIAN_POINT('',(-0.1954,-2.39295984553393E-17,-0.78));
#32795=CARTESIAN_POINT('Ctrl Pts',(-0.195179502128291,0.000133953588564106,
-0.772013030787577));
#32796=CARTESIAN_POINT('Ctrl Pts',(-0.195327243613688,0.0235571326323705,
-0.773345102698692));
#32797=CARTESIAN_POINT('Ctrl Pts',(-0.19142847176856,0.0469327719984332,
-0.774677174609807));
#32798=CARTESIAN_POINT('Ctrl Pts',(-0.183264095800439,0.0687091561557484,
-0.776009246520923));
#32799=CARTESIAN_POINT('Ctrl Pts',(-0.160550166747699,0.129292750873312,
-0.779715174199947));
#32800=CARTESIAN_POINT('Ctrl Pts',(-0.104820645923167,0.177498179312782,
-0.783421101878971));
#32801=CARTESIAN_POINT('Ctrl Pts',(-0.0415972519380625,0.191249432889064,
-0.787127029557995));
#32802=CARTESIAN_POINT('Ctrl Pts',(0.021626142047042,0.205000686465347,
-0.790832957237019));
#32803=CARTESIAN_POINT('Ctrl Pts',(0.0923434091927182,0.184297765178443,
-0.794538884916043));
#32804=CARTESIAN_POINT('Ctrl Pts',(0.138169089040245,0.138621714687765,
-0.798244812595067));
#32805=CARTESIAN_POINT('Ctrl Pts',(0.183994768887772,0.0929456641970873,
-0.801950740274091));
#32806=CARTESIAN_POINT('Ctrl Pts',(0.204928861437148,0.0222964845026362,
-0.805656667953116));
#32807=CARTESIAN_POINT('Ctrl Pts',(0.191384454554165,-0.0409715450549779,
-0.80936259563214));
#32808=CARTESIAN_POINT('Ctrl Pts',(0.177840047671182,-0.104239574612591,
-0.813068523311164));
#32809=CARTESIAN_POINT('Ctrl Pts',(0.129817141355837,-0.160126454033369,
-0.816774450990188));
#32810=CARTESIAN_POINT('Ctrl Pts',(0.069308156927028,-0.183038401251119,
-0.820480378669212));
#32811=CARTESIAN_POINT('Ctrl Pts',(0.00879917249821865,-0.20595034846887,
-0.824186306348236));
#32812=CARTESIAN_POINT('Ctrl Pts',(-0.0641958900440562,-0.195887363483594,
-0.82789223402726));
#32813=CARTESIAN_POINT('Ctrl Pts',(-0.116248438121764,-0.157457859706773,
-0.831598161706284));
#32814=CARTESIAN_POINT('Ctrl Pts',(-0.165010000725506,-0.121458034079663,
-0.835069784733382));
#32815=CARTESIAN_POINT('Ctrl Pts',(-0.19539348639974,-0.060565205969237,
-0.838541407760479));
#32816=CARTESIAN_POINT('Ctrl Pts',(-0.195686871268044,7.38626216447175E-5,
-0.842013030787577));
#32817=CARTESIAN_POINT('Ctrl Pts',(-0.195669687271611,9.02064299060124E-5,
-0.852186969212425));
#32818=CARTESIAN_POINT('Ctrl Pts',(-0.195327698603891,-0.0595612873674038,
-0.848772680338381));
#32819=CARTESIAN_POINT('Ctrl Pts',(-0.166069407350001,-0.119502984320218,
-0.845358391464337));
#32820=CARTESIAN_POINT('Ctrl Pts',(-0.1186654601828,-0.15564441171331,-0.841944102590294));
#32821=CARTESIAN_POINT('Ctrl Pts',(-0.0672124032263472,-0.194872936620427,
-0.83823817491127));
#32822=CARTESIAN_POINT('Ctrl Pts',(0.00561860216946389,-0.206061640981992,
-0.834532247232247));
#32823=CARTESIAN_POINT('Ctrl Pts',(0.0664740945288613,-0.184086580430367,
-0.830826319553223));
#32824=CARTESIAN_POINT('Ctrl Pts',(0.12732958688826,-0.162111519878741,
-0.827120391874198));
#32825=CARTESIAN_POINT('Ctrl Pts',(0.176209566211245,-0.106972694413925,
-0.823414464195174));
#32826=CARTESIAN_POINT('Ctrl Pts',(0.190729108681027,-0.0439213096311892,
-0.81970853651615));
#32827=CARTESIAN_POINT('Ctrl Pts',(0.205248651150809,0.0191300751515466,
-0.816002608837125));
#32828=CARTESIAN_POINT('Ctrl Pts',(0.185407756767386,0.0900940192522011,
-0.812296681158102));
#32829=CARTESIAN_POINT('Ctrl Pts',(0.140292700021491,0.136472094798379,
-0.808590753479078));
#32830=CARTESIAN_POINT('Ctrl Pts',(0.0951776432755965,0.182850170344557,
-0.804884825800054));
#32831=CARTESIAN_POINT('Ctrl Pts',(0.0247884241672289,0.204642377336258,
-0.801178898121029));
#32832=CARTESIAN_POINT('Ctrl Pts',(-0.0386397287071991,0.191868824209177,
-0.797472970442005));
#32833=CARTESIAN_POINT('Ctrl Pts',(-0.102067881581629,0.179095271082094,
-0.793767042762981));
#32834=CARTESIAN_POINT('Ctrl Pts',(-0.15853496822212,0.131755957836228,
-0.790061115083957));
#32835=CARTESIAN_POINT('Ctrl Pts',(-0.182181496662619,0.0715302496273156,
-0.786355187404933));
#32836=CARTESIAN_POINT('Ctrl Pts',(-0.191046923313482,0.0489507576750034,
-0.784965781340764));
#32837=CARTESIAN_POINT('Ctrl Pts',(-0.195299063071233,0.0245599425690687,
-0.783576375276594));
#32838=CARTESIAN_POINT('Ctrl Pts',(-0.195159317916871,0.00012225950549708,
-0.782186969212424));
#32839=CARTESIAN_POINT('Origin',(0.,0.,-0.78));
#32840=CARTESIAN_POINT('',(-0.195201026479454,-0.00014426443444554,-0.702013030787577));
#32841=CARTESIAN_POINT('',(-0.195224781921234,-0.000153591798034323,-0.712186969212424));
#32842=CARTESIAN_POINT('',(-0.1954,-2.39295984553393E-17,-0.78));
#32843=CARTESIAN_POINT('Ctrl Pts',(-0.195201026479454,-0.00014426443444554,
-0.702013030787577));
#32844=CARTESIAN_POINT('Ctrl Pts',(-0.194908728495298,0.0425702348016472,
-0.704442869957881));
#32845=CARTESIAN_POINT('Ctrl Pts',(-0.181117466392626,0.0854564354592731,
-0.706872709128184));
#32846=CARTESIAN_POINT('Ctrl Pts',(-0.155298824010949,0.119117388361245,
-0.709302548298488));
#32847=CARTESIAN_POINT('Ctrl Pts',(-0.11592090031688,0.170456200652327,
-0.713008475977512));
#32848=CARTESIAN_POINT('Ctrl Pts',(-0.0485654147671141,0.200335648249632,
-0.716714403656536));
#32849=CARTESIAN_POINT('Ctrl Pts',(0.0159217232587258,0.195072231949245,
-0.720420331335561));
#32850=CARTESIAN_POINT('Ctrl Pts',(0.0804088612845667,0.189808815648857,
-0.724126259014585));
#32851=CARTESIAN_POINT('Ctrl Pts',(0.142027651786483,0.149402535450774,
-0.727832186693609));
#32852=CARTESIAN_POINT('Ctrl Pts',(0.172559344466851,0.0923577261865951,
-0.731538114372633));
#32853=CARTESIAN_POINT('Ctrl Pts',(0.203091037147218,0.0353129169224173,
-0.735244042051657));
#32854=CARTESIAN_POINT('Ctrl Pts',(0.202535632006039,-0.0383704214078547,
-0.738949969730681));
#32855=CARTESIAN_POINT('Ctrl Pts',(0.171147480660172,-0.0949484955797788,
-0.742655897409705));
#32856=CARTESIAN_POINT('Ctrl Pts',(0.139759329314305,-0.151526569751704,
-0.746361825088729));
#32857=CARTESIAN_POINT('Ctrl Pts',(0.0775384317637469,-0.190999379765278,
-0.750067752767754));
#32858=CARTESIAN_POINT('Ctrl Pts',(0.0129792773837577,-0.195290079901112,
-0.753773680446778));
#32859=CARTESIAN_POINT('Ctrl Pts',(-0.0515798769962315,-0.199580780036946,
-0.757479608125802));
#32860=CARTESIAN_POINT('Ctrl Pts',(-0.118477288205653,-0.16868937029504,
-0.761185535804826));
#32861=CARTESIAN_POINT('Ctrl Pts',(-0.157076825169889,-0.116762784926257,
-0.76489146348385));
#32862=CARTESIAN_POINT('Ctrl Pts',(-0.181802006392339,-0.0835008772848329,
-0.767265319251759));
#32863=CARTESIAN_POINT('Ctrl Pts',(-0.194916215308456,-0.041607973564115,
-0.769639175019668));
#32864=CARTESIAN_POINT('Ctrl Pts',(-0.195179502128291,0.000133953588564106,
-0.772013030787577));
#32865=CARTESIAN_POINT('Ctrl Pts',(-0.195159317916871,0.00012225950549708,
-0.782186969212424));
#32866=CARTESIAN_POINT('Ctrl Pts',(-0.194926324352933,-0.0406220718268677,
-0.77987044759757));
#32867=CARTESIAN_POINT('Ctrl Pts',(-0.182484747099273,-0.0814966869427612,
-0.777553925982715));
#32868=CARTESIAN_POINT('Ctrl Pts',(-0.158860717615929,-0.114323867746546,
-0.77523740436786));
#32869=CARTESIAN_POINT('Ctrl Pts',(-0.121067439888232,-0.166840173739539,
-0.771531476688836));
#32870=CARTESIAN_POINT('Ctrl Pts',(-0.0546549141923333,-0.198760682553565,
-0.767825549009812));
#32871=CARTESIAN_POINT('Ctrl Pts',(0.00996278506392166,-0.195467176916607,
-0.764119621330788));
#32872=CARTESIAN_POINT('Ctrl Pts',(0.0745804843201748,-0.192173671279648,
-0.760413693651764));
#32873=CARTESIAN_POINT('Ctrl Pts',(0.137403357136784,-0.153666151191704,
-0.75670776597274));
#32874=CARTESIAN_POINT('Ctrl Pts',(0.169661235411597,-0.0975794011899468,
-0.753001838293716));
#32875=CARTESIAN_POINT('Ctrl Pts',(0.201919113686411,-0.0414926511881883,
-0.749295910614691));
#32876=CARTESIAN_POINT('Ctrl Pts',(0.20361199741943,0.0321733287273828,
-0.745589982935668));
#32877=CARTESIAN_POINT('Ctrl Pts',(0.173964618823738,0.0896826947381129,
-0.741884055256643));
#32878=CARTESIAN_POINT('Ctrl Pts',(0.144317240228045,0.147192060748842,
-0.738178127577619));
#32879=CARTESIAN_POINT('Ctrl Pts',(0.0833295993036407,0.188544812854729,
-0.734472199898595));
#32880=CARTESIAN_POINT('Ctrl Pts',(0.0189314070440128,0.194803172883071,
-0.73076627221957));
#32881=CARTESIAN_POINT('Ctrl Pts',(-0.0454667852156141,0.201061532911413,
-0.727060344540546));
#32882=CARTESIAN_POINT('Ctrl Pts',(-0.113275528810465,0.172225500862211,
-0.723354416861523));
#32883=CARTESIAN_POINT('Ctrl Pts',(-0.153441341711563,0.121500736589262,
-0.719648489182499));
#32884=CARTESIAN_POINT('Ctrl Pts',(-0.180397976328058,0.087457632821372,
-0.717161315859141));
#32885=CARTESIAN_POINT('Ctrl Pts',(-0.194903666161545,0.043555393663416,
-0.714674142535782));
#32886=CARTESIAN_POINT('Ctrl Pts',(-0.195224781921234,-0.000153591798034323,
-0.712186969212424));
#32887=CARTESIAN_POINT('Origin',(0.,0.,-0.78));
#32888=CARTESIAN_POINT('',(-0.195700638108693,-5.70533469873291E-5,-0.632013030787577));
#32889=CARTESIAN_POINT('',(-0.195711310405279,-3.91468106102235E-5,-0.642186969212423));
#32890=CARTESIAN_POINT('',(-0.1954,-2.39295984553393E-17,-0.78));
#32891=CARTESIAN_POINT('Ctrl Pts',(-0.195700638108693,-5.70533469873291E-5,
-0.632013030787577));
#32892=CARTESIAN_POINT('Ctrl Pts',(-0.195463028848959,0.0615483382290371,
-0.635540637217069));
#32893=CARTESIAN_POINT('Ctrl Pts',(-0.163955310161744,0.123363079763,-0.639068243646561));
#32894=CARTESIAN_POINT('Ctrl Pts',(-0.113861614071831,0.159192367248385,
-0.642595850076054));
#32895=CARTESIAN_POINT('Ctrl Pts',(-0.0612356710720203,0.196832832778126,
-0.646301777755078));
#32896=CARTESIAN_POINT('Ctrl Pts',(0.0119027926823546,0.205794302636062,
-0.650007705434102));
#32897=CARTESIAN_POINT('Ctrl Pts',(0.0720595130386693,0.181972809864049,
-0.653713633113126));
#32898=CARTESIAN_POINT('Ctrl Pts',(0.132216233394983,0.158151317092035,
-0.65741956079215));
#32899=CARTESIAN_POINT('Ctrl Pts',(0.179391210353237,0.101546861690073,
-0.661125488471174));
#32900=CARTESIAN_POINT('Ctrl Pts',(0.191980337694572,0.0380818445964134,
-0.664831416150198));
#32901=CARTESIAN_POINT('Ctrl Pts',(0.204569465035907,-0.0253831724972469,
-0.668537343829222));
#32902=CARTESIAN_POINT('Ctrl Pts',(0.182572742760322,-0.0957087512826043,
-0.672243271508247));
#32903=CARTESIAN_POINT('Ctrl Pts',(0.136063721617594,-0.140688807688307,
-0.675949199187271));
#32904=CARTESIAN_POINT('Ctrl Pts',(0.0895547004748648,-0.185668864094009,
-0.679655126866295));
#32905=CARTESIAN_POINT('Ctrl Pts',(0.0185333804649922,-0.205303398120056,
-0.683361054545319));
#32906=CARTESIAN_POINT('Ctrl Pts',(-0.0444755348460918,-0.190600639425322,
-0.687066982224343));
#32907=CARTESIAN_POINT('Ctrl Pts',(-0.107484450157176,-0.175897880730587,
-0.690772909903367));
#32908=CARTESIAN_POINT('Ctrl Pts',(-0.162480960769471,-0.126857829315072,
-0.694478837582392));
#32909=CARTESIAN_POINT('Ctrl Pts',(-0.184279035156432,-0.0659387151148841,
-0.698184765261416));
#32910=CARTESIAN_POINT('Ctrl Pts',(-0.191784921575877,-0.044962002041856,
-0.699460853770136));
#32911=CARTESIAN_POINT('Ctrl Pts',(-0.195354533799305,-0.0225768115334816,
-0.700736942278857));
#32912=CARTESIAN_POINT('Ctrl Pts',(-0.195201026479454,-0.00014426443444554,
-0.702013030787577));
#32913=CARTESIAN_POINT('Ctrl Pts',(-0.195224781921234,-0.000153591798034323,
-0.712186969212424));
#32914=CARTESIAN_POINT('Ctrl Pts',(-0.195382133733879,-0.0215716875586284,
-0.710968214856758));
#32915=CARTESIAN_POINT('Ctrl Pts',(-0.192133548947981,-0.0429433801044127,
-0.709749460501092));
#32916=CARTESIAN_POINT('Ctrl Pts',(-0.185275048015275,-0.0630859011262851,
-0.708530706145426));
#32917=CARTESIAN_POINT('Ctrl Pts',(-0.164420059210545,-0.124334278072184,
-0.704824778466402));
#32918=CARTESIAN_POINT('Ctrl Pts',(-0.11018719939374,-0.174217535467284,
-0.701118850787378));
#32919=CARTESIAN_POINT('Ctrl Pts',(-0.0474127809402028,-0.189891291378763,
-0.697412923108353));
#32920=CARTESIAN_POINT('Ctrl Pts',(0.0153616375133333,-0.205565047290241,
-0.693706995429329));
#32921=CARTESIAN_POINT('Ctrl Pts',(0.0866776146036013,-0.187029301718099,
-0.690001067750306));
#32922=CARTESIAN_POINT('Ctrl Pts',(0.133875506521484,-0.142772627249042,
-0.686295140071282));
#32923=CARTESIAN_POINT('Ctrl Pts',(0.181073398439368,-0.0985159527799843,
-0.682589212392258));
#32924=CARTESIAN_POINT('Ctrl Pts',(0.204153205184866,-0.0285383494140109,
-0.678883284713233));
#32925=CARTESIAN_POINT('Ctrl Pts',(0.192545370001613,0.0351134565219624,
-0.675177357034209));
#32926=CARTESIAN_POINT('Ctrl Pts',(0.18093753481836,0.0987652624579367,
-0.671471429355185));
#32927=CARTESIAN_POINT('Ctrl Pts',(0.134642057706355,0.156091270963911,
-0.66776550167616));
#32928=CARTESIAN_POINT('Ctrl Pts',(0.0748602718610678,0.180838640878726,
-0.664059573997136));
#32929=CARTESIAN_POINT('Ctrl Pts',(0.0150784860157823,0.205586010793541,
-0.660353646318112));
#32930=CARTESIAN_POINT('Ctrl Pts',(-0.0581896085627842,0.197754742117199,
-0.656647718639089));
#32931=CARTESIAN_POINT('Ctrl Pts',(-0.11139038239158,0.160931218378025,
-0.652941790960065));
#32932=CARTESIAN_POINT('Ctrl Pts',(-0.162854315214999,0.125309868994405,
-0.649356850377518));
#32933=CARTESIAN_POINT('Ctrl Pts',(-0.195539811246121,0.0625583792222248,
-0.64577190979497));
#32934=CARTESIAN_POINT('Ctrl Pts',(-0.195711310405279,-3.91468106102235E-5,
-0.642186969212423));
#32935=CARTESIAN_POINT('Origin',(0.,0.,-0.78));
#32936=CARTESIAN_POINT('',(-0.195370054518654,0.000178868712723643,-0.562013030787577));
#32937=CARTESIAN_POINT('',(-0.195340204128639,0.000177311515467854,-0.572186969212424));
#32938=CARTESIAN_POINT('',(-0.1954,-2.39295984553393E-17,-0.78));
#32939=CARTESIAN_POINT('Ctrl Pts',(-0.195370054518654,0.000178868712723643,
-0.562013030787577));
#32940=CARTESIAN_POINT('Ctrl Pts',(-0.195516344455089,0.0163065574472149,
-0.562932476797233));
#32941=CARTESIAN_POINT('Ctrl Pts',(-0.193686613410829,0.0324015011250242,
-0.56385192280689));
#32942=CARTESIAN_POINT('Ctrl Pts',(-0.189752676663686,0.047964556165507,
-0.564771368816547));
#32943=CARTESIAN_POINT('Ctrl Pts',(-0.173896514446821,0.110693151253132,
-0.568477296495571));
#32944=CARTESIAN_POINT('Ctrl Pts',(-0.123855822614536,0.164780783696336,
-0.572183224174595));
#32945=CARTESIAN_POINT('Ctrl Pts',(-0.0625470812865084,0.185457648997625,
-0.575889151853619));
#32946=CARTESIAN_POINT('Ctrl Pts',(-0.00123833995847777,0.206134514298915,
-0.579595079532643));
#32947=CARTESIAN_POINT('Ctrl Pts',(0.0713384508652961,0.193400612458291,
-0.583301007211667));
#32948=CARTESIAN_POINT('Ctrl Pts',(0.121946249026466,0.153087521691229,
-0.587006934890692));
#32949=CARTESIAN_POINT('Ctrl Pts',(0.172554047187635,0.112774430924167,
-0.590712862569716));
#32950=CARTESIAN_POINT('Ctrl Pts',(0.201192852686197,0.0448821512306687,
-0.59441879024874));
#32951=CARTESIAN_POINT('Ctrl Pts',(0.194747326928141,-0.0194975794274909,
-0.598124717927764));
#32952=CARTESIAN_POINT('Ctrl Pts',(0.188301801170084,-0.0838773100856497,
-0.601830645606789));
#32953=CARTESIAN_POINT('Ctrl Pts',(0.146771944155409,-0.144744491708471,
-0.605536573285813));
#32954=CARTESIAN_POINT('Ctrl Pts',(0.0891766404718725,-0.174224578470828,
-0.609242500964837));
#32955=CARTESIAN_POINT('Ctrl Pts',(0.0315813367883353,-0.203704665233185,
-0.61294842864386));
#32956=CARTESIAN_POINT('Ctrl Pts',(-0.0420794135640636,-0.201797657135079,
-0.616654356322884));
#32957=CARTESIAN_POINT('Ctrl Pts',(-0.0980721616812089,-0.169376881693938,
-0.620360284001909));
#32958=CARTESIAN_POINT('Ctrl Pts',(-0.154064909798354,-0.136956106252797,
-0.624066211680933));
#32959=CARTESIAN_POINT('Ctrl Pts',(-0.192389655680245,-0.0740215634686213,
-0.627772139359957));
#32960=CARTESIAN_POINT('Ctrl Pts',(-0.195495317498567,-0.00939456147576089,
-0.631478067038982));
#32961=CARTESIAN_POINT('Ctrl Pts',(-0.19564475524912,-0.00628484948270523,
-0.631656388288513));
#32962=CARTESIAN_POINT('Ctrl Pts',(-0.195712649306921,-0.00317121889331525,
-0.631834709538045));
#32963=CARTESIAN_POINT('Ctrl Pts',(-0.195700638108693,-5.70533469873291E-5,
-0.632013030787577));
#32964=CARTESIAN_POINT('Ctrl Pts',(-0.195711310405279,-3.91468106102235E-5,
-0.642186969212423));
#32965=CARTESIAN_POINT('Ctrl Pts',(-0.195717098279537,-0.00215173215114592,
-0.642065982115946));
#32966=CARTESIAN_POINT('Ctrl Pts',(-0.195685853524789,-0.00426414213083437,
-0.641944995019469));
#32967=CARTESIAN_POINT('Ctrl Pts',(-0.195617048160817,-0.00637532797793774,
-0.641824007922991));
#32968=CARTESIAN_POINT('Ctrl Pts',(-0.193509487022232,-0.0710425717927132,
-0.638118080243967));
#32969=CARTESIAN_POINT('Ctrl Pts',(-0.156160911666037,-0.134561280620253,
-0.634412152564944));
#32970=CARTESIAN_POINT('Ctrl Pts',(-0.100675359892449,-0.167842623455736,
-0.63070622488592));
#32971=CARTESIAN_POINT('Ctrl Pts',(-0.0451898081188624,-0.201123966291216,
-0.627000297206896));
#32972=CARTESIAN_POINT('Ctrl Pts',(0.0284327200721153,-0.204167943134643,
-0.623294369527871));
#32973=CARTESIAN_POINT('Ctrl Pts',(0.0864762798789366,-0.175580543786257,
-0.619588441848847));
#32974=CARTESIAN_POINT('Ctrl Pts',(0.14451983968576,-0.14699314443787,-0.615882514169823));
#32975=CARTESIAN_POINT('Ctrl Pts',(0.186984431108425,-0.0867743688976694,
-0.612176586490799));
#32976=CARTESIAN_POINT('Ctrl Pts',(0.194423101487104,-0.0225018209510558,
-0.608470658811775));
#32977=CARTESIAN_POINT('Ctrl Pts',(0.201861771865782,0.0417707269955578,
-0.604764731132751));
#32978=CARTESIAN_POINT('Ctrl Pts',(0.174274521200472,0.110097047348584,
-0.601058803453726));
#32979=CARTESIAN_POINT('Ctrl Pts',(0.12429512129327,0.151186630231212,-0.597352875774702));
#32980=CARTESIAN_POINT('Ctrl Pts',(0.0743157213860675,0.19227621311384,
-0.593646948095678));
#32981=CARTESIAN_POINT('Ctrl Pts',(0.00194417223697229,0.206129058526068,
-0.589941020416654));
#32982=CARTESIAN_POINT('Ctrl Pts',(-0.0596764758368093,0.186401160322774,
-0.58623509273763));
#32983=CARTESIAN_POINT('Ctrl Pts',(-0.121297123910592,0.16667326211948,
-0.582529165058606));
#32984=CARTESIAN_POINT('Ctrl Pts',(-0.17216687090906,0.113364620300662,
-0.578823237379581));
#32985=CARTESIAN_POINT('Ctrl Pts',(-0.188989565178469,0.0508882952321173,
-0.575117309700557));
#32986=CARTESIAN_POINT('Ctrl Pts',(-0.193423562673541,0.0344212618057884,
-0.574140529537846));
#32987=CARTESIAN_POINT('Ctrl Pts',(-0.195492297890079,0.0173173457821699,
-0.573163749375135));
#32988=CARTESIAN_POINT('Ctrl Pts',(-0.195340204128639,0.000177311515467854,
-0.572186969212424));
#32989=CARTESIAN_POINT('Origin',(0.,0.,-0.78));
#32990=CARTESIAN_POINT('',(-0.195089308542836,-4.70021948510008E-5,-0.492013030787576));
#32991=CARTESIAN_POINT('',(-0.195097772416105,-6.2815082009945E-5,-0.502186969212424));
#32992=CARTESIAN_POINT('',(-0.1954,-2.39295984553393E-17,-0.78));
#32993=CARTESIAN_POINT('Ctrl Pts',(-0.195089308542836,-4.70021948510008E-5,
-0.492013030787576));
#32994=CARTESIAN_POINT('Ctrl Pts',(-0.195012935367883,0.0354647848324114,
-0.494030244056422));
#32995=CARTESIAN_POINT('Ctrl Pts',(-0.185752717710553,0.0710136700588578,
-0.496047457325267));
#32996=CARTESIAN_POINT('Ctrl Pts',(-0.167549278060548,0.101162821088464,
-0.498064670594113));
#32997=CARTESIAN_POINT('Ctrl Pts',(-0.134106789904096,0.156551398501326,
-0.501770598273137));
#32998=CARTESIAN_POINT('Ctrl Pts',(-0.0704797828327725,0.193715181859728,
-0.505476525952161));
#32999=CARTESIAN_POINT('Ctrl Pts',(-0.00580668377942445,0.195634760133963,
-0.509182453631185));
#33000=CARTESIAN_POINT('Ctrl Pts',(0.0588664152739227,0.197554338408197,
-0.512888381310209));
#33001=CARTESIAN_POINT('Ctrl Pts',(0.124585606309294,0.164229711598261,
-0.516594308989234));
#33002=CARTESIAN_POINT('Ctrl Pts',(0.161254332310831,0.110922122501218,
-0.520300236668258));
#33003=CARTESIAN_POINT('Ctrl Pts',(0.197923058312368,0.0576145334041769,
-0.524006164347282));
#33004=CARTESIAN_POINT('Ctrl Pts',(0.205541319280075,-0.0156760179799715,
-0.527712092026305));
#33005=CARTESIAN_POINT('Ctrl Pts',(0.180620280035612,-0.0753856179190998,
-0.53141801970533));
#33006=CARTESIAN_POINT('Ctrl Pts',(0.155699240791148,-0.135095217858229,
-0.535123947384354));
#33007=CARTESIAN_POINT('Ctrl Pts',(0.0982389013345159,-0.181223866352336,
-0.538829875063378));
#33008=CARTESIAN_POINT('Ctrl Pts',(0.0345536206126452,-0.192646630522687,
-0.542535802742402));
#33009=CARTESIAN_POINT('Ctrl Pts',(-0.0291316601092254,-0.204069394693038,
-0.546241730421427));
#33010=CARTESIAN_POINT('Ctrl Pts',(-0.0990418820963334,-0.180786274539629,
-0.54994765810045));
#33011=CARTESIAN_POINT('Ctrl Pts',(-0.143161176789165,-0.133459935596901,
-0.553653585779475));
#33012=CARTESIAN_POINT('Ctrl Pts',(-0.176334410746974,-0.0978753296995445,
-0.556440067448842));
#33013=CARTESIAN_POINT('Ctrl Pts',(-0.194926706870171,-0.0486978554841558,
-0.559226549118209));
#33014=CARTESIAN_POINT('Ctrl Pts',(-0.195370054518654,0.000178868712723643,
-0.562013030787577));
#33015=CARTESIAN_POINT('Ctrl Pts',(-0.195340204128639,0.000177311515467854,
-0.572186969212424));
#33016=CARTESIAN_POINT('Ctrl Pts',(-0.194915250462372,-0.0477123608327619,
-0.569457821696111));
#33017=CARTESIAN_POINT('Ctrl Pts',(-0.177153235872989,-0.0958839928397431,
-0.566728674179798));
#33018=CARTESIAN_POINT('Ctrl Pts',(-0.145204503609113,-0.131233861749203,
-0.563999526663485));
#33019=CARTESIAN_POINT('Ctrl Pts',(-0.101821106229999,-0.17923568534371,
-0.560293598984461));
#33020=CARTESIAN_POINT('Ctrl Pts',(-0.0322786699314196,-0.203595324214454,
-0.556587671305437));
#33021=CARTESIAN_POINT('Ctrl Pts',(0.031575366720999,-0.193157113652105,
-0.552881743626412));
#33022=CARTESIAN_POINT('Ctrl Pts',(0.0954294033734167,-0.182718903089756,
-0.549175815947388));
#33023=CARTESIAN_POINT('Ctrl Pts',(0.153595040379674,-0.137482843094316,
-0.545469888268365));
#33024=CARTESIAN_POINT('Ctrl Pts',(0.179434922913233,-0.0781650994824409,
-0.541763960589341));
#33025=CARTESIAN_POINT('Ctrl Pts',(0.205274805446792,-0.0188473558705653,
-0.538058032910317));
#33026=CARTESIAN_POINT('Ctrl Pts',(0.198788933507652,0.0545520713577456,
-0.534352105231292));
#33027=CARTESIAN_POINT('Ctrl Pts',(0.162947556904712,0.108419408026255,
-0.530646177552268));
#33028=CARTESIAN_POINT('Ctrl Pts',(0.127106180301771,0.162286744694765,
-0.526940249873244));
#33029=CARTESIAN_POINT('Ctrl Pts',(0.0619092990350311,0.196621990803474,
-0.52323432219422));
#33030=CARTESIAN_POINT('Ctrl Pts',(-0.00278572524228628,0.195701083473885,
-0.519528394515196));
#33031=CARTESIAN_POINT('Ctrl Pts',(-0.0674807495196046,0.194780176144295,
-0.515822466836172));
#33032=CARTESIAN_POINT('Ctrl Pts',(-0.131673916807498,0.158603115376409,
-0.512116539157147));
#33033=CARTESIAN_POINT('Ctrl Pts',(-0.165967523195273,0.103737435780939,
-0.508410611478123));
#33034=CARTESIAN_POINT('Ctrl Pts',(-0.185164798177752,0.0730240857067314,
-0.506336064056223));
#33035=CARTESIAN_POINT('Ctrl Pts',(-0.194992546219555,0.0364543446917346,
-0.504261516634324));
#33036=CARTESIAN_POINT('Ctrl Pts',(-0.195097772416105,-6.2815082009945E-5,
-0.502186969212424));
#33037=CARTESIAN_POINT('Origin',(0.,0.,-0.78));
#33038=CARTESIAN_POINT('',(-0.195542596598123,-0.000155681910894878,-0.422013030787576));
#33039=CARTESIAN_POINT('',(-0.19557059622782,-0.000146131833415082,-0.432186969212424));
#33040=CARTESIAN_POINT('',(-0.1954,-2.39295984553393E-17,-0.78));
#33041=CARTESIAN_POINT('Ctrl Pts',(-0.195542596598123,-0.000155681910894878,
-0.422013030787576));
#33042=CARTESIAN_POINT('Ctrl Pts',(-0.195068207836276,0.0543592358526127,
-0.42512801131561));
#33043=CARTESIAN_POINT('Ctrl Pts',(-0.171264515120332,0.109237316871241,
-0.428242991843644));
#33044=CARTESIAN_POINT('Ctrl Pts',(-0.130811232943367,0.145585364254193,
-0.431357972371678));
#33045=CARTESIAN_POINT('Ctrl Pts',(-0.0826835041252334,0.188829048656927,
-0.435063900050703));
#33046=CARTESIAN_POINT('Ctrl Pts',(-0.0109897284654487,0.205845080920964,
-0.438769827729727));
#33047=CARTESIAN_POINT('Ctrl Pts',(0.0514374347650197,0.188840851655517,
-0.442475755408751));
#33048=CARTESIAN_POINT('Ctrl Pts',(0.113864597995486,0.171836622390071,
-0.446181683087775));
#33049=CARTESIAN_POINT('Ctrl Pts',(0.16702514879664,0.120812131595144,-0.449887610766799));
#33050=CARTESIAN_POINT('Ctrl Pts',(0.186573846106103,0.059134396913838,
-0.453593538445823));
#33051=CARTESIAN_POINT('Ctrl Pts',(0.206122543415566,-0.00254333776746921,
-0.457299466124847));
#33052=CARTESIAN_POINT('Ctrl Pts',(0.192059387233338,-0.074874316335157,
-0.461005393803871));
#33053=CARTESIAN_POINT('Ctrl Pts',(0.150824696972863,-0.124734068049718,
-0.464711321482896));
#33054=CARTESIAN_POINT('Ctrl Pts',(0.10959000671239,-0.174593819764278,
-0.46841724916192));
#33055=CARTESIAN_POINT('Ctrl Pts',(0.0411837823736688,-0.201982344625713,
-0.472123176840944));
#33056=CARTESIAN_POINT('Ctrl Pts',(-0.0230668735848738,-0.194356878685079,
-0.475829104519968));
#33057=CARTESIAN_POINT('Ctrl Pts',(-0.0873175295434183,-0.186731412744445,
-0.479535032198992));
#33058=CARTESIAN_POINT('Ctrl Pts',(-0.147412617121784,-0.144091956001744,
-0.483240959878016));
#33059=CARTESIAN_POINT('Ctrl Pts',(-0.17583117629018,-0.0859655418967326,
-0.48694688755704));
#33060=CARTESIAN_POINT('Ctrl Pts',(-0.188780924515387,-0.059478540095068,
-0.488635601967219));
#33061=CARTESIAN_POINT('Ctrl Pts',(-0.195153244509888,-0.0297757707937514,
-0.490324316377398));
#33062=CARTESIAN_POINT('Ctrl Pts',(-0.195089308542836,-4.70021948510008E-5,
-0.492013030787576));
#33063=CARTESIAN_POINT('Ctrl Pts',(-0.195097772416105,-6.2815082009945E-5,
-0.502186969212424));
#33064=CARTESIAN_POINT('Ctrl Pts',(-0.195180520073629,-0.0287791379157325,
-0.500555588955299));
#33065=CARTESIAN_POINT('Ctrl Pts',(-0.189250940656692,-0.0574629449448703,
-0.498924208698175));
#33066=CARTESIAN_POINT('Ctrl Pts',(-0.177137376206997,-0.0832407609796949,
-0.497292828441051));
#33067=CARTESIAN_POINT('Ctrl Pts',(-0.149619577343291,-0.141798979721807,
-0.493586900762027));
#33068=CARTESIAN_POINT('Ctrl Pts',(-0.0901899341282235,-0.185361118782977,
-0.489880973083003));
#33069=CARTESIAN_POINT('Ctrl Pts',(-0.0260646617536622,-0.193977595988931,
-0.486175045403978));
#33070=CARTESIAN_POINT('Ctrl Pts',(0.0380606106208982,-0.202594073194885,
-0.482469117724954));
#33071=CARTESIAN_POINT('Ctrl Pts',(0.106881512154954,-0.176264888545622,
-0.47876319004593));
#33072=CARTESIAN_POINT('Ctrl Pts',(0.148881036107087,-0.127047673830174,
-0.475057262366906));
#33073=CARTESIAN_POINT('Ctrl Pts',(0.19088056005922,-0.0778304591147251,
-0.471351334687882));
#33074=CARTESIAN_POINT('Ctrl Pts',(0.206058706429431,-0.00572521433309026,
-0.467645407008858));
#33075=CARTESIAN_POINT('Ctrl Pts',(0.187464538353933,0.0562469661201786,
-0.463939479329834));
#33076=CARTESIAN_POINT('Ctrl Pts',(0.168870370278435,0.118219146573448,
-0.46023355165081));
#33077=CARTESIAN_POINT('Ctrl Pts',(0.116503887757229,0.170058262698351,
-0.456527623971785));
#33078=CARTESIAN_POINT('Ctrl Pts',(0.0543466828045978,0.188024233560768,
-0.452821696292761));
#33079=CARTESIAN_POINT('Ctrl Pts',(-0.00781052214803026,0.205990204423184,
-0.449115768613737));
#33080=CARTESIAN_POINT('Ctrl Pts',(-0.0797584495320804,0.190083030023117,
-0.445409840934713));
#33081=CARTESIAN_POINT('Ctrl Pts',(-0.12854804954076,0.147587510641126,
-0.441703913255689));
#33082=CARTESIAN_POINT('Ctrl Pts',(-0.170312481498787,0.111210880633205,
-0.4385315985746));
#33083=CARTESIAN_POINT('Ctrl Pts',(-0.195107539066149,0.0553515145401952,
-0.435359283893512));
#33084=CARTESIAN_POINT('Ctrl Pts',(-0.19557059622782,-0.000146131833415082,
-0.432186969212424));
#33085=CARTESIAN_POINT('Origin',(0.,0.,-0.78));
#33086=CARTESIAN_POINT('',(-0.195583232845723,0.00014114408237359,-0.352013030787576));
#33087=CARTESIAN_POINT('',(-0.195555830895482,0.000151412478162425,-0.362186969212424));
#33088=CARTESIAN_POINT('',(-0.1954,-2.39295984553393E-17,-0.78));
#33089=CARTESIAN_POINT('Ctrl Pts',(-0.195583232845723,0.00014114408237359,
-0.352013030787576));
#33090=CARTESIAN_POINT('Ctrl Pts',(-0.195655424697362,0.00900615037703061,
-0.352519850895775));
#33091=CARTESIAN_POINT('Ctrl Pts',(-0.195104888905283,0.0178621385962115,
-0.353026671003973));
#33092=CARTESIAN_POINT('Ctrl Pts',(-0.193901018627014,0.0266284044659732,
-0.353533491112172));
#33093=CARTESIAN_POINT('Ctrl Pts',(-0.1850981788935,0.0907283618333217,
-0.357239418791196));
#33094=CARTESIAN_POINT('Ctrl Pts',(-0.141363472953698,0.150031130055026,
-0.36094534647022));
#33095=CARTESIAN_POINT('Ctrl Pts',(-0.0827255111732556,0.177378597216332,
-0.364651274149244));
#33096=CARTESIAN_POINT('Ctrl Pts',(-0.0240875493928135,0.204726064377639,
-0.368357201828268));
#33097=CARTESIAN_POINT('Ctrl Pts',(0.0494536682282692,0.200118230478549,
-0.372063129507292));
#33098=CARTESIAN_POINT('Ctrl Pts',(0.104219433624227,0.165665284849347,
-0.375769057186316));
#33099=CARTESIAN_POINT('Ctrl Pts',(0.158985199020186,0.131212339220144,
-0.37947498486534));
#33100=CARTESIAN_POINT('Ctrl Pts',(0.194975512191018,0.0669142818608283,
-0.383180912544365));
#33101=CARTESIAN_POINT('Ctrl Pts',(0.195708360877096,0.00221685181364163,
-0.386886840223389));
#33102=CARTESIAN_POINT('Ctrl Pts',(0.196441209563174,-0.062480578233545,
-0.390592767902413));
#33103=CARTESIAN_POINT('Ctrl Pts',(0.161916593764496,-0.127577380968602,
-0.394298695581437));
#33104=CARTESIAN_POINT('Ctrl Pts',(0.107945299515574,-0.163262026392235,
-0.398004623260461));
#33105=CARTESIAN_POINT('Ctrl Pts',(0.0539740052666519,-0.198946671815868,
-0.401710550939485));
#33106=CARTESIAN_POINT('Ctrl Pts',(-0.0194439674325147,-0.205219159928075,
-0.40541647861851));
#33107=CARTESIAN_POINT('Ctrl Pts',(-0.0786863513792303,-0.17920696151603,
-0.409122406297534));
#33108=CARTESIAN_POINT('Ctrl Pts',(-0.137928735325944,-0.153194763103985,
-0.412828333976558));
#33109=CARTESIAN_POINT('Ctrl Pts',(-0.182995530520208,-0.0948978781676894,
-0.416534261655582));
#33110=CARTESIAN_POINT('Ctrl Pts',(-0.193248087129097,-0.031013767428828,
-0.420240189334606));
#33111=CARTESIAN_POINT('Ctrl Pts',(-0.194882959593738,-0.0208268084527132,
-0.420831136485596));
#33112=CARTESIAN_POINT('Ctrl Pts',(-0.195632593529003,-0.0104977803763184,
-0.421422083636586));
#33113=CARTESIAN_POINT('Ctrl Pts',(-0.195542596598123,-0.000155681910894878,
-0.422013030787576));
#33114=CARTESIAN_POINT('Ctrl Pts',(-0.19557059622782,-0.000146131833415082,
-0.432186969212424));
#33115=CARTESIAN_POINT('Ctrl Pts',(-0.195648486773083,-0.00948135498650791,
-0.431653356214488));
#33116=CARTESIAN_POINT('Ctrl Pts',(-0.195037918301464,-0.0188063435021582,
-0.431119743216553));
#33117=CARTESIAN_POINT('Ctrl Pts',(-0.193703849275159,-0.0280266500667519,
-0.430586130218617));
#33118=CARTESIAN_POINT('Ctrl Pts',(-0.184438776367567,-0.0920614270287232,
-0.426880202539593));
#33119=CARTESIAN_POINT('Ctrl Pts',(-0.140277357919073,-0.151047116588746,
-0.423174274860568));
#33120=CARTESIAN_POINT('Ctrl Pts',(-0.0814436202345694,-0.177970815194695,
-0.419468347181544));
#33121=CARTESIAN_POINT('Ctrl Pts',(-0.0226098825500687,-0.204894513800643,
-0.41576241950252));
#33122=CARTESIAN_POINT('Ctrl Pts',(0.0508961743704401,-0.199756221452522,
-0.412056491823496));
#33123=CARTESIAN_POINT('Ctrl Pts',(0.105411944547391,-0.164909054586819,
-0.408350564144472));
#33124=CARTESIAN_POINT('Ctrl Pts',(0.159927714724343,-0.130061887721115,
-0.404644636465448));
#33125=CARTESIAN_POINT('Ctrl Pts',(0.195453198157735,-0.0655058463378307,
-0.400938708786423));
#33126=CARTESIAN_POINT('Ctrl Pts',(0.195719254573281,-0.000804815043615771,
-0.397232781107399));
#33127=CARTESIAN_POINT('Ctrl Pts',(0.195985310988826,0.0638962162505983,
-0.393526853428375));
#33128=CARTESIAN_POINT('Ctrl Pts',(0.160991940386524,0.128742237455741,
-0.389820925749351));
#33129=CARTESIAN_POINT('Ctrl Pts',(0.106764598297912,0.164036565704904,
-0.386114998070327));
#33130=CARTESIAN_POINT('Ctrl Pts',(0.052537256209301,0.199330893954067,
-0.382409070391303));
#33131=CARTESIAN_POINT('Ctrl Pts',(-0.0209240573656208,0.205073529247252,
-0.378703142712278));
#33132=CARTESIAN_POINT('Ctrl Pts',(-0.0799772269710618,0.178634592125981,
-0.374997215033254));
#33133=CARTESIAN_POINT('Ctrl Pts',(-0.139030396576502,0.152195655004712,
-0.37129128735423));
#33134=CARTESIAN_POINT('Ctrl Pts',(-0.183675422212462,0.0935751454689875,
-0.367585359675206));
#33135=CARTESIAN_POINT('Ctrl Pts',(-0.193466806325688,0.0296187303592283,
-0.363879431996182));
#33136=CARTESIAN_POINT('Ctrl Pts',(-0.194957351082485,0.0198826299159174,
-0.36331527773493));
#33137=CARTESIAN_POINT('Ctrl Pts',(-0.19564019594481,0.0100228749509908,
-0.362751123473677));
#33138=CARTESIAN_POINT('Ctrl Pts',(-0.195555830895482,0.000151412478162425,
-0.362186969212424));
#33139=CARTESIAN_POINT('Origin',(0.,0.,-0.78));
#33140=CARTESIAN_POINT('',(-0.195102573297888,7.00326263145673E-5,-0.282013030787576));
#33141=CARTESIAN_POINT('',(-0.195092954415088,5.44486870368686E-5,-0.292186969212424));
#33142=CARTESIAN_POINT('',(-0.1954,-2.39295984553393E-17,-0.78));
#33143=CARTESIAN_POINT('Ctrl Pts',(-0.195102573297888,7.00326263145673E-5,
-0.282013030787576));
#33144=CARTESIAN_POINT('Ctrl Pts',(-0.195193440705579,0.0283130019996957,
-0.283617618154963));
#33145=CARTESIAN_POINT('Ctrl Pts',(-0.189464713165188,0.0565208456325242,
-0.28522220552235));
#33146=CARTESIAN_POINT('Ctrl Pts',(-0.177733329944698,0.081960602518178,
-0.286826792889737));
#33147=CARTESIAN_POINT('Ctrl Pts',(-0.150638726887431,0.140715832121982,
-0.290532720568761));
#33148=CARTESIAN_POINT('Ctrl Pts',(-0.0915249166295698,0.184705606595511,
-0.294238648247786));
#33149=CARTESIAN_POINT('Ctrl Pts',(-0.0274634764115514,0.193784505101985,
-0.29794457592681));
#33150=CARTESIAN_POINT('Ctrl Pts',(0.0365979638064669,0.202863403608459,
-0.301650503605834));
#33151=CARTESIAN_POINT('Ctrl Pts',(0.105607033984642,0.177031426147878,
-0.305356431284858));
#33152=CARTESIAN_POINT('Ctrl Pts',(0.147960554216137,0.128118505085543,
-0.309062358963882));
#33153=CARTESIAN_POINT('Ctrl Pts',(0.190314074447633,0.0792055840232077,
-0.312768286642906));
#33154=CARTESIAN_POINT('Ctrl Pts',(0.206012044732447,0.00721171935911754,
-0.31647421432193));
#33155=CARTESIAN_POINT('Ctrl Pts',(0.187865471277307,-0.0548930018261547,
-0.320180142000955));
#33156=CARTESIAN_POINT('Ctrl Pts',(0.169718897822168,-0.116997723011427,
-0.323886069679979));
#33157=CARTESIAN_POINT('Ctrl Pts',(0.117727780627074,-0.169213300717881,
-0.327591997359002));
#33158=CARTESIAN_POINT('Ctrl Pts',(0.0557018105550347,-0.187627250821613,
-0.331297925038027));
#33159=CARTESIAN_POINT('Ctrl Pts',(-0.00632415951700459,-0.206041200925345,
-0.335003852717051));
#33160=CARTESIAN_POINT('Ctrl Pts',(-0.0783849824659894,-0.190653523426354,
-0.338709780396075));
#33161=CARTESIAN_POINT('Ctrl Pts',(-0.12747990717687,-0.148511111420363,
-0.342415708075099));
#33162=CARTESIAN_POINT('Ctrl Pts',(-0.169860643914036,-0.112132066555481,
-0.345614815645925));
#33163=CARTESIAN_POINT('Ctrl Pts',(-0.19512754946735,-0.0558158084810627,
-0.348813923216751));
#33164=CARTESIAN_POINT('Ctrl Pts',(-0.195583232845723,0.00014114408237359,
-0.352013030787576));
#33165=CARTESIAN_POINT('Ctrl Pts',(-0.195555830895482,0.000151412478162425,
-0.362186969212424));
#33166=CARTESIAN_POINT('Ctrl Pts',(-0.195086002184484,-0.0548227329316184,
-0.359045195794653));
#33167=CARTESIAN_POINT('Ctrl Pts',(-0.1708221338281,-0.110159971808954,
-0.355903422376881));
#33168=CARTESIAN_POINT('Ctrl Pts',(-0.129757467814254,-0.146525335298689,
-0.35276164895911));
#33169=CARTESIAN_POINT('Ctrl Pts',(-0.0813190025991063,-0.189420665163049,
-0.349055721280085));
#33170=CARTESIAN_POINT('Ctrl Pts',(-0.00950432957832131,-0.205919004207974,
-0.345349793601062));
#33171=CARTESIAN_POINT('Ctrl Pts',(0.052798526195835,-0.188464824223644,
-0.341643865922038));
#33172=CARTESIAN_POINT('Ctrl Pts',(0.115101381969993,-0.171010644239313,
-0.337937938243013));
#33173=CARTESIAN_POINT('Ctrl Pts',(0.167892420497522,-0.119603945225725,
-0.334232010563989));
#33174=CARTESIAN_POINT('Ctrl Pts',(0.186995621412669,-0.0577867797188634,
-0.330526082884965));
#33175=CARTESIAN_POINT('Ctrl Pts',(0.206098822327817,0.00403038578799705,
-0.326820155205941));
#33176=CARTESIAN_POINT('Ctrl Pts',(0.191514185630584,0.0762580177881299,
-0.323114227526917));
#33177=CARTESIAN_POINT('Ctrl Pts',(0.14992084633237,0.125818973819177,-0.319408299847893));
#33178=CARTESIAN_POINT('Ctrl Pts',(0.108327507034157,0.175379929850223,
-0.315702372168869));
#33179=CARTESIAN_POINT('Ctrl Pts',(0.0397254651349634,0.202274209912184,
-0.311996444489844));
#33180=CARTESIAN_POINT('Ctrl Pts',(-0.0244685008994722,0.194185392865971,
-0.30829051681082));
#33181=CARTESIAN_POINT('Ctrl Pts',(-0.0886624669339077,0.186096575819758,
-0.304584589131796));
#33182=CARTESIAN_POINT('Ctrl Pts',(-0.148448357103585,0.143024661665371,
-0.300878661452772));
#33183=CARTESIAN_POINT('Ctrl Pts',(-0.176446810473754,0.0846947307106876,
-0.297172733773748));
#33184=CARTESIAN_POINT('Ctrl Pts',(-0.189002703687302,0.0585367006746086,
-0.295510812253306));
#33185=CARTESIAN_POINT('Ctrl Pts',(-0.195165921495514,0.0293101769644822,
-0.293848890732865));
#33186=CARTESIAN_POINT('Ctrl Pts',(-0.195092954415088,5.44486870368687E-5,
-0.292186969212424));
#33187=CARTESIAN_POINT('Origin',(0.,0.,-0.78));
#33188=CARTESIAN_POINT('',(-0.195326501059731,-0.000176025207787534,-0.212013030787576));
#33189=CARTESIAN_POINT('',(-0.195356026374599,-0.000178344182095036,-0.222186969212423));
#33190=CARTESIAN_POINT('',(-0.1954,-2.39295984553393E-17,-0.78));
#33191=CARTESIAN_POINT('Ctrl Pts',(-0.195326501059731,-0.000176025207787534,
-0.212013030787576));
#33192=CARTESIAN_POINT('Ctrl Pts',(-0.194911123079697,0.04725196296477,
-0.214715385414152));
#33193=CARTESIAN_POINT('Ctrl Pts',(-0.177529267435098,0.0949526855082682,
-0.217417740040727));
#33194=CARTESIAN_POINT('Ctrl Pts',(-0.146147542718918,0.130182841238995,
-0.220120094667303));
#33195=CARTESIAN_POINT('Ctrl Pts',(-0.10311159136838,0.178496414881354,
-0.223826022346327));
#33196=CARTESIAN_POINT('Ctrl Pts',(-0.033746712246184,0.203357151128855,
-0.227531950025351));
#33197=CARTESIAN_POINT('Ctrl Pts',(0.0301809729126184,0.193379900723762,
-0.231237877704375));
#33198=CARTESIAN_POINT('Ctrl Pts',(0.0941086580714263,0.183402650318669,
-0.2349438053834));
#33199=CARTESIAN_POINT('Ctrl Pts',(0.152599149266839,0.138587413260975,
-0.238649733062424));
#33200=CARTESIAN_POINT('Ctrl Pts',(0.178866320722857,0.0794576384627894,
-0.242355660741448));
#33201=CARTESIAN_POINT('Ctrl Pts',(0.205133492178873,0.0203278636646087,
-0.246061588420472));
#33202=CARTESIAN_POINT('Ctrl Pts',(0.199177343895502,-0.0531164488740613,
-0.249767516099496));
#33203=CARTESIAN_POINT('Ctrl Pts',(0.163725535988198,-0.10724097041851,
-0.25347344377852));
#33204=CARTESIAN_POINT('Ctrl Pts',(0.128273728080893,-0.161365491962961,
-0.257179371457544));
#33205=CARTESIAN_POINT('Ctrl Pts',(0.0633262605496548,-0.196170222513189,
-0.260885299136568));
#33206=CARTESIAN_POINT('Ctrl Pts',(-0.00137372617158459,-0.195716095036698,
-0.264591226815592));
#33207=CARTESIAN_POINT('Ctrl Pts',(-0.066073712892824,-0.195261967560207,
-0.268297154494617));
#33208=CARTESIAN_POINT('Ctrl Pts',(-0.130526218804065,-0.159548982056996,
-0.272003082173641));
#33209=CARTESIAN_POINT('Ctrl Pts',(-0.16521477383135,-0.104932146938352,
-0.275709009852665));
#33210=CARTESIAN_POINT('Ctrl Pts',(-0.184883926967784,-0.073963232466964,
-0.277810350164302));
#33211=CARTESIAN_POINT('Ctrl Pts',(-0.194983574887034,-0.0369164794644935,
-0.279911690475939));
#33212=CARTESIAN_POINT('Ctrl Pts',(-0.195102573297888,7.00326263145673E-5,
-0.282013030787576));
#33213=CARTESIAN_POINT('Ctrl Pts',(-0.195092954415088,5.44486870368687E-5,
-0.292186969212424));
#33214=CARTESIAN_POINT('Ctrl Pts',(-0.195003211812967,-0.0359273278513876,
-0.290142963053841));
#33215=CARTESIAN_POINT('Ctrl Pts',(-0.185480197162667,-0.0719532811795465,
-0.288098956895258));
#33216=CARTESIAN_POINT('Ctrl Pts',(-0.16681505127669,-0.102369004125496,
-0.286054950736675));
#33217=CARTESIAN_POINT('Ctrl Pts',(-0.132973822138797,-0.157514860252015,
-0.282349023057651));
#33218=CARTESIAN_POINT('Ctrl Pts',(-0.0690803472923488,-0.194218624750074,
-0.278643095378627));
#33219=CARTESIAN_POINT('Ctrl Pts',(-0.00439508445617105,-0.195671555356572,
-0.274937167699603));
#33220=CARTESIAN_POINT('Ctrl Pts',(0.0602901783800058,-0.19712448596307,
-0.271231240020579));
#33221=CARTESIAN_POINT('Ctrl Pts',(0.125767229205913,-0.163326582678009,
-0.267525312341555));
#33222=CARTESIAN_POINT('Ctrl Pts',(0.162050400841887,-0.109755828611132,
-0.263819384662531));
#33223=CARTESIAN_POINT('Ctrl Pts',(0.198333572477861,-0.0561850745442543,
-0.260113456983507));
#33224=CARTESIAN_POINT('Ctrl Pts',(0.205422864923902,0.0171585303044398,
-0.256407529304482));
#33225=CARTESIAN_POINT('Ctrl Pts',(0.18007168767881,0.0766867761647091,
-0.252701601625458));
#33226=CARTESIAN_POINT('Ctrl Pts',(0.154720510433717,0.136215022024978,
-0.248995673946434));
#33227=CARTESIAN_POINT('Ctrl Pts',(0.0969288634974908,0.181927908896823,
-0.24528974626741));
#33228=CARTESIAN_POINT('Ctrl Pts',(0.0331628305678363,0.19289090449688,
-0.241583818588386));
#33229=CARTESIAN_POINT('Ctrl Pts',(-0.0306032023618182,0.203853900096938,
-0.237877890909362));
#33230=CARTESIAN_POINT('Ctrl Pts',(-0.100343621284901,0.180067004425208,
-0.234171963230337));
#33231=CARTESIAN_POINT('Ctrl Pts',(-0.144120320515705,0.132423591077881,
-0.230466035551313));
#33232=CARTESIAN_POINT('Ctrl Pts',(-0.176719463332301,0.0969450268354948,
-0.227706346771683));
#33233=CARTESIAN_POINT('Ctrl Pts',(-0.194920901915774,0.0482372685640377,
-0.224946657992053));
#33234=CARTESIAN_POINT('Ctrl Pts',(-0.195356026374599,-0.000178344182095036,
-0.222186969212423));
#33235=CARTESIAN_POINT('Origin',(0.,0.,-0.78));
#33236=CARTESIAN_POINT('',(-0.195715103822041,3.06823192254271E-5,-0.142013030787576));
#33237=CARTESIAN_POINT('',(-0.195706082681088,4.87745040611329E-5,-0.152186969212423));
#33238=CARTESIAN_POINT('',(-0.1954,-2.39295984553393E-17,-0.78));
#33239=CARTESIAN_POINT('Ctrl Pts',(-0.195715103822041,3.06823192254271E-5,
-0.142013030787576));
#33240=CARTESIAN_POINT('Ctrl Pts',(-0.195718688241172,0.00167534937911104,
-0.142107224994316));
#33241=CARTESIAN_POINT('Ctrl Pts',(-0.195699753624677,0.00331993167571746,
-0.142201419201056));
#33242=CARTESIAN_POINT('Ctrl Pts',(-0.19565804723958,0.00496393608527703,
-0.142295613407796));
#33243=CARTESIAN_POINT('Ctrl Pts',(-0.194017173004602,0.0696447870281606,
-0.14600154108682));
#33244=CARTESIAN_POINT('Ctrl Pts',(-0.157127667667993,0.133431121269766,
-0.149707468765844));
#33245=CARTESIAN_POINT('Ctrl Pts',(-0.101883633031363,0.167111867856658,
-0.153413396444869));
#33246=CARTESIAN_POINT('Ctrl Pts',(-0.0466395983947323,0.200792614443549,
-0.157119324123893));
#33247=CARTESIAN_POINT('Ctrl Pts',(0.0269589655419205,0.204367773375727,
-0.160825251802917));
#33248=CARTESIAN_POINT('Ctrl Pts',(0.0852072452906279,0.176199907320885,
-0.164531179481941));
#33249=CARTESIAN_POINT('Ctrl Pts',(0.143455525039335,0.148032041266044,
-0.168237107160965));
#33250=CARTESIAN_POINT('Ctrl Pts',(0.186353520600098,0.0881211502241835,
-0.171943034839989));
#33251=CARTESIAN_POINT('Ctrl Pts',(0.194255716558216,0.023903928747813,
-0.175648962519013));
#33252=CARTESIAN_POINT('Ctrl Pts',(0.202157912516335,-0.0403132927285585,
-0.179354890198038));
#33253=CARTESIAN_POINT('Ctrl Pts',(0.17506430887181,-0.108836844639439,
-0.183060817877062));
#33254=CARTESIAN_POINT('Ctrl Pts',(0.125382651628076,-0.150285940104107,
-0.186766745556086));
#33255=CARTESIAN_POINT('Ctrl Pts',(0.0757009943843419,-0.191735035568774,
-0.19047267323511));
#33256=CARTESIAN_POINT('Ctrl Pts',(0.00343128354139923,-0.206109674587227,
-0.194178600914134));
#33257=CARTESIAN_POINT('Ctrl Pts',(-0.0583300908676832,-0.186826867575142,
-0.197884528593158));
#33258=CARTESIAN_POINT('Ctrl Pts',(-0.120091465276766,-0.167544060563056,
-0.201590456272182));
#33259=CARTESIAN_POINT('Ctrl Pts',(-0.171344503251989,-0.11460380752043,
-0.205296383951207));
#33260=CARTESIAN_POINT('Ctrl Pts',(-0.188617510450161,-0.0522504754805079,
-0.209002311630231));
#33261=CARTESIAN_POINT('Ctrl Pts',(-0.193295077326858,-0.0353650613047726,
-0.210005884682679));
#33262=CARTESIAN_POINT('Ctrl Pts',(-0.195480759920963,-0.0177893504145328,
-0.211009457735128));
#33263=CARTESIAN_POINT('Ctrl Pts',(-0.195326501059731,-0.000176025207787534,
-0.212013030787576));
#33264=CARTESIAN_POINT('Ctrl Pts',(-0.195356026374599,-0.000178344182095036,
-0.222186969212423));
#33265=CARTESIAN_POINT('Ctrl Pts',(-0.195505221346168,-0.0167790335266869,
-0.221240730313029));
#33266=CARTESIAN_POINT('Ctrl Pts',(-0.193565703574764,-0.0333453765191166,
-0.220294491413635));
#33267=CARTESIAN_POINT('Ctrl Pts',(-0.189401681496759,-0.0493323163259868,
-0.219348252514241));
#33268=CARTESIAN_POINT('Ctrl Pts',(-0.173093363708484,-0.111944879359601,
-0.215642324835217));
#33269=CARTESIAN_POINT('Ctrl Pts',(-0.122663748593409,-0.165670074403903,
-0.211936397156193));
#33270=CARTESIAN_POINT('Ctrl Pts',(-0.0612074277809205,-0.185904075543387,
-0.208230469477169));
#33271=CARTESIAN_POINT('Ctrl Pts',(0.000248893031568463,-0.20613807668287,
-0.204524541798144));
#33272=CARTESIAN_POINT('Ctrl Pts',(0.0727319195414718,-0.192880883917535,
-0.20081861411912));
#33273=CARTESIAN_POINT('Ctrl Pts',(0.123047552285821,-0.15220372419822,
-0.197112686440096));
#33274=CARTESIAN_POINT('Ctrl Pts',(0.173363185030169,-0.111526564478907,
-0.193406758761072));
#33275=CARTESIAN_POINT('Ctrl Pts',(0.201511424008965,-0.0434294378056156,
-0.189700831082048));
#33276=CARTESIAN_POINT('Ctrl Pts',(0.194601583849065,0.020902114471021,
-0.185994903403024));
#33277=CARTESIAN_POINT('Ctrl Pts',(0.187691743689166,0.0852336667476595,
-0.182288975724));
#33278=CARTESIAN_POINT('Ctrl Pts',(0.145723824390569,0.145799644627643,
-0.178583048044976));
#33279=CARTESIAN_POINT('Ctrl Pts',(0.0879173338961301,0.174863425966255,
-0.174877120365952));
#33280=CARTESIAN_POINT('Ctrl Pts',(0.0301108434016909,0.203927207304867,
-0.171171192686928));
#33281=CARTESIAN_POINT('Ctrl Pts',(-0.0435342182885909,0.201488792102106,
-0.167465265007903));
#33282=CARTESIAN_POINT('Ctrl Pts',(-0.0992916054796352,0.168664897310039,
-0.163759337328879));
#33283=CARTESIAN_POINT('Ctrl Pts',(-0.155048992670679,0.135841002517972,
-0.160053409649855));
#33284=CARTESIAN_POINT('Ctrl Pts',(-0.192918705362486,0.0726316281365982,
-0.156347481970831));
#33285=CARTESIAN_POINT('Ctrl Pts',(-0.195558012150656,0.00798389026030548,
-0.152641554291807));
#33286=CARTESIAN_POINT('Ctrl Pts',(-0.195665928403547,0.00534056677067936,
-0.152490025932012));
#33287=CARTESIAN_POINT('Ctrl Pts',(-0.195714945155934,0.00269483857156378,
-0.152338497572218));
#33288=CARTESIAN_POINT('Ctrl Pts',(-0.195706082681088,4.87745040611329E-5,
-0.152186969212423));
#33289=CARTESIAN_POINT('Origin',(0.,0.,-0.78));
#33290=CARTESIAN_POINT('',(-0.195234571671998,0.00015548015543182,-0.0720130307875768));
#33291=CARTESIAN_POINT('',(-0.195211655640432,0.00014838930625368,-0.0821869692124233));
#33292=CARTESIAN_POINT('',(-0.1954,-2.39295984553393E-17,-0.78));
#33293=CARTESIAN_POINT('Ctrl Pts',(-0.195234571671998,0.00015548015543182,
-0.0720130307875768));
#33294=CARTESIAN_POINT('Ctrl Pts',(-0.195395484933967,0.0211022265122616,
-0.0732049922535051));
#33295=CARTESIAN_POINT('Ctrl Pts',(-0.192293783362919,0.0420031688312999,
-0.0743969537194334));
#33296=CARTESIAN_POINT('Ctrl Pts',(-0.185729534825066,0.0617520264313488,
-0.0755889151853617));
#33297=CARTESIAN_POINT('Ctrl Pts',(-0.165320628124816,0.123153204322723,
-0.0792948428643858));
#33298=CARTESIAN_POINT('Ctrl Pts',(-0.11144099628659,0.173417750325887,
-0.08300077054341));
#33299=CARTESIAN_POINT('Ctrl Pts',(-0.0487793746833237,0.189541935775739,
-0.0867066982224341));
#33300=CARTESIAN_POINT('Ctrl Pts',(0.013882246919943,0.205666121225591,
-0.0904126259014582));
#33301=CARTESIAN_POINT('Ctrl Pts',(0.0853258582882511,0.18764994612213,
-0.0941185535804823));
#33302=CARTESIAN_POINT('Ctrl Pts',(0.132840815824477,0.143736024314436,
-0.0978244812595064));
#33303=CARTESIAN_POINT('Ctrl Pts',(0.180355773360702,0.0998221025067421,
-0.10153040893853));
#33304=CARTESIAN_POINT('Ctrl Pts',(0.203942077064845,0.0300104339948153,
-0.105236336617555));
#33305=CARTESIAN_POINT('Ctrl Pts',(0.192794301808586,-0.0337240337379463,
-0.108942264296579));
#33306=CARTESIAN_POINT('Ctrl Pts',(0.181646526552325,-0.0974585014707116,
-0.112648191975603));
#33307=CARTESIAN_POINT('Ctrl Pts',(0.135764672335656,-0.155115768424311,
-0.116354119654627));
#33308=CARTESIAN_POINT('Ctrl Pts',(0.0761627075839468,-0.180293504362447,
-0.120060047333651));
#33309=CARTESIAN_POINT('Ctrl Pts',(0.0165607428322397,-0.205471240300582,
-0.123765975012675));
#33310=CARTESIAN_POINT('Ctrl Pts',(-0.0567613324545061,-0.198169445223256,
-0.1274719026917));
#33311=CARTESIAN_POINT('Ctrl Pts',(-0.110226248531205,-0.161730863862512,
-0.131177830370724));
#33312=CARTESIAN_POINT('Ctrl Pts',(-0.162332237560633,-0.126218448245754,
-0.134789563843008));
#33313=CARTESIAN_POINT('Ctrl Pts',(-0.195577664726791,-0.0630315725321448,
-0.138401297315292));
#33314=CARTESIAN_POINT('Ctrl Pts',(-0.195715103822041,3.06823192254271E-5,
-0.142013030787576));
#33315=CARTESIAN_POINT('Ctrl Pts',(-0.195706082681088,4.87745040611329E-5,
-0.152186969212423));
#33316=CARTESIAN_POINT('Ctrl Pts',(-0.195498195691465,-0.0620199255922364,
-0.148632569893194));
#33317=CARTESIAN_POINT('Ctrl Pts',(-0.163443397744359,-0.124273430689011,
-0.145078170573964));
#33318=CARTESIAN_POINT('Ctrl Pts',(-0.112710100455115,-0.160009726727084,
-0.141523771254734));
#33319=CARTESIAN_POINT('Ctrl Pts',(-0.0598139810868729,-0.197269504466969,
-0.13781784357571));
#33320=CARTESIAN_POINT('Ctrl Pts',(0.0133871585341446,-0.205702958575528,
-0.134111915896686));
#33321=CARTESIAN_POINT('Ctrl Pts',(0.0733704787706765,-0.181448122744779,
-0.130405988217662));
#33322=CARTESIAN_POINT('Ctrl Pts',(0.133353799007208,-0.157193286914031,
-0.126700060538638));
#33323=CARTESIAN_POINT('Ctrl Pts',(0.180119299859255,-0.100250161143975,
-0.122994132859614));
#33324=CARTESIAN_POINT('Ctrl Pts',(0.192250155136095,-0.0366958770406265,
-0.11928820518059));
#33325=CARTESIAN_POINT('Ctrl Pts',(0.204381010412935,0.026858407062722,
-0.115582277501566));
#33326=CARTESIAN_POINT('Ctrl Pts',(0.181877220114569,0.0970238494993633,
-0.111876349822541));
#33327=CARTESIAN_POINT('Ctrl Pts',(0.135045011563638,0.141667005659141,
-0.108170422143517));
#33328=CARTESIAN_POINT('Ctrl Pts',(0.0882128030127068,0.186310161818919,
-0.104464494464493));
#33329=CARTESIAN_POINT('Ctrl Pts',(0.0170521762092105,0.205431031701833,
-0.100758566785469));
#33330=CARTESIAN_POINT('Ctrl Pts',(-0.0458492466208386,0.190274405722975,
-0.0970526391064448));
#33331=CARTESIAN_POINT('Ctrl Pts',(-0.108750669450888,0.175117779744117,
-0.0933467114274207));
#33332=CARTESIAN_POINT('Ctrl Pts',(-0.16339288830749,0.125683657903486,
-0.0896407837483966));
#33333=CARTESIAN_POINT('Ctrl Pts',(-0.184750451385629,0.0646082163317357,
-0.0859348560693725));
#33334=CARTESIAN_POINT('Ctrl Pts',(-0.191950243798388,0.0440192334395667,
-0.0846855604503894));
#33335=CARTESIAN_POINT('Ctrl Pts',(-0.195367521513062,0.0221073147393436,
-0.0834362648314064));
#33336=CARTESIAN_POINT('Ctrl Pts',(-0.195211655640432,0.00014838930625368,
-0.0821869692124233));
#33337=CARTESIAN_POINT('Origin',(0.,0.,-1.69400562256037));
#33338=CARTESIAN_POINT('',(-0.155418309230191,0.000123771433864409,-0.0490056225603702));
#33339=CARTESIAN_POINT('',(-0.155328830661012,-0.000161474934390352,-0.0351943774396294));
#33340=CARTESIAN_POINT('',(-0.15555,-7.70311135908521E-15,-1.69400562256037));
#33341=CARTESIAN_POINT('',(0.133820275402922,-0.0797997733406099,-0.0200000000000001));
#33342=CARTESIAN_POINT('Ctrl Pts',(-0.155418309230191,0.000123771433864406,
-0.0490056225603702));
#33343=CARTESIAN_POINT('Ctrl Pts',(-0.155148140851959,-0.0350451663106925,
-0.0464916563472745));
#33344=CARTESIAN_POINT('Ctrl Pts',(-0.125895296854632,-0.122459193602597,
-0.0402717624551546));
#33345=CARTESIAN_POINT('Ctrl Pts',(0.0153022004281231,-0.181264675260222,
-0.030603221601698));
#33346=CARTESIAN_POINT('Ctrl Pts',(0.10904323201914,-0.120867443416895,
-0.023448646961337));
#33347=CARTESIAN_POINT('Ctrl Pts',(0.133821766704343,-0.0798002879704671,
-0.0200000000000001));
#33348=CARTESIAN_POINT('',(-0.0319621170202007,-0.152230829911641,-0.02));
#33349=CARTESIAN_POINT('Origin',(0.,0.,-0.02));
#33350=CARTESIAN_POINT('Ctrl Pts',(-0.155328830661012,-0.000161474934390372,
-0.0351943774396294));
#33351=CARTESIAN_POINT('Ctrl Pts',(-0.155437122863521,-0.0191944279743207,
-0.0338355126387771));
#33352=CARTESIAN_POINT('Ctrl Pts',(-0.14338792007184,-0.089950127265619,
-0.0287707201589006));
#33353=CARTESIAN_POINT('Ctrl Pts',(-0.0826006812134621,-0.141598846131356,
-0.0237059276790242));
#33354=CARTESIAN_POINT('Ctrl Pts',(-0.0319621170202007,-0.152230829911641,
-0.02));
#33355=CARTESIAN_POINT('Origin',(0.,0.,-1.69400562256037));
#33356=CARTESIAN_POINT('',(-0.15580084134861,2.44249475701479E-5,-0.11900562256037));
#33357=CARTESIAN_POINT('',(-0.155400066708645,0.000118126696958647,-0.105194377439629));
#33358=CARTESIAN_POINT('',(-0.15555,-7.70311135908521E-15,-1.69400562256037));
#33359=CARTESIAN_POINT('Ctrl Pts',(-0.15580084134861,2.44249475701479E-5,
-0.11900562256037));
#33360=CARTESIAN_POINT('Ctrl Pts',(-0.155691431669664,-0.0501768736303758,
-0.115393889088086));
#33361=CARTESIAN_POINT('Ctrl Pts',(-0.10207054701376,-0.15208972189888,
-0.108076227936777));
#33362=CARTESIAN_POINT('Ctrl Pts',(0.0715520591525512,-0.169379967518084,
-0.0970526391064447));
#33363=CARTESIAN_POINT('Ctrl Pts',(0.181126098406431,-0.0316841454920027,
-0.0859348560693724));
#33364=CARTESIAN_POINT('Ctrl Pts',(0.124797804529567,0.135038552108262,
-0.0748170730322999));
#33365=CARTESIAN_POINT('Ctrl Pts',(-0.0458222632545728,0.17806438686788,
-0.0636992899952276));
#33366=CARTESIAN_POINT('Ctrl Pts',(-0.145400467791554,0.0851674409887763,
-0.055095473171251));
#33367=CARTESIAN_POINT('Ctrl Pts',(-0.155546405739399,0.0167986250459671,
-0.0501975840262985));
#33368=CARTESIAN_POINT('Ctrl Pts',(-0.155418309230191,0.000123771433864406,
-0.0490056225603702));
#33369=CARTESIAN_POINT('Ctrl Pts',(-0.155400066708645,0.000118126696958645,
-0.105194377439629));
#33370=CARTESIAN_POINT('Ctrl Pts',(-0.155156077066721,-0.0342559813938016,
-0.102737745379588));
#33371=CARTESIAN_POINT('Ctrl Pts',(-0.126953063311157,-0.120847780513784,
-0.0965751856405233));
#33372=CARTESIAN_POINT('Ctrl Pts',(0.016274431326597,-0.183144050045734,
-0.0867066982224341));
#33373=CARTESIAN_POINT('Ctrl Pts',(0.162746700955473,-0.0856111115207315,
-0.0755889151853617));
#33374=CARTESIAN_POINT('Ctrl Pts',(0.160120950075793,0.0903886722456795,
-0.0644711321482895));
#33375=CARTESIAN_POINT('Ctrl Pts',(0.0109069706335314,0.18349634534749,
-0.0533533491112173));
#33376=CARTESIAN_POINT('Ctrl Pts',(-0.128953969743316,0.117874527456855,
-0.0435944308749972));
#33377=CARTESIAN_POINT('Ctrl Pts',(-0.155141785851002,0.0327126840798016,
-0.0375414403178012));
#33378=CARTESIAN_POINT('Ctrl Pts',(-0.155328830661012,-0.000161474934390372,
-0.0351943774396294));
#33379=CARTESIAN_POINT('Origin',(0.,0.,-1.69400562256037));
#33380=CARTESIAN_POINT('',(-0.155491490480251,-0.00014012651520363,-0.18900562256037));
#33381=CARTESIAN_POINT('',(-0.155793659984868,3.88274007404833E-5,-0.175194377439629));
#33382=CARTESIAN_POINT('',(-0.15555,-7.70311135908521E-15,-1.69400562256037));
#33383=CARTESIAN_POINT('Ctrl Pts',(-0.155491490480251,-0.000140126515203627,
-0.18900562256037));
#33384=CARTESIAN_POINT('Ctrl Pts',(-0.155614289691432,-0.0141613790019463,
-0.188002049507921));
#33385=CARTESIAN_POINT('Ctrl Pts',(-0.147449247613328,-0.0798188625535115,
-0.183292548776449));
#33386=CARTESIAN_POINT('Ctrl Pts',(-0.0547994747530945,-0.175518602770541,
-0.174877120365952));
#33387=CARTESIAN_POINT('Ctrl Pts',(0.11779346570166,-0.141189404725702,
-0.163759337328879));
#33388=CARTESIAN_POINT('Ctrl Pts',(0.182497816472988,0.0224570410225731,
-0.152641554291807));
#33389=CARTESIAN_POINT('Ctrl Pts',(0.080049763103335,0.16553491873334,-0.141523771254734));
#33390=CARTESIAN_POINT('Ctrl Pts',(-0.0957167152029026,0.156996802481032,
-0.130405988217662));
#33391=CARTESIAN_POINT('Ctrl Pts',(-0.155195594339883,0.054150759132695,
-0.122899938652874));
#33392=CARTESIAN_POINT('Ctrl Pts',(-0.155803694759029,0.00133367756356404,
-0.11909981676711));
#33393=CARTESIAN_POINT('Ctrl Pts',(-0.15580084134861,2.44249475701479E-5,
-0.11900562256037));
#33394=CARTESIAN_POINT('Ctrl Pts',(-0.155793659984868,3.88274007404889E-5,
-0.175194377439629));
#33395=CARTESIAN_POINT('Ctrl Pts',(-0.155628169599829,-0.0493715426093849,
-0.1716399781204));
#33396=CARTESIAN_POINT('Ctrl Pts',(-0.10350528241731,-0.150599209937992,
-0.164379651122146));
#33397=CARTESIAN_POINT('Ctrl Pts',(0.0689294256808382,-0.170465296791246,
-0.153413396444868));
#33398=CARTESIAN_POINT('Ctrl Pts',(0.18061377047412,-0.0344749710973018,
-0.142295613407796));
#33399=CARTESIAN_POINT('Ctrl Pts',(0.126870711401792,0.133092601640971,
-0.131177830370724));
#33400=CARTESIAN_POINT('Ctrl Pts',(-0.0430735388430987,0.178756644275882,
-0.120060047333651));
#33401=CARTESIAN_POINT('Ctrl Pts',(-0.144734088084764,0.0867856357268612,
-0.11139889635662));
#33402=CARTESIAN_POINT('Ctrl Pts',(-0.1555241451963,0.0175987349421875,
-0.106443673058612));
#33403=CARTESIAN_POINT('Ctrl Pts',(-0.155400066708645,0.000118126696958645,
-0.105194377439629));
#33404=CARTESIAN_POINT('Origin',(0.,0.,-1.69400562256037));
#33405=CARTESIAN_POINT('',(-0.155313230688262,5.57501280555406E-5,-0.259005622560369));
#33406=CARTESIAN_POINT('',(-0.155514994383668,-0.000141972556441383,-0.245194377439629));
#33407=CARTESIAN_POINT('',(-0.15555,-7.70311135908521E-15,-1.69400562256037));
#33408=CARTESIAN_POINT('Ctrl Pts',(-0.155313230688262,5.57501280555421E-5,
-0.259005622560369));
#33409=CARTESIAN_POINT('Ctrl Pts',(-0.155218500888833,-0.02938770921547,
-0.256904282248733));
#33410=CARTESIAN_POINT('Ctrl Pts',(-0.132999364931809,-0.110890237651056,
-0.251097014258072));
#33411=CARTESIAN_POINT('Ctrl Pts',(-0.0012905770009465,-0.183869774559952,
-0.241583818588386));
#33412=CARTESIAN_POINT('Ctrl Pts',(0.153815542361654,-0.100749879415303,
-0.230466035551314));
#33413=CARTESIAN_POINT('Ctrl Pts',(0.168039885229795,0.0746482190809691,
-0.219348252514241));
#33414=CARTESIAN_POINT('Ctrl Pts',(0.0283541753201865,0.181674986598733,
-0.208230469477169));
#33415=CARTESIAN_POINT('Ctrl Pts',(-0.122348206378289,0.127662463104303,
-0.198116259492545));
#33416=CARTESIAN_POINT('Ctrl Pts',(-0.155160824949062,0.0376153676518437,
-0.191707977186946));
#33417=CARTESIAN_POINT('Ctrl Pts',(-0.155491490480251,-0.000140126515203627,
-0.18900562256037));
#33418=CARTESIAN_POINT('Ctrl Pts',(-0.155514994383668,-0.000141972556441401,
-0.245194377439629));
#33419=CARTESIAN_POINT('Ctrl Pts',(-0.155633762438056,-0.0133571067813652,
-0.244248138540235));
#33420=CARTESIAN_POINT('Ctrl Pts',(-0.148042855299553,-0.0781946520382958,
-0.239595971961817));
#33421=CARTESIAN_POINT('Ctrl Pts',(-0.0575026584572911,-0.174651658969645,
-0.231237877704375));
#33422=CARTESIAN_POINT('Ctrl Pts',(0.115599717800877,-0.142991121590197,
-0.220120094667303));
#33423=CARTESIAN_POINT('Ctrl Pts',(0.182822725577002,0.0196369447459957,
-0.209002311630231));
#33424=CARTESIAN_POINT('Ctrl Pts',(0.0825958599644629,0.164279286494686,
-0.197884528593158));
#33425=CARTESIAN_POINT('Ctrl Pts',(-0.0932816632585158,0.158455916717979,
-0.186766745556086));
#33426=CARTESIAN_POINT('Ctrl Pts',(-0.154807377033864,0.0557616631925561,
-0.179203361838243));
#33427=CARTESIAN_POINT('Ctrl Pts',(-0.15580071504097,0.0021452514831387,
-0.175345905799424));
#33428=CARTESIAN_POINT('Ctrl Pts',(-0.155793659984868,3.88274007404889E-5,
-0.175194377439629));
#33429=CARTESIAN_POINT('Origin',(0.,0.,-1.69400562256037));
#33430=CARTESIAN_POINT('',(-0.155695864222888,0.0001123590686367,-0.32900562256037));
#33431=CARTESIAN_POINT('',(-0.155305573486524,4.33443872281669E-5,-0.315194377439629));
#33432=CARTESIAN_POINT('',(-0.15555,-7.70311135908521E-15,-1.69400562256037));
#33433=CARTESIAN_POINT('Ctrl Pts',(-0.155695864222888,0.000112359068636702,
-0.32900562256037));
#33434=CARTESIAN_POINT('Ctrl Pts',(-0.155333113201872,-0.044432697078968,
-0.325806514989544));
#33435=CARTESIAN_POINT('Ctrl Pts',(-0.111918636618463,-0.141197251894673,
-0.318901479739694));
#33436=CARTESIAN_POINT('Ctrl Pts',(0.0523302865754574,-0.176270532440662,
-0.30829051681082));
#33437=CARTESIAN_POINT('Ctrl Pts',(0.176494333858419,-0.0515704334810062,
-0.297172733773748));
#33438=CARTESIAN_POINT('Ctrl Pts',(0.139004785069224,0.12036373717149,-0.286054950736676));
#33439=CARTESIAN_POINT('Ctrl Pts',(-0.0258011647703144,0.182055099924714,
-0.274937167699603));
#33440=CARTESIAN_POINT('Ctrl Pts',(-0.140292520438531,0.0968559071634296,
-0.265920724974167));
#33441=CARTESIAN_POINT('Ctrl Pts',(-0.155385566539166,0.0225388304045638,
-0.260610209927757));
#33442=CARTESIAN_POINT('Ctrl Pts',(-0.155313230688262,5.57501280555421E-5,
-0.259005622560369));
#33443=CARTESIAN_POINT('Ctrl Pts',(-0.155305573486524,4.33443872281461E-5,
-0.315194377439629));
#33444=CARTESIAN_POINT('Ctrl Pts',(-0.155234133047627,-0.0286002858100627,
-0.313150371281046));
#33445=CARTESIAN_POINT('Ctrl Pts',(-0.133908567567703,-0.10927577092568,
-0.30740043744344));
#33446=CARTESIAN_POINT('Ctrl Pts',(-0.00412905838771584,-0.183827930642512,
-0.29794457592681));
#33447=CARTESIAN_POINT('Ctrl Pts',(0.152241800199334,-0.103112518319205,
-0.286826792889737));
#33448=CARTESIAN_POINT('Ctrl Pts',(0.169172293136615,0.0720450722777397,
-0.275709009852665));
#33449=CARTESIAN_POINT('Ctrl Pts',(0.031155547779449,0.181215587419735,
-0.264591226815592));
#33450=CARTESIAN_POINT('Ctrl Pts',(-0.12122164066584,0.129243139587191,
-0.254419682677914));
#33451=CARTESIAN_POINT('Ctrl Pts',(-0.155168609483109,0.0383997294019111,
-0.247954066219259));
#33452=CARTESIAN_POINT('Ctrl Pts',(-0.155514994383668,-0.000141972556441401,
-0.245194377439629));
#33453=CARTESIAN_POINT('Origin',(0.,0.,-1.69400562256037));
#33454=CARTESIAN_POINT('',(-0.155663515357411,-0.000123932043195673,-0.39900562256037));
#33455=CARTESIAN_POINT('',(-0.155674050643768,0.000120533321258946,-0.385194377439629));
#33456=CARTESIAN_POINT('',(-0.15555,-7.70311135908521E-15,-1.69400562256037));
#33457=CARTESIAN_POINT('Ctrl Pts',(-0.155663515357411,-0.000123932043195673,
-0.39900562256037));
#33458=CARTESIAN_POINT('Ctrl Pts',(-0.155735158257095,-0.00835685638452879,
-0.39841467540938));
#33459=CARTESIAN_POINT('Ctrl Pts',(-0.1513960673005,-0.068144160838432,
-0.394117800579365));
#33460=CARTESIAN_POINT('Ctrl Pts',(-0.0739236171314337,-0.168359907127257,
-0.386114998070327));
#33461=CARTESIAN_POINT('Ctrl Pts',(0.101411577137068,-0.153380088408926,
-0.374997215033255));
#33462=CARTESIAN_POINT('Ctrl Pts',(0.183862508367636,0.00208267001642915,
-0.363879431996182));
#33463=CARTESIAN_POINT('Ctrl Pts',(0.0979112307772101,0.155637882230987,
-0.35276164895911));
#33464=CARTESIAN_POINT('Ctrl Pts',(-0.0777182943142881,0.166642210219781,
-0.341643865922037));
#33465=CARTESIAN_POINT('Ctrl Pts',(-0.152110471914154,0.0657689570239066,
-0.333725190455791));
#33466=CARTESIAN_POINT('Ctrl Pts',(-0.155753333222491,0.00716943035386869,
-0.329512442668568));
#33467=CARTESIAN_POINT('Ctrl Pts',(-0.155695864222888,0.000112359068636702,
-0.32900562256037));
#33468=CARTESIAN_POINT('Ctrl Pts',(-0.155674050643768,0.00012053332125895,
-0.385194377439629));
#33469=CARTESIAN_POINT('Ctrl Pts',(-0.155300039098235,-0.0436421499872883,
-0.382052604021858));
#33470=CARTESIAN_POINT('Ctrl Pts',(-0.113200685144466,-0.139655777002699,
-0.375204902925063));
#33471=CARTESIAN_POINT('Ctrl Pts',(0.0496027324589358,-0.177057409124813,
-0.364651274149244));
#33472=CARTESIAN_POINT('Ctrl Pts',(0.175677134346707,-0.054289056541952,
-0.353533491112171));
#33473=CARTESIAN_POINT('Ctrl Pts',(0.140846424445151,0.118203392142091,
-0.342415708075099));
#33474=CARTESIAN_POINT('Ctrl Pts',(-0.0229874693739835,0.182431722699479,
-0.331297925038026));
#33475=CARTESIAN_POINT('Ctrl Pts',(-0.139516816184985,0.0984797733671933,
-0.322224148159537));
#33476=CARTESIAN_POINT('Ctrl Pts',(-0.155363659614267,0.0233326408742186,
-0.316856298960071));
#33477=CARTESIAN_POINT('Ctrl Pts',(-0.155305573486524,4.33443872281461E-5,
-0.315194377439629));
#33478=CARTESIAN_POINT('Origin',(0.,0.,-1.69400562256037));
#33479=CARTESIAN_POINT('',(-0.155302671155773,-3.74165374094889E-5,-0.46900562256037));
#33480=CARTESIAN_POINT('',(-0.155685804724859,-0.000116329614590766,-0.455194377439629));
#33481=CARTESIAN_POINT('',(-0.15555,-7.70311135908521E-15,-1.69400562256037));
#33482=CARTESIAN_POINT('Ctrl Pts',(-0.155302671155773,-3.74165374095008E-5,
-0.46900562256037));
#33483=CARTESIAN_POINT('Ctrl Pts',(-0.155353567981131,-0.0237032812024999,
-0.467316908150191));
#33484=CARTESIAN_POINT('Ctrl Pts',(-0.139148552154265,-0.0992383841234035,
-0.461922266060988));
#33485=CARTESIAN_POINT('Ctrl Pts',(-0.0216706798754521,-0.182592828806171,
-0.452821696292762));
#33486=CARTESIAN_POINT('Ctrl Pts',(0.141695566734905,-0.117184153644509,
-0.441703913255688));
#33487=CARTESIAN_POINT('Ctrl Pts',(0.175280888292921,0.0555551050484869,
-0.430586130218617));
#33488=CARTESIAN_POINT('Ctrl Pts',(0.0483240252869895,0.177410676335346,
-0.419468347181544));
#33489=CARTESIAN_POINT('Ctrl Pts',(-0.113792699461829,0.138933369296078,
-0.408941511295462));
#33490=CARTESIAN_POINT('Ctrl Pts',(-0.155285873740701,0.0432731787966904,
-0.402120603088404));
#33491=CARTESIAN_POINT('Ctrl Pts',(-0.155663515357411,-0.000123932043195673,
-0.39900562256037));
#33492=CARTESIAN_POINT('Ctrl Pts',(-0.155685804724859,-0.000116329614590777,
-0.455194377439629));
#33493=CARTESIAN_POINT('Ctrl Pts',(-0.155747810222891,-0.00754772143374497,
-0.454660764441694));
#33494=CARTESIAN_POINT('Ctrl Pts',(-0.15188616619471,-0.0665251955223991,
-0.450421223764734));
#33495=CARTESIAN_POINT('Ctrl Pts',(-0.0765139937801866,-0.167198582376871,
-0.44247575540875));
#33496=CARTESIAN_POINT('Ctrl Pts',(0.0990315612963532,-0.154927425139147,
-0.431357972371679));
#33497=CARTESIAN_POINT('Ctrl Pts',(0.183872742689355,-0.000756101129370498,
-0.420240189334605));
#33498=CARTESIAN_POINT('Ctrl Pts',(0.100302341504276,0.154107746339307,
-0.409122406297534));
#33499=CARTESIAN_POINT('Ctrl Pts',(-0.0751363584943781,0.167822182161027,
-0.398004623260461));
#33500=CARTESIAN_POINT('Ctrl Pts',(-0.15162681660732,0.0673874850065461,
-0.390028613641159));
#33501=CARTESIAN_POINT('Ctrl Pts',(-0.155741210231399,0.00797880347299771,
-0.385758531700882));
#33502=CARTESIAN_POINT('Ctrl Pts',(-0.155674050643768,0.00012053332125895,
-0.385194377439629));
#33503=CARTESIAN_POINT('Origin',(0.,0.,-1.69400562256037));
#33504=CARTESIAN_POINT('',(-0.155526161619123,0.000142390113939882,-0.53900562256037));
#33505=CARTESIAN_POINT('',(-0.155309408901357,-5.00045343397038E-5,-0.525194377439629));
#33506=CARTESIAN_POINT('',(-0.15555,-7.70311135908521E-15,-1.69400562256037));
#33507=CARTESIAN_POINT('Ctrl Pts',(-0.155526161619123,0.000142390113939881,
-0.53900562256037));
#33508=CARTESIAN_POINT('Ctrl Pts',(-0.155173230571418,-0.0387663839332682,
-0.536219140891002));
#33509=CARTESIAN_POINT('Ctrl Pts',(-0.120688392748538,-0.129980358346068,
-0.529726731542611));
#33510=CARTESIAN_POINT('Ctrl Pts',(0.032462156090606,-0.180986098691733,
-0.519528394515196));
#33511=CARTESIAN_POINT('Ctrl Pts',(0.169687680181897,-0.0708226707501974,
-0.508410611478123));
#33512=CARTESIAN_POINT('Ctrl Pts',(0.151493916207583,0.104208218724794,
-0.497292828441051));
#33513=CARTESIAN_POINT('Ctrl Pts',(-0.00545521632391679,0.183793362536746,
-0.486175045403978));
#33514=CARTESIAN_POINT('Ctrl Pts',(-0.13432728737953,0.108520707887271,
-0.476745976777085));
#33515=CARTESIAN_POINT('Ctrl Pts',(-0.155241873574587,0.0282320741078864,
-0.471022835829215));
#33516=CARTESIAN_POINT('Ctrl Pts',(-0.155302671155773,-3.74165374095008E-5,
-0.46900562256037));
#33517=CARTESIAN_POINT('Ctrl Pts',(-0.155309408901357,-5.00045343397228E-5,
-0.525194377439629));
#33518=CARTESIAN_POINT('Ctrl Pts',(-0.155375280949092,-0.0229099022660926,
-0.523562997182505));
#33519=CARTESIAN_POINT('Ctrl Pts',(-0.139932112659729,-0.0976148396626936,
-0.518225689246357));
#33520=CARTESIAN_POINT('Ctrl Pts',(-0.0244870176639766,-0.182236503365697,
-0.509182453631186));
#33521=CARTESIAN_POINT('Ctrl Pts',(0.139869551941277,-0.119357721295182,
-0.498064670594112));
#33522=CARTESIAN_POINT('Ctrl Pts',(0.176117668643726,0.0528424449143884,
-0.486946887557041));
#33523=CARTESIAN_POINT('Ctrl Pts',(0.0510571821108666,0.176643486570915,
-0.475829104519967));
#33524=CARTESIAN_POINT('Ctrl Pts',(-0.112520335133757,0.140477662351258,
-0.465244934480831));
#33525=CARTESIAN_POINT('Ctrl Pts',(-0.155317183734598,0.0440630915390226,
-0.458366692120718));
#33526=CARTESIAN_POINT('Ctrl Pts',(-0.155685804724859,-0.000116329614590777,
-0.455194377439629));
#33527=CARTESIAN_POINT('Origin',(0.,0.,-1.69400562256037));
#33528=CARTESIAN_POINT('',(-0.155789325782022,-4.54178512007087E-5,-0.60900562256037));
#33529=CARTESIAN_POINT('',(-0.15550239893659,0.000141150492465145,-0.595194377439629));
#33530=CARTESIAN_POINT('',(-0.15555,-7.70311135908521E-15,-1.69400562256037));
#33531=CARTESIAN_POINT('Ctrl Pts',(-0.155789325782022,-4.54178512007122E-5,
-0.60900562256037));
#33532=CARTESIAN_POINT('Ctrl Pts',(-0.155798887408862,-0.00252447849977371,
-0.608827301310838));
#33533=CARTESIAN_POINT('Ctrl Pts',(-0.154621603582211,-0.0565148725602989,
-0.604943052382282));
#33534=CARTESIAN_POINT('Ctrl Pts',(-0.0921360414391275,-0.159124823222627,
-0.597352875774703));
#33535=CARTESIAN_POINT('Ctrl Pts',(0.0837789491030789,-0.163679098191823,
-0.58623509273763));
#33536=CARTESIAN_POINT('Ctrl Pts',(0.182959643964377,-0.01831742826199,
-0.575117309700558));
#33537=CARTESIAN_POINT('Ctrl Pts',(0.114565075971008,0.143821427003983,
-0.563999526663485));
#33538=CARTESIAN_POINT('Ctrl Pts',(-0.0587612261677574,0.174232252459085,
-0.552881743626413));
#33539=CARTESIAN_POINT('Ctrl Pts',(-0.14831515963045,0.0774358242001071,
-0.544550442258708));
#33540=CARTESIAN_POINT('Ctrl Pts',(-0.155642617093086,0.012980987773357,
-0.539925068570027));
#33541=CARTESIAN_POINT('Ctrl Pts',(-0.155526161619123,0.000142390113939881,
-0.53900562256037));
#33542=CARTESIAN_POINT('Ctrl Pts',(-0.15550239893659,0.000141150492465129,
-0.595194377439629));
#33543=CARTESIAN_POINT('Ctrl Pts',(-0.155164110590692,-0.0379818716864814,
-0.592465229923317));
#33544=CARTESIAN_POINT('Ctrl Pts',(-0.121824210522794,-0.128401648628898,
-0.58603015472798));
#33545=CARTESIAN_POINT('Ctrl Pts',(0.0296641702068159,-0.181465683254363,
-0.575889151853619));
#33546=CARTESIAN_POINT('Ctrl Pts',(0.168574070457431,-0.0734339156142763,
-0.564771368816547));
#33547=CARTESIAN_POINT('Ctrl Pts',(0.153084653157532,0.101856988766946,
-0.553653585779474));
#33548=CARTESIAN_POINT('Ctrl Pts',(-0.00261711062509075,0.183855671451842,
-0.542535802742403));
#33549=CARTESIAN_POINT('Ctrl Pts',(-0.133426488682267,0.110136005965318,
-0.533049399962453));
#33550=CARTESIAN_POINT('Ctrl Pts',(-0.155225642602111,0.0290198225015199,
-0.527268924861529));
#33551=CARTESIAN_POINT('Ctrl Pts',(-0.155309408901357,-5.00045343397228E-5,
-0.525194377439629));
#33552=CARTESIAN_POINT('Origin',(0.,0.,-1.69400562256037));
#33553=CARTESIAN_POINT('',(-0.155391605265501,-0.00011484305413676,-0.67900562256037));
#33554=CARTESIAN_POINT('',(-0.15579782156367,-3.11631852267236E-5,-0.665194377439629));
#33555=CARTESIAN_POINT('',(-0.15555,-7.70311135908521E-15,-1.69400562256037));
#33556=CARTESIAN_POINT('Ctrl Pts',(-0.155391605265501,-0.000114843054136771,
-0.67900562256037));
#33557=CARTESIAN_POINT('Ctrl Pts',(-0.155513806205127,-0.0179724822621975,
-0.67772953405165));
#33558=CARTESIAN_POINT('Ctrl Pts',(-0.144419737971622,-0.0875438573516224,
-0.672747517863905));
#33559=CARTESIAN_POINT('Ctrl Pts',(-0.041783515845475,-0.179063947519582,
-0.664059573997137));
#33560=CARTESIAN_POINT('Ctrl Pts',(0.127828044966229,-0.132173183429228,
-0.652941790960064));
#33561=CARTESIAN_POINT('Ctrl Pts',(0.180360135293257,0.0357768234294574,
-0.641824007922992));
#33562=CARTESIAN_POINT('Ctrl Pts',(0.0676978886322038,0.170958343968484,
-0.630706224885919));
#33563=CARTESIAN_POINT('Ctrl Pts',(-0.104168244489674,0.149900024002337,
-0.619766763098379));
#33564=CARTESIAN_POINT('Ctrl Pts',(-0.155600174705506,0.0489961310722934,
-0.612533228989862));
#33565=CARTESIAN_POINT('Ctrl Pts',(-0.155789325782022,-4.54178512007122E-5,
-0.60900562256037));
#33566=CARTESIAN_POINT('Ctrl Pts',(-0.15579782156367,-3.11631852267405E-5,
-0.665194377439629));
#33567=CARTESIAN_POINT('Ctrl Pts',(-0.155802429055179,-0.00171290653077161,
-0.665073390343152));
#33568=CARTESIAN_POINT('Ctrl Pts',(-0.155015687096898,-0.0549033244907316,
-0.661246475567651));
#33569=CARTESIAN_POINT('Ctrl Pts',(-0.0945816730450154,-0.157683430699099,
-0.653713633113126));
#33570=CARTESIAN_POINT('Ctrl Pts',(0.081242036168499,-0.164952989521948,
-0.642595850076053));
#33571=CARTESIAN_POINT('Ctrl Pts',(0.182655043268737,-0.0211398287960793,
-0.631478067038982));
#33572=CARTESIAN_POINT('Ctrl Pts',(0.116771775495109,0.142035592865843,
-0.620360284001909));
#33573=CARTESIAN_POINT('Ctrl Pts',(-0.0560643729717556,0.175118654849549,
-0.609242500964836));
#33574=CARTESIAN_POINT('Ctrl Pts',(-0.147728502578342,0.0790597880150364,
-0.600853865444076));
#33575=CARTESIAN_POINT('Ctrl Pts',(-0.155623474599805,0.0137856352938298,
-0.596171157602341));
#33576=CARTESIAN_POINT('Ctrl Pts',(-0.15550239893659,0.000141150492465129,
-0.595194377439629));
#33577=CARTESIAN_POINT('Origin',(0.,0.,-1.69400562256037));
#33578=CARTESIAN_POINT('',(-0.155374470604174,0.000106635008702182,-0.74900562256037));
#33579=CARTESIAN_POINT('',(-0.15541051600741,-0.000122268189293742,-0.735194377439629));
#33580=CARTESIAN_POINT('',(-0.15555,-7.70311135908521E-15,-1.69400562256037));
#33581=CARTESIAN_POINT('Ctrl Pts',(-0.155374470604174,0.000106635008702186,
-0.74900562256037));
#33582=CARTESIAN_POINT('Ctrl Pts',(-0.155164878665456,-0.0331224170312113,
-0.746631766792461));
#33583=CARTESIAN_POINT('Ctrl Pts',(-0.12842734549985,-0.118534576453168,
-0.740551983345528));
#33584=CARTESIAN_POINT('Ctrl Pts',(0.0121936665653112,-0.183469545138692,
-0.730766272219571));
#33585=CARTESIAN_POINT('Ctrl Pts',(0.160788251222258,-0.0892014448683006,
-0.719648489182499));
#33586=CARTESIAN_POINT('Ctrl Pts',(0.162114657614943,0.0867674897879067,
-0.708530706145426));
#33587=CARTESIAN_POINT('Ctrl Pts',(0.014958011823137,0.183264883106403,
-0.697412923108354));
#33588=CARTESIAN_POINT('Ctrl Pts',(-0.12743588276431,0.120097779836716,
-0.687571228580002));
#33589=CARTESIAN_POINT('Ctrl Pts',(-0.155158918717726,0.0338884341013097,
-0.681435461730674));
#33590=CARTESIAN_POINT('Ctrl Pts',(-0.155391605265501,-0.000114843054136771,
-0.67900562256037));
#33591=CARTESIAN_POINT('Ctrl Pts',(-0.15541051600741,-0.000122268189293732,
-0.735194377439629));
#33592=CARTESIAN_POINT('Ctrl Pts',(-0.155535777391527,-0.0171723439086348,
-0.733975623083964));
#33593=CARTESIAN_POINT('Ctrl Pts',(-0.145086129026133,-0.085918178416682,
-0.729050941049274));
#33594=CARTESIAN_POINT('Ctrl Pts',(-0.0445429760552296,-0.17839753495263,
-0.72042033133556));
#33595=CARTESIAN_POINT('Ctrl Pts',(0.125772278341771,-0.134130873380261,
-0.709302548298488));
#33596=CARTESIAN_POINT('Ctrl Pts',(0.180890967276192,0.032988106203831,
-0.698184765261415));
#33597=CARTESIAN_POINT('Ctrl Pts',(0.0703291228835756,0.169892824061108,
-0.687066982224344));
#33598=CARTESIAN_POINT('Ctrl Pts',(-0.102743979992633,0.151393885647765,
-0.676070186283748));
#33599=CARTESIAN_POINT('Ctrl Pts',(-0.155661298051869,0.0498001836643546,
-0.668779318022176));
#33600=CARTESIAN_POINT('Ctrl Pts',(-0.15579782156367,-3.11631852267405E-5,
-0.665194377439629));
#33601=CARTESIAN_POINT('Origin',(0.,0.,-1.69400562256037));
#33602=CARTESIAN_POINT('',(-0.155778366559592,5.87990317054179E-5,-0.81900562256037));
#33603=CARTESIAN_POINT('',(-0.15535840277364,9.73258243413475E-5,-0.805194377439629));
#33604=CARTESIAN_POINT('',(-0.15555,-7.70311135908521E-15,-1.69400562256037));
#33605=CARTESIAN_POINT('Ctrl Pts',(-0.155778366559592,5.8799031705413E-5,
-0.81900562256037));
#33606=CARTESIAN_POINT('Ctrl Pts',(-0.155544814787508,-0.0482134994294573,
-0.815533999533272));
#33607=CARTESIAN_POINT('Ctrl Pts',(-0.105538280033678,-0.148433709770403,
-0.808356448827152));
#33608=CARTESIAN_POINT('Ctrl Pts',(0.0651130668400682,-0.171959437148373,
-0.797472970442005));
#33609=CARTESIAN_POINT('Ctrl Pts',(0.179800319818854,-0.0384916158499819,
-0.786355187404933));
#33610=CARTESIAN_POINT('Ctrl Pts',(0.129805978528337,0.130231207611715,
-0.775237404367861));
#33611=CARTESIAN_POINT('Ctrl Pts',(-0.039079449893004,0.179673470756717,
-0.764119621330788));
#33612=CARTESIAN_POINT('Ctrl Pts',(-0.143753821336814,0.0891312796984386,
-0.755375694061625));
#33613=CARTESIAN_POINT('Ctrl Pts',(-0.155492081597284,0.0187528760540667,
-0.750337694471485));
#33614=CARTESIAN_POINT('Ctrl Pts',(-0.155374470604174,0.000106635008702186,
-0.74900562256037));
#33615=CARTESIAN_POINT('Ctrl Pts',(-0.15535840277364,9.73258243413457E-5,
-0.805194377439629));
#33616=CARTESIAN_POINT('Ctrl Pts',(-0.155172926064984,-0.0323375807199177,
-0.802877855824775));
#33617=CARTESIAN_POINT('Ctrl Pts',(-0.129424084682119,-0.116930873012904,
-0.796855406530896));
#33618=CARTESIAN_POINT('Ctrl Pts',(0.00935975675220263,-0.183635922810792,
-0.787127029557995));
#33619=CARTESIAN_POINT('Ctrl Pts',(0.159391965553992,-0.0916731067972864,
-0.776009246520922));
#33620=CARTESIAN_POINT('Ctrl Pts',(0.163434873404623,0.0842543728731427,
-0.76489146348385));
#33621=CARTESIAN_POINT('Ctrl Pts',(0.0177855252092632,0.183012109670541,
-0.753773680446777));
#33622=CARTESIAN_POINT('Ctrl Pts',(-0.126401704041202,0.121695716778875,
-0.743874651765371));
#33623=CARTESIAN_POINT('Ctrl Pts',(-0.155154888799535,0.0346726790396201,
-0.737681550762988));
#33624=CARTESIAN_POINT('Ctrl Pts',(-0.15541051600741,-0.000122268189293732,
-0.735194377439629));
#33625=CARTESIAN_POINT('Origin',(0.,0.,-1.69400562256037));
#33626=CARTESIAN_POINT('',(-0.155549735916814,-0.000142332827097759,-0.88900562256037));
#33627=CARTESIAN_POINT('',(-0.155764687078297,7.18096733227647E-5,-0.875194377439629));
#33628=CARTESIAN_POINT('',(-0.15555,-7.70311135908521E-15,-1.69400562256037));
#33629=CARTESIAN_POINT('Ctrl Pts',(-0.155549735916814,-0.00014233282709776,
-0.88900562256037));
#33630=CARTESIAN_POINT('Ctrl Pts',(-0.155660546006807,-0.0121945460934811,
-0.888142159953108));
#33631=CARTESIAN_POINT('Ctrl Pts',(-0.148873723913168,-0.0758506683039087,
-0.883572769666822));
#33632=CARTESIAN_POINT('Ctrl Pts',(-0.0613810315003473,-0.173326652508083,
-0.875297451701512));
#33633=CARTESIAN_POINT('Ctrl Pts',(0.112384007026421,-0.145532108011909,
-0.86417966866444));
#33634=CARTESIAN_POINT('Ctrl Pts',(0.183214982554139,0.0155573026386719,
-0.853061885627367));
#33635=CARTESIAN_POINT('Ctrl Pts',(0.086236827089008,0.162397565102822,
-0.841944102590294));
#33636=CARTESIAN_POINT('Ctrl Pts',(-0.0897268284244655,0.160495656510048,
-0.830826319553223));
#33637=CARTESIAN_POINT('Ctrl Pts',(-0.154224330533382,0.0580895164678045,
-0.823180159543247));
#33638=CARTESIAN_POINT('Ctrl Pts',(-0.155794129292538,0.00331676339026758,
-0.819239927212296));
#33639=CARTESIAN_POINT('Ctrl Pts',(-0.155778366559592,5.8799031705413E-5,
-0.81900562256037));
#33640=CARTESIAN_POINT('Ctrl Pts',(-0.155764687078297,7.18096733227586E-5,
-0.875194377439629));
#33641=CARTESIAN_POINT('Ctrl Pts',(-0.155492443796488,-0.0474143206243747,
-0.871780088565587));
#33642=CARTESIAN_POINT('Ctrl Pts',(-0.106920290789132,-0.146924481715035,
-0.864659872012519));
#33643=CARTESIAN_POINT('Ctrl Pts',(0.0624505448146294,-0.172944172048056,
-0.853833727780429));
#33644=CARTESIAN_POINT('Ctrl Pts',(0.179184640777123,-0.0412628368220751,
-0.842715944743356));
#33645=CARTESIAN_POINT('Ctrl Pts',(0.131801051401358,0.128211700099984,
-0.831598161706284));
#33646=CARTESIAN_POINT('Ctrl Pts',(-0.0363009398827759,0.180255371505702,
-0.820480378669211));
#33647=CARTESIAN_POINT('Ctrl Pts',(-0.143056085809257,0.090756946949155,
-0.811679117246994));
#33648=CARTESIAN_POINT('Ctrl Pts',(-0.155469648212542,0.0195511722958854,
-0.806583783503799));
#33649=CARTESIAN_POINT('Ctrl Pts',(-0.15535840277364,9.73258243413457E-5,
-0.805194377439629));
#33650=CARTESIAN_POINT('Origin',(0.,0.,-1.69400562256037));
#33651=CARTESIAN_POINT('',(-0.155297992403489,2.48232510734268E-5,-0.95900562256037));
#33652=CARTESIAN_POINT('',(-0.155574065889681,-0.000140958060374008,-0.94519437743963));
#33653=CARTESIAN_POINT('',(-0.15555,-7.70311135908521E-15,-1.69400562256037));
#33654=CARTESIAN_POINT('Ctrl Pts',(-0.155297992403489,2.48232510734348E-5,
-0.95900562256037));
#33655=CARTESIAN_POINT('Ctrl Pts',(-0.155258843021101,-0.027462174823301,
-0.95704439269392));
#33656=CARTESIAN_POINT('Ctrl Pts',(-0.135189599997863,-0.106941847650722,
-0.951377235148446));
#33657=CARTESIAN_POINT('Ctrl Pts',(-0.00822520867957112,-0.183690243180965,
-0.942004149923946));
#33658=CARTESIAN_POINT('Ctrl Pts',(0.14990580454341,-0.106480088570106,
-0.930886366886874));
#33659=CARTESIAN_POINT('Ctrl Pts',(0.170736022599271,0.0682566486482162,
-0.919768583849802));
#33660=CARTESIAN_POINT('Ctrl Pts',(0.0351867613017287,0.18047617938886,
-0.908650800812729));
#33661=CARTESIAN_POINT('Ctrl Pts',(-0.119560116328767,0.13151762975358,
-0.898396480382919));
#33662=CARTESIAN_POINT('Ctrl Pts',(-0.155184956008855,0.0395328018678041,
-0.891848087632132));
#33663=CARTESIAN_POINT('Ctrl Pts',(-0.155549735916814,-0.00014233282709776,
-0.88900562256037));
#33664=CARTESIAN_POINT('Ctrl Pts',(-0.155574065889681,-0.000140958060374001,
-0.94519437743963));
#33665=CARTESIAN_POINT('Ctrl Pts',(-0.155678059406658,-0.0113883944085503,
-0.944388248985422));
#33666=CARTESIAN_POINT('Ctrl Pts',(-0.149431301112879,-0.0742278940490436,
-0.939876192852191));
#33667=CARTESIAN_POINT('Ctrl Pts',(-0.0640495814302482,-0.172358371748057,
-0.931658209039936));
#33668=CARTESIAN_POINT('Ctrl Pts',(0.110123842548254,-0.147249775875683,
-0.920540426002863));
#33669=CARTESIAN_POINT('Ctrl Pts',(0.183433319364821,0.0127269218523267,
-0.909422642965792));
#33670=CARTESIAN_POINT('Ctrl Pts',(0.0887336874904625,0.161046856216992,
-0.898304859928718));
#33671=CARTESIAN_POINT('Ctrl Pts',(-0.0872383533320315,0.16186175243382,
-0.887187076891646));
#33672=CARTESIAN_POINT('Ctrl Pts',(-0.153804569176776,0.0597032248363634,
-0.879483582728616));
#33673=CARTESIAN_POINT('Ctrl Pts',(-0.155787941321947,0.00412793931088879,
-0.875486016244611));
#33674=CARTESIAN_POINT('Ctrl Pts',(-0.155764687078297,7.18096733227586E-5,
-0.875194377439629));
#33675=CARTESIAN_POINT('Origin',(0.,0.,-1.69400562256037));
#33676=CARTESIAN_POINT('',(-0.15564091233498,0.000130139906504897,-1.02900562256037));
#33677=CARTESIAN_POINT('',(-0.155295176870621,1.17227753446275E-5,-1.01519437743963));
#33678=CARTESIAN_POINT('',(-0.15555,-7.70311135908521E-15,-1.69400562256037));
#33679=CARTESIAN_POINT('Ctrl Pts',(-0.15564091233498,0.00013013990650489,
-1.02900562256037));
#33680=CARTESIAN_POINT('Ctrl Pts',(-0.155258831108901,-0.0425030626805927,
-1.02594662543473));
#33681=CARTESIAN_POINT('Ctrl Pts',(-0.115015154867651,-0.137419804614315,
-1.01918170063007));
#33682=CARTESIAN_POINT('Ctrl Pts',(0.0456441385565052,-0.178118983022976,
-1.00871084814638));
#33683=CARTESIAN_POINT('Ctrl Pts',(0.174423500194588,-0.0581910824574806,
-0.997593065109308));
#33684=CARTESIAN_POINT('Ctrl Pts',(0.143445970860419,0.11503483360103,-0.986475282072236));
#33685=CARTESIAN_POINT('Ctrl Pts',(-0.0189157028212204,0.182898758017883,
-0.975357499035165));
#33686=CARTESIAN_POINT('Ctrl Pts',(-0.138367090429786,0.100822903310039,
-0.966200945864541));
#33687=CARTESIAN_POINT('Ctrl Pts',(-0.155332819448999,0.0244770846789348,
-0.960750320372944));
#33688=CARTESIAN_POINT('Ctrl Pts',(-0.155297992403489,2.48232510734348E-5,
-0.95900562256037));
#33689=CARTESIAN_POINT('Ctrl Pts',(-0.155295176870621,1.1722775344624E-5,
-1.01519437743963));
#33690=CARTESIAN_POINT('Ctrl Pts',(-0.155277247152915,-0.026672930115448,
-1.01329048172623));
#33691=CARTESIAN_POINT('Ctrl Pts',(-0.136055195927886,-0.105323398094664,
-1.00768065833381));
#33692=CARTESIAN_POINT('Ctrl Pts',(-0.0110600915264488,-0.183541362009925,
-0.99836490726237));
#33693=CARTESIAN_POINT('Ctrl Pts',(0.148244063463316,-0.10878168430814,
-0.987247124225296));
#33694=CARTESIAN_POINT('Ctrl Pts',(0.171769434874196,0.0656126393009093,
-0.976129341188226));
#33695=CARTESIAN_POINT('Ctrl Pts',(0.0379688103673882,0.17991144108232,
-0.965011558151151));
#33696=CARTESIAN_POINT('Ctrl Pts',(-0.118384802577525,0.133087407394055,
-0.954699903568288));
#33697=CARTESIAN_POINT('Ctrl Pts',(-0.155199981190967,0.0403182355500233,
-0.948094176664447));
#33698=CARTESIAN_POINT('Ctrl Pts',(-0.155574065889681,-0.000140958060374001,
-0.94519437743963));
#33699=CARTESIAN_POINT('Origin',(0.,0.,-1.69400562256037));
#33700=CARTESIAN_POINT('',(-0.155715979727104,-0.000103239153171051,-1.09900562256037));
#33701=CARTESIAN_POINT('',(-0.15561713819096,0.000135214911208083,-1.08519437743963));
#33702=CARTESIAN_POINT('',(-0.15555,-7.70311135908521E-15,-1.69400562256037));
#33703=CARTESIAN_POINT('Ctrl Pts',(-0.155715979727104,-0.000103239153171026,
-1.09900562256037));
#33704=CARTESIAN_POINT('Ctrl Pts',(-0.155764022106253,-0.0063786663684298,
-1.09855478585457));
#33705=CARTESIAN_POINT('Ctrl Pts',(-0.15256950177487,-0.0641894789869248,
-1.09439802146974));
#33706=CARTESIAN_POINT('Ctrl Pts',(-0.0802215287029169,-0.165451702409712,
-1.08653532940589));
#33707=CARTESIAN_POINT('Ctrl Pts',(0.0955539257930597,-0.157096170428305,
-1.07541754636882));
#33708=CARTESIAN_POINT('Ctrl Pts',(0.183810220956364,-0.00485408793464279,
-1.06429976333174));
#33709=CARTESIAN_POINT('Ctrl Pts',(0.103712198059592,0.151833920687547,
-1.05318198029467));
#33710=CARTESIAN_POINT('Ctrl Pts',(-0.0713772583275903,0.169455145957098,
-1.0420641972576));
#33711=CARTESIAN_POINT('Ctrl Pts',(-0.150904081293975,0.0697258462719453,
-1.03400541134617));
#33712=CARTESIAN_POINT('Ctrl Pts',(-0.1557217166015,0.0091464024950112,
-1.02965255311376));
#33713=CARTESIAN_POINT('Ctrl Pts',(-0.15564091233498,0.00013013990650489,
-1.02900562256037));
#33714=CARTESIAN_POINT('Ctrl Pts',(-0.15561713819096,0.000135214911208083,
-1.08519437743963));
#33715=CARTESIAN_POINT('Ctrl Pts',(-0.155234629029245,-0.0417154247154185,
-1.08219271446705));
#33716=CARTESIAN_POINT('Ctrl Pts',(-0.116246810649056,-0.135864191994095,
-1.07548512381544));
#33717=CARTESIAN_POINT('Ctrl Pts',(0.0428888445928814,-0.17880241665738,
-1.06507160548481));
#33718=CARTESIAN_POINT('Ctrl Pts',(0.173504336038483,-0.060876946119833,
-1.05395382244773));
#33719=CARTESIAN_POINT('Ctrl Pts',(0.145204811647398,0.112806559505532,
-1.04283603941066));
#33720=CARTESIAN_POINT('Ctrl Pts',(-0.0160898036409584,0.183168980484762,
-1.03171825637359));
#33721=CARTESIAN_POINT('Ctrl Pts',(-0.13754985709603,0.102444722253558,
-1.02250436904991));
#33722=CARTESIAN_POINT('Ctrl Pts',(-0.155312147298262,0.0252686720728152,
-1.01699640940526));
#33723=CARTESIAN_POINT('Ctrl Pts',(-0.155295176870621,1.1722775344624E-5,
-1.01519437743963));
#33724=CARTESIAN_POINT('Origin',(0.,0.,-1.69400562256037));
#33725=CARTESIAN_POINT('',(-0.155322542976565,-6.74140301452986E-5,-1.16900562256037));
#33726=CARTESIAN_POINT('',(-0.155735118268745,-9.28043970148673E-5,-1.15519437743963));
#33727=CARTESIAN_POINT('',(-0.15555,-7.70311135908521E-15,-1.69400562256037));
#33728=CARTESIAN_POINT('Ctrl Pts',(-0.155322542976565,-6.74140301453116E-5,
-1.16900562256037));
#33729=CARTESIAN_POINT('Ctrl Pts',(-0.15540725279883,-0.021762817988561,
-1.16745701859538));
#33730=CARTESIAN_POINT('Ctrl Pts',(-0.141033818316528,-0.0952697082468468,
-1.16220248695136));
#33731=CARTESIAN_POINT('Ctrl Pts',(-0.0285426415962272,-0.181645470927358,
-1.15324202762832));
#33732=CARTESIAN_POINT('Ctrl Pts',(0.137174554457832,-0.122445502600127,
-1.14212424459125));
#33733=CARTESIAN_POINT('Ctrl Pts',(0.177251682996677,0.0489039913764663,
-1.13100646155418));
#33734=CARTESIAN_POINT('Ctrl Pts',(0.0549815489042986,0.175461644748333,
-1.11988867851711));
#33735=CARTESIAN_POINT('Ctrl Pts',(-0.110646694549052,0.142696374884672,
-1.10922173218584));
#33736=CARTESIAN_POINT('Ctrl Pts',(-0.155369108426059,0.0452060407225295,
-1.10226071353359));
#33737=CARTESIAN_POINT('Ctrl Pts',(-0.155715979727104,-0.000103239153171026,
-1.09900562256037));
#33738=CARTESIAN_POINT('Ctrl Pts',(-0.155735118268745,-9.28043970148612E-5,
-1.15519437743963));
#33739=CARTESIAN_POINT('Ctrl Pts',(-0.155773755432419,-0.00556840185665671,
-1.15480087488688));
#33740=CARTESIAN_POINT('Ctrl Pts',(-0.153026196109622,-0.0625728674990446,
-1.15070144465511));
#33741=CARTESIAN_POINT('Ctrl Pts',(-0.0827662568575337,-0.164193495360887,
-1.14289608674431));
#33742=CARTESIAN_POINT('Ctrl Pts',(0.0931172382976506,-0.158552632033813,
-1.13177830370724));
#33743=CARTESIAN_POINT('Ctrl Pts',(0.183713369824886,-0.00769122491000194,
-1.12066052067017));
#33744=CARTESIAN_POINT('Ctrl Pts',(0.106043890579969,0.150214681252184,
-1.10954273763309));
#33745=CARTESIAN_POINT('Ctrl Pts',(-0.0687526515134619,0.170536887807008,
-1.09842495459602));
#33746=CARTESIAN_POINT('Ctrl Pts',(-0.150386323062114,0.0713465315647904,
-1.09030883453153));
#33747=CARTESIAN_POINT('Ctrl Pts',(-0.155706884343325,0.00995441470151274,
-1.08589864214607));
#33748=CARTESIAN_POINT('Ctrl Pts',(-0.15561713819096,0.000135214911208083,
-1.08519437743963));
#33749=CARTESIAN_POINT('Origin',(0.,0.,-1.69400562256037));
#33750=CARTESIAN_POINT('',(-0.155469168273574,0.00013710264519145,-1.23900562256037));
#33751=CARTESIAN_POINT('',(-0.155333899255999,-7.87989482575052E-5,-1.22519437743963));
#33752=CARTESIAN_POINT('',(-0.15555,-7.70311135908521E-15,-1.69400562256037));
#33753=CARTESIAN_POINT('Ctrl Pts',(-0.155469168273574,0.000137102645191454,
-1.23900562256037));
#33754=CARTESIAN_POINT('Ctrl Pts',(-0.155155856663809,-0.0368497007893972,
-1.23635925133619));
#33755=CARTESIAN_POINT('Ctrl Pts',(-0.12342921310041,-0.126115115492115,
-1.23000695243298));
#33756=CARTESIAN_POINT('Ctrl Pts',(0.0256122765083437,-0.182081769516105,
-1.21994872585076));
#33757=CARTESIAN_POINT('Ctrl Pts',(0.166895497950393,-0.0771728725754398,
-1.20883094281368));
#33758=CARTESIAN_POINT('Ctrl Pts',(0.155316829566065,0.0984197233850115,
-1.19771315977661));
#33759=CARTESIAN_POINT('Ctrl Pts',(0.00148133352129465,0.183868336449635,
-1.18659537673954));
#33760=CARTESIAN_POINT('Ctrl Pts',(-0.132094093876729,0.112464811996422,
-1.17702619766746));
#33761=CARTESIAN_POINT('Ctrl Pts',(-0.155204535718084,0.030155942297909,
-1.1711629462744));
#33762=CARTESIAN_POINT('Ctrl Pts',(-0.155322542976565,-6.74140301453116E-5,
-1.16900562256037));
#33763=CARTESIAN_POINT('Ctrl Pts',(-0.155333899255999,-7.87989482575243E-5,
-1.22519437743963));
#33764=CARTESIAN_POINT('Ctrl Pts',(-0.155429657836139,-0.0209671487471519,
-1.22370310762769));
#33765=CARTESIAN_POINT('Ctrl Pts',(-0.141776642167995,-0.0936447578516373,
-1.21850591013673));
#33766=CARTESIAN_POINT('Ctrl Pts',(-0.0313435345808448,-0.181183167079792,
-1.20960278496674));
#33767=CARTESIAN_POINT('Ctrl Pts',(0.135267852386276,-0.124548646334775,
-1.19848500192967));
#33768=CARTESIAN_POINT('Ctrl Pts',(0.177985546579018,0.0461616984305375,
-1.1873672188926));
#33769=CARTESIAN_POINT('Ctrl Pts',(0.0576838223577768,0.174591906545624,
-1.17624943585553));
#33770=CARTESIAN_POINT('Ctrl Pts',(-0.109323369976581,0.144225213236364,
-1.1655251553712));
#33771=CARTESIAN_POINT('Ctrl Pts',(-0.155409878417394,0.0459996706834923,
-1.1585068025659));
#33772=CARTESIAN_POINT('Ctrl Pts',(-0.155735118268745,-9.28043970148612E-5,
-1.15519437743963));
#33773=CARTESIAN_POINT('Origin',(0.,0.,-1.69400562256037));
#33774=CARTESIAN_POINT('',(-0.155804675564127,-9.9298664568263E-6,-1.30900562256037));
#33775=CARTESIAN_POINT('',(-0.155447125224745,0.0001327912984651,-1.29519437743963));
#33776=CARTESIAN_POINT('',(-0.15555,-7.70311135908521E-15,-1.69400562256037));
#33777=CARTESIAN_POINT('Ctrl Pts',(-0.155804675564127,-9.92986645682631E-6,
-1.30900562256037));
#33778=CARTESIAN_POINT('Ctrl Pts',(-0.155805165222731,-0.000541004492398835,
-1.30896741175602));
#33779=CARTESIAN_POINT('Ctrl Pts',(-0.155562120987005,-0.0525786248856173,
-1.30522327327266));
#33780=CARTESIAN_POINT('Ctrl Pts',(-0.0980726456853608,-0.155536219688844,
-1.29777320711026));
#33781=CARTESIAN_POINT('Ctrl Pts',(0.0775453683472552,-0.166722749977294,
-1.28665542407319));
#33782=CARTESIAN_POINT('Ctrl Pts',(0.18213850936899,-0.025205612527195,
-1.27553764103612));
#33783=CARTESIAN_POINT('Ctrl Pts',(0.119908476028974,0.139397693201698,
-1.26441985799905));
#33784=CARTESIAN_POINT('Ctrl Pts',(-0.0521473853035587,0.176324728004856,
-1.25330207496197));
#33785=CARTESIAN_POINT('Ctrl Pts',(-0.146855130761894,0.0814052574977526,
-1.24483066314908));
#33786=CARTESIAN_POINT('Ctrl Pts',(-0.155594612253418,0.0149459117665484,
-1.24006517901521));
#33787=CARTESIAN_POINT('Ctrl Pts',(-0.155469168273574,0.000137102645191454,
-1.23900562256037));
#33788=CARTESIAN_POINT('Ctrl Pts',(-0.155447125224745,0.000132791298465095,
-1.29519437743963));
#33789=CARTESIAN_POINT('Ctrl Pts',(-0.155153338736769,-0.0360656743444678,
-1.2926053403685));
#33790=CARTESIAN_POINT('Ctrl Pts',(-0.124516957166434,-0.124526645405497,
-1.28631037561835));
#33791=CARTESIAN_POINT('Ctrl Pts',(0.0227981919227724,-0.182455473034852,
-1.27630948318918));
#33792=CARTESIAN_POINT('Ctrl Pts',(0.165684184825268,-0.0797402538976839,
-1.26519170015211));
#33793=CARTESIAN_POINT('Ctrl Pts',(0.1568177463056,0.0960101642333705,-1.25407391711503));
#33794=CARTESIAN_POINT('Ctrl Pts',(0.00431976977229057,0.183823547954278,
-1.24295613407796));
#33795=CARTESIAN_POINT('Ctrl Pts',(-0.13114891460843,0.114075301211355,
-1.23332962085283));
#33796=CARTESIAN_POINT('Ctrl Pts',(-0.155191689917924,0.0309421121184549,
-1.22740903530672));
#33797=CARTESIAN_POINT('Ctrl Pts',(-0.155333899255999,-7.87989482575243E-5,
-1.22519437743963));
#33798=CARTESIAN_POINT('Origin',(0.,0.,-1.69400562256037));
#33799=CARTESIAN_POINT('',(-0.155440006104157,-0.000131091492392236,-1.37900562256037));
#33800=CARTESIAN_POINT('',(-0.155805262673826,4.97304114227787E-6,-1.36519437743963));
#33801=CARTESIAN_POINT('',(-0.15555,-7.70311135908521E-15,-1.69400562256037));
#33802=CARTESIAN_POINT('Ctrl Pts',(-0.155440006104157,-0.000131091492392219,
-1.37900562256037));
#33803=CARTESIAN_POINT('Ctrl Pts',(-0.155566842076363,-0.0160155424259783,
-1.37786964449684));
#33804=CARTESIAN_POINT('Ctrl Pts',(-0.14602074484413,-0.0835713921170919,
-1.37302773875428));
#33805=CARTESIAN_POINT('Ctrl Pts',(-0.048508054493723,-0.177360442508133,
-1.3644799053327));
#33806=CARTESIAN_POINT('Ctrl Pts',(0.12275151636726,-0.136900786130964,
-1.35336212229563));
#33807=CARTESIAN_POINT('Ctrl Pts',(0.181581280715027,0.0289481974204555,
-1.34224433925855));
#33808=CARTESIAN_POINT('Ctrl Pts',(0.0740982434113141,0.1682831233296,-1.33112655622148));
#33809=CARTESIAN_POINT('Ctrl Pts',(-0.100649733124876,0.15353607539823,
-1.32004698398875));
#33810=CARTESIAN_POINT('Ctrl Pts',(-0.155757675006093,0.0509660022204176,
-1.31267333943505));
#33811=CARTESIAN_POINT('Ctrl Pts',(-0.155804675564127,-9.92986645682631E-6,
-1.30900562256037));
#33812=CARTESIAN_POINT('Ctrl Pts',(-0.155805262673826,4.97304114227722E-6,
-1.36519437743963));
#33813=CARTESIAN_POINT('Ctrl Pts',(-0.155781279836539,-0.0512357195429724,
-1.36150757310931));
#33814=CARTESIAN_POINT('Ctrl Pts',(-0.100160425534363,-0.154027506270637,
-1.35411484109998));
#33815=CARTESIAN_POINT('Ctrl Pts',(0.0749622096468331,-0.167900042901071,
-1.34301618141161));
#33816=CARTESIAN_POINT('Ctrl Pts',(0.181727664822887,-0.0280145148561602,
-1.33189839837454));
#33817=CARTESIAN_POINT('Ctrl Pts',(0.122046243641521,0.137529893387063,
-1.32078061533747));
#33818=CARTESIAN_POINT('Ctrl Pts',(-0.0494190162937222,0.17710877458793,
-1.3096628323004));
#33819=CARTESIAN_POINT('Ctrl Pts',(-0.146231685180962,0.0830303065190035,
-1.30113408633445));
#33820=CARTESIAN_POINT('Ctrl Pts',(-0.155573862447942,0.01574852996355,
-1.29631126804753));
#33821=CARTESIAN_POINT('Ctrl Pts',(-0.155447125224745,0.000132791298465095,
-1.29519437743963));
#33822=CARTESIAN_POINT('Origin',(0.,0.,-1.69400562256037));
#33823=CARTESIAN_POINT('',(-0.155338051549543,8.26344013249621E-5,-1.44900562256037));
#33824=CARTESIAN_POINT('',(-0.15546172451378,-0.000135797342094887,-1.43519437743963));
#33825=CARTESIAN_POINT('',(-0.15555,-7.70311135908521E-15,-1.69400562256037));
#33826=CARTESIAN_POINT('Ctrl Pts',(-0.155338051549543,8.26344013249731E-5,
-1.44900562256037));
#33827=CARTESIAN_POINT('Ctrl Pts',(-0.155187751699248,-0.0312036093690435,
-1.44677187723765));
#33828=CARTESIAN_POINT('Ctrl Pts',(-0.130830226648687,-0.114611274732386,
-1.4408322042359));
#33829=CARTESIAN_POINT('Ctrl Pts',(0.00526457092671344,-0.183798721027812,
-1.43118660355513));
#33830=CARTESIAN_POINT('Ctrl Pts',(0.157309138173746,-0.095202988083288,
-1.42006882051806));
#33831=CARTESIAN_POINT('Ctrl Pts',(0.165272159879762,0.0805908485969487,
-1.40895103748099));
#33832=CARTESIAN_POINT('Ctrl Pts',(0.021860095314849,0.182570218824516,
-1.39783325444391));
#33833=CARTESIAN_POINT('Ctrl Pts',(-0.124874771184232,0.123997024126219,
-1.38785144947038));
#33834=CARTESIAN_POINT('Ctrl Pts',(-0.155153062131851,0.0358046715997731,
-1.38157557217586));
#33835=CARTESIAN_POINT('Ctrl Pts',(-0.155440006104157,-0.000131091492392219,
-1.37900562256037));
#33836=CARTESIAN_POINT('Ctrl Pts',(-0.15546172451378,-0.000135797342094889,
-1.43519437743963));
#33837=CARTESIAN_POINT('Ctrl Pts',(-0.155587764885392,-0.015213215124397,
-1.43411573352915));
#33838=CARTESIAN_POINT('Ctrl Pts',(-0.146649276514878,-0.0819462556503598,
-1.42933116193965));
#33839=CARTESIAN_POINT('Ctrl Pts',(-0.0512404048426255,-0.176590393721669,
-1.42084066267112));
#33840=CARTESIAN_POINT('Ctrl Pts',(0.120623364083146,-0.138779552138408,
-1.40972287963405));
#33841=CARTESIAN_POINT('Ctrl Pts',(0.1820065472977,0.0261414484512927,-1.39860509659698));
#33842=CARTESIAN_POINT('Ctrl Pts',(0.0766874125244866,0.167119108331645,
-1.3874873135599));
#33843=CARTESIAN_POINT('Ctrl Pts',(-0.0988707767058873,0.15503008489993,
-1.37636953052283));
#33844=CARTESIAN_POINT('Ctrl Pts',(-0.155684373061444,0.0520429010369321,
-1.36893855181607));
#33845=CARTESIAN_POINT('Ctrl Pts',(-0.155805387072118,0.000270757049356713,
-1.36521350078834));
#33846=CARTESIAN_POINT('Ctrl Pts',(-0.155805262673826,4.97304114227722E-6,
-1.36519437743963));
#33847=CARTESIAN_POINT('Origin',(0.,0.,-1.69400562256037));
#33848=CARTESIAN_POINT('',(-0.155739242772632,9.98782012467415E-5,-1.51900562256037));
#33849=CARTESIAN_POINT('',(-0.155325699155423,7.24743171157949E-5,-1.50519437743963));
#33850=CARTESIAN_POINT('',(-0.15555,-7.70311135908521E-15,-1.69400562256037));
#33851=CARTESIAN_POINT('Ctrl Pts',(-0.155739242772632,9.98782012467418E-5,
-1.51900562256037));
#33852=CARTESIAN_POINT('Ctrl Pts',(-0.155421972044204,-0.0462505870687982,
-1.51567410997846));
#33853=CARTESIAN_POINT('Ctrl Pts',(-0.108881181232048,-0.144750054452956,
-1.50863666971753));
#33854=CARTESIAN_POINT('Ctrl Pts',(0.0585821121664253,-0.174283509875506,
-1.49789330177756));
#33855=CARTESIAN_POINT('Ctrl Pts',(0.178219584548083,-0.0452513232337437,
-1.4867755187405));
#33856=CARTESIAN_POINT('Ctrl Pts',(0.134626373349144,0.125244912864161,
-1.47565773570342));
#33857=CARTESIAN_POINT('Ctrl Pts',(-0.0322746164076941,0.18101828554357,
-1.46453995266635));
#33858=CARTESIAN_POINT('Ctrl Pts',(-0.14202024933615,0.0931040090647467,
-1.455655914952));
#33859=CARTESIAN_POINT('Ctrl Pts',(-0.155437108852768,0.0207022885781798,
-1.45047780491667));
#33860=CARTESIAN_POINT('Ctrl Pts',(-0.155338051549543,8.26344013249731E-5,
-1.44900562256037));
#33861=CARTESIAN_POINT('Ctrl Pts',(-0.155325699155423,7.24743171158018E-5,
-1.50519437743963));
#33862=CARTESIAN_POINT('Ctrl Pts',(-0.155199852209928,-0.0304170665609612,
-1.50301796626996));
#33863=CARTESIAN_POINT('Ctrl Pts',(-0.131782164237154,-0.113003219889635,
-1.49713562742127));
#33864=CARTESIAN_POINT('Ctrl Pts',(0.00242683334840427,-0.183856950102903,
-1.48754736089355));
#33865=CARTESIAN_POINT('Ctrl Pts',(0.155820388725155,-0.0976208199140973,
-1.47642957785648));
#33866=CARTESIAN_POINT('Ctrl Pts',(0.166496760685316,0.078030035232174,
-1.46531179481941));
#33867=CARTESIAN_POINT('Ctrl Pts',(0.0246759993484255,0.182210807009283,
-1.45419401178234));
#33868=CARTESIAN_POINT('Ctrl Pts',(-0.123793478086846,0.125586772778578,
-1.44415487265574));
#33869=CARTESIAN_POINT('Ctrl Pts',(-0.155154724382133,0.036588699617641,
-1.43782166120817));
#33870=CARTESIAN_POINT('Ctrl Pts',(-0.15546172451378,-0.000135797342094889,
-1.43519437743963));
#33871=CARTESIAN_POINT('Origin',(2.59090492670967E-17,0.,-0.02));
#33872=CARTESIAN_POINT('',(0.00853826423429785,0.19521336543348,-0.02));
#33873=CARTESIAN_POINT('Ctrl Pts',(0.133821766704343,-0.0798002879704671,
-0.0200000000000001));
#33874=CARTESIAN_POINT('Ctrl Pts',(0.136065138599399,-0.0769506293259119,
-0.0200000000000001));
#33875=CARTESIAN_POINT('Ctrl Pts',(0.138197889310311,-0.0740223739865894,
-0.0199999999999998));
#33876=CARTESIAN_POINT('Ctrl Pts',(0.140214087153587,-0.0710196745109591,
-0.0199999999999999));
#33877=CARTESIAN_POINT('Ctrl Pts',(0.145120054681607,-0.0637132754028678,
-0.0199999999999999));
#33878=CARTESIAN_POINT('Ctrl Pts',(0.149337231868511,-0.055967386575868,
-0.0200000000000001));
#33879=CARTESIAN_POINT('Ctrl Pts',(0.152881379977793,-0.0478854058222795,
-0.0199999999999998));
#33880=CARTESIAN_POINT('Ctrl Pts',(0.154570678326317,-0.0440331749563981,
-0.0199999999999997));
#33881=CARTESIAN_POINT('Ctrl Pts',(0.156106559607416,-0.0401039093554644,
-0.0199999999999995));
#33882=CARTESIAN_POINT('Ctrl Pts',(0.157485311894354,-0.036122580876755,
-0.0199999999999995));
#33883=CARTESIAN_POINT('Ctrl Pts',(0.160039385365418,-0.0287473579716647,
-0.0199999999999996));
#33884=CARTESIAN_POINT('Ctrl Pts',(0.162060174255282,-0.0211826817802034,
-0.0199999999999997));
#33885=CARTESIAN_POINT('Ctrl Pts',(0.163555878906819,-0.0134954408667204,
-0.0199999999999998));
#33886=CARTESIAN_POINT('Ctrl Pts',(0.164335346674248,-0.00948933143437693,
-0.0199999999999998));
#33887=CARTESIAN_POINT('Ctrl Pts',(0.164972230950227,-0.00544823120734308,
-0.0200000000000002));
#33888=CARTESIAN_POINT('Ctrl Pts',(0.165465981759546,-0.00138582933311573,
-0.0200000000000002));
#33889=CARTESIAN_POINT('Ctrl Pts',(0.166873155854188,0.0101918867365069,
-0.0200000000000002));
#33890=CARTESIAN_POINT('Ctrl Pts',(0.167113372873192,0.0218697098856196,
-0.0199999999999994));
#33891=CARTESIAN_POINT('Ctrl Pts',(0.166212385384324,0.0334410544872706,
-0.0199999999999993));
#33892=CARTESIAN_POINT('Ctrl Pts',(0.165524991089037,0.0422692306453721,
-0.0199999999999993));
#33893=CARTESIAN_POINT('Ctrl Pts',(0.164172506243096,0.051036511458747,
-0.0199999999999997));
#33894=CARTESIAN_POINT('Ctrl Pts',(0.162147313208725,0.0596568175050613,
-0.0199999999999997));
#33895=CARTESIAN_POINT('Ctrl Pts',(0.161339114894091,0.0630969423228057,
-0.0199999999999997));
#33896=CARTESIAN_POINT('Ctrl Pts',(0.160423339052115,0.066513402035509,
-0.0199999999999997));
#33897=CARTESIAN_POINT('Ctrl Pts',(0.159403754602336,0.069887176638175,
-0.0199999999999997));
#33898=CARTESIAN_POINT('Ctrl Pts',(0.157419300482608,0.0764536762652955,
-0.0199999999999997));
#33899=CARTESIAN_POINT('Ctrl Pts',(0.155039126041078,0.0828715355915416,
-0.0199999999999998));
#33900=CARTESIAN_POINT('Ctrl Pts',(0.152264969414956,0.0891018848696017,
-0.0199999999999998));
#33901=CARTESIAN_POINT('Ctrl Pts',(0.149133055506545,0.0961357045805976,
-0.0199999999999998));
#33902=CARTESIAN_POINT('Ctrl Pts',(0.145499258844698,0.10293079067009,-0.0199999999999997));
#33903=CARTESIAN_POINT('Ctrl Pts',(0.141411895748059,0.109465395998025,
-0.0199999999999996));
#33904=CARTESIAN_POINT('Ctrl Pts',(0.138924049814933,0.113442799254188,
-0.0199999999999996));
#33905=CARTESIAN_POINT('Ctrl Pts',(0.136267962558613,0.117323661573993,
-0.0199999999999997));
#33906=CARTESIAN_POINT('Ctrl Pts',(0.133452844321485,0.121102461008537,
-0.0199999999999997));
#33907=CARTESIAN_POINT('Ctrl Pts',(0.131317154149409,0.123969248168011,
-0.0199999999999997));
#33908=CARTESIAN_POINT('Ctrl Pts',(0.129090064208231,0.126776619840538,
-0.0199999999999998));
#33909=CARTESIAN_POINT('Ctrl Pts',(0.126784735751445,0.129512001730073,
-0.0199999999999999));
#33910=CARTESIAN_POINT('Ctrl Pts',(0.119384017280744,0.138293306283324,
-0.0200000000000001));
#33911=CARTESIAN_POINT('Ctrl Pts',(0.111159161660068,0.146362743803953,
-0.0200000000000003));
#33912=CARTESIAN_POINT('Ctrl Pts',(0.102260233844386,0.153651749300115,
-0.0200000000000002));
#33913=CARTESIAN_POINT('Ctrl Pts',(0.0967966677903543,0.158126891004974,
-0.0200000000000001));
#33914=CARTESIAN_POINT('Ctrl Pts',(0.0910781750600193,0.162307627165175,
-0.0199999999999998));
#33915=CARTESIAN_POINT('Ctrl Pts',(0.0851331862206853,0.166174253363221,
-0.0199999999999996));
#33916=CARTESIAN_POINT('Ctrl Pts',(0.0806708967451739,0.169076530534058,
-0.0199999999999995));
#33917=CARTESIAN_POINT('Ctrl Pts',(0.0760753987718405,0.171804249124038,
-0.02));
#33918=CARTESIAN_POINT('Ctrl Pts',(0.0713880909719757,0.174332475493028,
-0.02));
#33919=CARTESIAN_POINT('Ctrl Pts',(0.0601005419700875,0.18042072065343,
-0.02));
#33920=CARTESIAN_POINT('Ctrl Pts',(0.0482596588054404,0.185373180166949,
-0.0199999999999998));
#33921=CARTESIAN_POINT('Ctrl Pts',(0.0360387384670489,0.189087621526514,
-0.0199999999999995));
#33922=CARTESIAN_POINT('Ctrl Pts',(0.0270584772457173,0.191817093021016,
-0.0199999999999992));
#33923=CARTESIAN_POINT('Ctrl Pts',(0.0178719156836204,0.19387762520946,
-0.02));
#33924=CARTESIAN_POINT('Ctrl Pts',(0.00853826423429785,0.19521336543348,
-0.02));
#33925=CARTESIAN_POINT('',(-0.1954,-2.39295984553393E-17,-0.02));
#33926=CARTESIAN_POINT('Origin',(0.,0.,-0.02));
#33927=CARTESIAN_POINT('',(-0.149577187126323,0.126230651412956,-0.0200000000000003));
#33928=CARTESIAN_POINT('Origin',(0.,0.,-0.02));
#33929=CARTESIAN_POINT('Ctrl Pts',(-0.149578925757925,0.126231591330479,
-0.0200000000000002));
#33930=CARTESIAN_POINT('Ctrl Pts',(-0.152148426341253,0.122532430052756,
-0.0200000000000002));
#33931=CARTESIAN_POINT('Ctrl Pts',(-0.154577059731215,0.118743491976515,
-0.0200000000000004));
#33932=CARTESIAN_POINT('Ctrl Pts',(-0.156856766744289,0.114867806158737,
-0.0200000000000003));
#33933=CARTESIAN_POINT('Ctrl Pts',(-0.161319559432387,0.107280698591954,
-0.0200000000000001));
#33934=CARTESIAN_POINT('Ctrl Pts',(-0.165212332552683,0.099361225354574,
-0.0200000000000002));
#33935=CARTESIAN_POINT('Ctrl Pts',(-0.168532013693597,0.0911785794352264,
-0.0200000000000004));
#33936=CARTESIAN_POINT('Ctrl Pts',(-0.17021136272293,0.0870391702875616,
-0.0200000000000005));
#33937=CARTESIAN_POINT('Ctrl Pts',(-0.171744680598151,0.0828297970998818,
-0.0200000000000001));
#33938=CARTESIAN_POINT('Ctrl Pts',(-0.173127719604902,0.0785680462167742,
-0.02));
#33939=CARTESIAN_POINT('Ctrl Pts',(-0.176934316037692,0.0668382499999685,
-0.02));
#33940=CARTESIAN_POINT('Ctrl Pts',(-0.179597768596154,0.05474203377193,
-0.02));
#33941=CARTESIAN_POINT('Ctrl Pts',(-0.18110253115427,0.042471584803998,
-0.0199999999999998));
#33942=CARTESIAN_POINT('Ctrl Pts',(-0.181600194320072,0.0384134359311063,
-0.0199999999999998));
#33943=CARTESIAN_POINT('Ctrl Pts',(-0.181970877474762,0.0343338115398897,
-0.0200000000000001));
#33944=CARTESIAN_POINT('Ctrl Pts',(-0.182212486373446,0.0302478964060663,
-0.0200000000000001));
#33945=CARTESIAN_POINT('Ctrl Pts',(-0.182939758490654,0.0179487958088136,
-0.0199999999999999));
#33946=CARTESIAN_POINT('Ctrl Pts',(-0.182499636986404,0.00564566013123739,
-0.0199999999999998));
#33947=CARTESIAN_POINT('Ctrl Pts',(-0.180874130922987,-0.0064689356643982,
-0.0199999999999997));
#33948=CARTESIAN_POINT('Ctrl Pts',(-0.179782006632617,-0.0146083358390246,
-0.0199999999999996));
#33949=CARTESIAN_POINT('Ctrl Pts',(-0.178153737391779,-0.0226626229005816,
-0.0200000000000001));
#33950=CARTESIAN_POINT('Ctrl Pts',(-0.175971558313481,-0.0305673708748629,
-0.0200000000000001));
#33951=CARTESIAN_POINT('Ctrl Pts',(-0.17467131893799,-0.0352773713838545,
-0.0200000000000001));
#33952=CARTESIAN_POINT('Ctrl Pts',(-0.173172167501843,-0.0399385102644172,
-0.02));
#33953=CARTESIAN_POINT('Ctrl Pts',(-0.171480129271394,-0.0445086904000026,
-0.02));
#33954=CARTESIAN_POINT('Ctrl Pts',(-0.169172916523709,-0.050740451407697,
-0.02));
#33955=CARTESIAN_POINT('Ctrl Pts',(-0.1665054327452,-0.056812742784086,
-0.0200000000000005));
#33956=CARTESIAN_POINT('Ctrl Pts',(-0.163471173762726,-0.0626921515535454,
-0.0200000000000004));
#33957=CARTESIAN_POINT('Ctrl Pts',(-0.158053708478377,-0.0731894403759654,
-0.0200000000000002));
#33958=CARTESIAN_POINT('Ctrl Pts',(-0.15146825397439,-0.0830745741085914,
-0.0200000000000001));
#33959=CARTESIAN_POINT('Ctrl Pts',(-0.143867977301061,-0.0922205054292428,
-0.0200000000000001));
#33960=CARTESIAN_POINT('Ctrl Pts',(-0.141491856997698,-0.0950798530606812,
-0.02));
#33961=CARTESIAN_POINT('Ctrl Pts',(-0.13901541851784,-0.097867176501796,
-0.0200000000000004));
#33962=CARTESIAN_POINT('Ctrl Pts',(-0.136455144305558,-0.100566063717065,
-0.0200000000000004));
#33963=CARTESIAN_POINT('Ctrl Pts',(-0.129616213094456,-0.107775254015195,
-0.0200000000000004));
#33964=CARTESIAN_POINT('Ctrl Pts',(-0.122162587580282,-0.114377608974371,
-0.0200000000000003));
#33965=CARTESIAN_POINT('Ctrl Pts',(-0.114191093890929,-0.120301882844334,
-0.0200000000000004));
#33966=CARTESIAN_POINT('Ctrl Pts',(-0.109769836460304,-0.123587683584993,
-0.0200000000000004));
#33967=CARTESIAN_POINT('Ctrl Pts',(-0.105188998350819,-0.126664460370265,
-0.0200000000000003));
#33968=CARTESIAN_POINT('Ctrl Pts',(-0.10046396900964,-0.129516366658698,
-0.0200000000000003));
#33969=CARTESIAN_POINT('Ctrl Pts',(-0.0975150341637712,-0.131296267951124,
-0.0200000000000003));
#33970=CARTESIAN_POINT('Ctrl Pts',(-0.0945099247899165,-0.132988524390106,
-0.0200000000000002));
#33971=CARTESIAN_POINT('Ctrl Pts',(-0.0914523710575882,-0.134588691868093,
-0.0200000000000002));
#33972=CARTESIAN_POINT('Ctrl Pts',(-0.0882670061071807,-0.13625574921046,
-0.0200000000000002));
#33973=CARTESIAN_POINT('Ctrl Pts',(-0.0850316946920376,-0.137819083369016,
-0.0199999999999997));
#33974=CARTESIAN_POINT('Ctrl Pts',(-0.0817560776251171,-0.139272781926057,
-0.0199999999999997));
#33975=CARTESIAN_POINT('Ctrl Pts',(-0.0719395593097613,-0.143629291926666,
-0.0199999999999999));
#33976=CARTESIAN_POINT('Ctrl Pts',(-0.0617469188109472,-0.147012280054498,
-0.02));
#33977=CARTESIAN_POINT('Ctrl Pts',(-0.0512986076831915,-0.149302477071082,
-0.02));
#33978=CARTESIAN_POINT('Ctrl Pts',(-0.0449384648191926,-0.150696576082307,
-0.02));
#33979=CARTESIAN_POINT('Ctrl Pts',(-0.0384834618551675,-0.151684836018586,
-0.02));
#33980=CARTESIAN_POINT('Ctrl Pts',(-0.0319621170202007,-0.152230829911641,
-0.02));
#33981=CARTESIAN_POINT('Ctrl Pts',(-0.0685825729128752,0.139614588036674,
-1.58760740822721));
#33982=CARTESIAN_POINT('Ctrl Pts',(-0.115024428893785,0.116801055304812,
-1.58390148054818));
#33983=CARTESIAN_POINT('Ctrl Pts',(-0.182548960740187,0.0215828567384845,
-1.57648962519013));
#33984=CARTESIAN_POINT('Ctrl Pts',(-0.116961678516305,-0.14203802638652,
-1.56537184215306));
#33985=CARTESIAN_POINT('Ctrl Pts',(0.0559048769350007,-0.175112865030439,
-1.55425405911599));
#33986=CARTESIAN_POINT('Ctrl Pts',(0.177489043046939,-0.0480257256248533,
-1.54313627607892));
#33987=CARTESIAN_POINT('Ctrl Pts',(0.136549507894468,0.123166484814191,
-1.53201849304185));
#33988=CARTESIAN_POINT('Ctrl Pts',(-0.0294791068043894,0.181487141263986,
-1.52090071000477));
#33989=CARTESIAN_POINT('Ctrl Pts',(-0.168496105669099,0.0736136087933882,
-1.5097829269677));
#33990=CARTESIAN_POINT('Ctrl Pts',(-0.153191130802483,-0.101700660683814,
-1.49866514393063));
#33991=CARTESIAN_POINT('Ctrl Pts',(0.00242683334840427,-0.183856950102903,
-1.48754736089355));
#33992=CARTESIAN_POINT('Ctrl Pts',(0.155820388725155,-0.0976208199140973,
-1.47642957785648));
#33993=CARTESIAN_POINT('Ctrl Pts',(0.166496760685316,0.078030035232174,
-1.46531179481941));
#33994=CARTESIAN_POINT('Ctrl Pts',(0.0246759993484255,0.182210807009283,
-1.45419401178234));
#33995=CARTESIAN_POINT('Ctrl Pts',(-0.139745612598391,0.119502867680789,
-1.44307622874526));
#33996=CARTESIAN_POINT('Ctrl Pts',(-0.176172414317729,-0.0526597555425937,
-1.43195844570819));
#33997=CARTESIAN_POINT('Ctrl Pts',(-0.0512404048426255,-0.176590393721669,
-1.42084066267112));
#33998=CARTESIAN_POINT('Ctrl Pts',(0.120623364083146,-0.138779552138408,
-1.40972287963405));
#33999=CARTESIAN_POINT('Ctrl Pts',(0.1820065472977,0.0261414484512927,-1.39860509659698));
#34000=CARTESIAN_POINT('Ctrl Pts',(0.0766874125244866,0.167119108331645,
-1.3874873135599));
#34001=CARTESIAN_POINT('Ctrl Pts',(-0.0988707767058873,0.15503008489993,
-1.37636953052283));
#34002=CARTESIAN_POINT('Ctrl Pts',(-0.183871859707572,0.000946859665196946,
-1.36525174748576));
#34003=CARTESIAN_POINT('Ctrl Pts',(-0.100462167484613,-0.154003603442465,
-1.35413396444869));
#34004=CARTESIAN_POINT('Ctrl Pts',(0.0749622096468331,-0.167900042901071,
-1.34301618141161));
#34005=CARTESIAN_POINT('Ctrl Pts',(0.181727664822887,-0.0280145148561602,
-1.33189839837454));
#34006=CARTESIAN_POINT('Ctrl Pts',(0.122046243641521,0.137529893387063,
-1.32078061533747));
#34007=CARTESIAN_POINT('Ctrl Pts',(-0.0494190162937222,0.17710877458793,
-1.3096628323004));
#34008=CARTESIAN_POINT('Ctrl Pts',(-0.175620717250213,0.054471284782664,
-1.29854504926333));
#34009=CARTESIAN_POINT('Ctrl Pts',(-0.140968979581843,-0.118057206406529,
-1.28742726622625));
#34010=CARTESIAN_POINT('Ctrl Pts',(0.0227981919227724,-0.182455473034852,
-1.27630948318918));
#34011=CARTESIAN_POINT('Ctrl Pts',(0.165684184825268,-0.0797402538976839,
-1.26519170015211));
#34012=CARTESIAN_POINT('Ctrl Pts',(0.1568177463056,0.0960101642333705,-1.25407391711503));
#34013=CARTESIAN_POINT('Ctrl Pts',(0.00431976977229057,0.183823547954278,
-1.24295613407796));
#34014=CARTESIAN_POINT('Ctrl Pts',(-0.152134743511917,0.103270407230458,
-1.23183835104089));
#34015=CARTESIAN_POINT('Ctrl Pts',(-0.169246945666504,-0.0718695246646475,
-1.22072056800382));
#34016=CARTESIAN_POINT('Ctrl Pts',(-0.0313435345808448,-0.181183167079792,
-1.20960278496674));
#34017=CARTESIAN_POINT('Ctrl Pts',(0.135267852386276,-0.124548646334775,
-1.19848500192967));
#34018=CARTESIAN_POINT('Ctrl Pts',(0.177985546579018,0.0461616984305375,
-1.1873672188926));
#34019=CARTESIAN_POINT('Ctrl Pts',(0.0576838223577768,0.174591906545624,
-1.17624943585553));
#34020=CARTESIAN_POINT('Ctrl Pts',(-0.115451310830705,0.14311097798737,
-1.16513165281845));
#34021=CARTESIAN_POINT('Ctrl Pts',(-0.182842995135233,-0.0194472703227996,
-1.15401386978138));
#34022=CARTESIAN_POINT('Ctrl Pts',(-0.0827662568575337,-0.164193495360887,
-1.14289608674431));
#34023=CARTESIAN_POINT('Ctrl Pts',(0.0931172382976506,-0.158552632033813,
-1.13177830370724));
#34024=CARTESIAN_POINT('Ctrl Pts',(0.183713369824886,-0.00769122491000194,
-1.12066052067017));
#34025=CARTESIAN_POINT('Ctrl Pts',(0.106043890579969,0.150214681252184,
-1.10954273763309));
#34026=CARTESIAN_POINT('Ctrl Pts',(-0.0687526515134619,0.170536887807008,
-1.09842495459602));
#34027=CARTESIAN_POINT('Ctrl Pts',(-0.180577691259814,0.0346620053128379,
-1.08730717155895));
#34028=CARTESIAN_POINT('Ctrl Pts',(-0.127009131505917,-0.132960286202853,
-1.07618938852188));
#34029=CARTESIAN_POINT('Ctrl Pts',(0.0428888445928814,-0.17880241665738,
-1.06507160548481));
#34030=CARTESIAN_POINT('Ctrl Pts',(0.173504336038483,-0.060876946119833,
-1.05395382244773));
#34031=CARTESIAN_POINT('Ctrl Pts',(0.145204811647398,0.112806559505532,
-1.04283603941066));
#34032=CARTESIAN_POINT('Ctrl Pts',(-0.0160898036409584,0.183168980484762,
-1.03171825637359));
#34033=CARTESIAN_POINT('Ctrl Pts',(-0.162647545726072,0.0857644044013417,
-1.02060047333651));
#34034=CARTESIAN_POINT('Ctrl Pts',(-0.160234156051553,-0.0901929732710832,
-1.00948269029944));
#34035=CARTESIAN_POINT('Ctrl Pts',(-0.0110600915264488,-0.183541362009925,
-0.99836490726237));
#34036=CARTESIAN_POINT('Ctrl Pts',(0.148244063463316,-0.10878168430814,
-0.987247124225296));
#34037=CARTESIAN_POINT('Ctrl Pts',(0.171769434874196,0.0656126393009093,
-0.976129341188226));
#34038=CARTESIAN_POINT('Ctrl Pts',(0.0379688103673882,0.17991144108232,
-0.965011558151151));
#34039=CARTESIAN_POINT('Ctrl Pts',(-0.130607971546202,0.129426871095682,
-0.953893775114081));
#34040=CARTESIAN_POINT('Ctrl Pts',(-0.179559109855943,-0.0396015562923112,
-0.942775992077008));
#34041=CARTESIAN_POINT('Ctrl Pts',(-0.0640495814302482,-0.172358371748057,
-0.931658209039936));
#34042=CARTESIAN_POINT('Ctrl Pts',(0.110123842548254,-0.147249775875683,
-0.920540426002863));
#34043=CARTESIAN_POINT('Ctrl Pts',(0.183433319364821,0.0127269218523267,
-0.909422642965792));
#34044=CARTESIAN_POINT('Ctrl Pts',(0.0887336874904625,0.161046856216992,
-0.898304859928718));
#34045=CARTESIAN_POINT('Ctrl Pts',(-0.0872383533320315,0.16186175243382,
-0.887187076891646));
#34046=CARTESIAN_POINT('Ctrl Pts',(-0.183307582398564,0.0144252358117838,
-0.876069293854574));
#34047=CARTESIAN_POINT('Ctrl Pts',(-0.111482866996807,-0.146223553366767,
-0.864951510817501));
#34048=CARTESIAN_POINT('Ctrl Pts',(0.0624505448146294,-0.172944172048056,
-0.853833727780429));
#34049=CARTESIAN_POINT('Ctrl Pts',(0.179184640777123,-0.0412628368220751,
-0.842715944743356));
#34050=CARTESIAN_POINT('Ctrl Pts',(0.131801051401358,0.128211700099984,
-0.831598161706284));
#34051=CARTESIAN_POINT('Ctrl Pts',(-0.0363009398827759,0.180255371505702,
-0.820480378669211));
#34052=CARTESIAN_POINT('Ctrl Pts',(-0.171154399354551,0.0672006605221613,
-0.80936259563214));
#34053=CARTESIAN_POINT('Ctrl Pts',(-0.149245182428924,-0.107404062841165,
-0.798244812595067));
#34054=CARTESIAN_POINT('Ctrl Pts',(0.00935975675220263,-0.183635922810792,
-0.787127029557995));
#34055=CARTESIAN_POINT('Ctrl Pts',(0.159391965553992,-0.0916731067972864,
-0.776009246520922));
#34056=CARTESIAN_POINT('Ctrl Pts',(0.163434873404623,0.0842543728731427,
-0.76489146348385));
#34057=CARTESIAN_POINT('Ctrl Pts',(0.0177855252092632,0.183012109670541,
-0.753773680446777));
#34058=CARTESIAN_POINT('Ctrl Pts',(-0.144153830975677,0.114146529548942,
-0.742655897409706));
#34059=CARTESIAN_POINT('Ctrl Pts',(-0.174060703964709,-0.0592674322739036,
-0.731538114372633));
#34060=CARTESIAN_POINT('Ctrl Pts',(-0.0445429760552296,-0.17839753495263,
-0.72042033133556));
#34061=CARTESIAN_POINT('Ctrl Pts',(0.125772278341771,-0.134130873380261,
-0.709302548298488));
#34062=CARTESIAN_POINT('Ctrl Pts',(0.180890967276192,0.032988106203831,
-0.698184765261415));
#34063=CARTESIAN_POINT('Ctrl Pts',(0.0703291228835756,0.169892824061108,
-0.687066982224344));
#34064=CARTESIAN_POINT('Ctrl Pts',(-0.104648135740215,0.151190359742707,
-0.675949199187271));
#34065=CARTESIAN_POINT('Ctrl Pts',(-0.183776722635436,-0.00598944157744644,
-0.664831416150198));
#34066=CARTESIAN_POINT('Ctrl Pts',(-0.0945816730450154,-0.157683430699099,
-0.653713633113126));
#34067=CARTESIAN_POINT('Ctrl Pts',(0.081242036168499,-0.164952989521948,
-0.642595850076053));
#34068=CARTESIAN_POINT('Ctrl Pts',(0.182655043268737,-0.0211398287960793,
-0.631478067038982));
#34069=CARTESIAN_POINT('Ctrl Pts',(0.116771775495109,0.142035592865843,
-0.620360284001909));
#34070=CARTESIAN_POINT('Ctrl Pts',(-0.0560643729717556,0.175118654849549,
-0.609242500964836));
#34071=CARTESIAN_POINT('Ctrl Pts',(-0.177550388513388,0.0478081241189917,
-0.598124717927763));
#34072=CARTESIAN_POINT('Ctrl Pts',(-0.136415552918731,-0.123290527271597,
-0.587006934890692));
#34073=CARTESIAN_POINT('Ctrl Pts',(0.0296641702068159,-0.181465683254363,
-0.575889151853619));
#34074=CARTESIAN_POINT('Ctrl Pts',(0.168574070457431,-0.0734339156142763,
-0.564771368816547));
#34075=CARTESIAN_POINT('Ctrl Pts',(0.153084653157532,0.101856988766946,
-0.553653585779474));
#34076=CARTESIAN_POINT('Ctrl Pts',(-0.00261711062509075,0.183855671451842,
-0.542535802742403));
#34077=CARTESIAN_POINT('Ctrl Pts',(-0.15592182666857,0.0974584073406097,
-0.531418019705329));
#34078=CARTESIAN_POINT('Ctrl Pts',(-0.166415589855949,-0.0782023570356304,
-0.520300236668257));
#34079=CARTESIAN_POINT('Ctrl Pts',(-0.0244870176639766,-0.182236503365697,
-0.509182453631186));
#34080=CARTESIAN_POINT('Ctrl Pts',(0.139869551941277,-0.119357721295182,
-0.498064670594112));
#34081=CARTESIAN_POINT('Ctrl Pts',(0.176117668643726,0.0528424449143884,
-0.486946887557041));
#34082=CARTESIAN_POINT('Ctrl Pts',(0.0510571821108666,0.176643486570915,
-0.475829104519967));
#34083=CARTESIAN_POINT('Ctrl Pts',(-0.120767282135644,0.138654321096036,
-0.464711321482895));
#34084=CARTESIAN_POINT('Ctrl Pts',(-0.181979326016571,-0.0263302505796173,
-0.453593538445823));
#34085=CARTESIAN_POINT('Ctrl Pts',(-0.0765139937801866,-0.167198582376871,
-0.44247575540875));
#34086=CARTESIAN_POINT('Ctrl Pts',(0.0990315612963532,-0.154927425139147,
-0.431357972371679));
#34087=CARTESIAN_POINT('Ctrl Pts',(0.183872742689355,-0.000756101129370498,
-0.420240189334605));
#34088=CARTESIAN_POINT('Ctrl Pts',(0.100302341504276,0.154107746339307,
-0.409122406297534));
#34089=CARTESIAN_POINT('Ctrl Pts',(-0.0751363584943781,0.167822182161027,
-0.398004623260461));
#34090=CARTESIAN_POINT('Ctrl Pts',(-0.181756630823041,0.0278259652989701,
-0.386886840223389));
#34091=CARTESIAN_POINT('Ctrl Pts',(-0.121903496635997,-0.13765643719383,
-0.375769057186316));
#34092=CARTESIAN_POINT('Ctrl Pts',(0.0496027324589358,-0.177057409124813,
-0.364651274149244));
#34093=CARTESIAN_POINT('Ctrl Pts',(0.175677134346707,-0.054289056541952,
-0.353533491112171));
#34094=CARTESIAN_POINT('Ctrl Pts',(0.140846424445151,0.118203392142091,
-0.342415708075099));
#34095=CARTESIAN_POINT('Ctrl Pts',(-0.0229874693739835,0.182431722699479,
-0.331297925038026));
#34096=CARTESIAN_POINT('Ctrl Pts',(-0.165766822739796,0.0795683207540087,
-0.320180142000955));
#34097=CARTESIAN_POINT('Ctrl Pts',(-0.156718055506932,-0.0961728042196944,
-0.309062358963882));
#34098=CARTESIAN_POINT('Ctrl Pts',(-0.00412905838771584,-0.183827930642512,
-0.29794457592681));
#34099=CARTESIAN_POINT('Ctrl Pts',(0.152241800199334,-0.103112518319205,
-0.286826792889737));
#34100=CARTESIAN_POINT('Ctrl Pts',(0.169172293136615,0.0720450722777397,
-0.275709009852665));
#34101=CARTESIAN_POINT('Ctrl Pts',(0.031155547779449,0.181215587419735,
-0.264591226815592));
#34102=CARTESIAN_POINT('Ctrl Pts',(-0.135396993113368,0.124408244199608,
-0.25347344377852));
#34103=CARTESIAN_POINT('Ctrl Pts',(-0.17793756067556,-0.0463463249500769,
-0.242355660741447));
#34104=CARTESIAN_POINT('Ctrl Pts',(-0.0575026584572911,-0.174651658969645,
-0.231237877704375));
#34105=CARTESIAN_POINT('Ctrl Pts',(0.115599717800877,-0.142991121590197,
-0.220120094667303));
#34106=CARTESIAN_POINT('Ctrl Pts',(0.182822725577002,0.0196369447459957,
-0.209002311630231));
#34107=CARTESIAN_POINT('Ctrl Pts',(0.0825958599644629,0.164279286494686,
-0.197884528593158));
#34108=CARTESIAN_POINT('Ctrl Pts',(-0.0932816632585158,0.158455916717979,
-0.186766745556086));
#34109=CARTESIAN_POINT('Ctrl Pts',(-0.183721281618962,0.00750067334506049,
-0.175648962519013));
#34110=CARTESIAN_POINT('Ctrl Pts',(-0.105887932579898,-0.150324706413772,
-0.164531179481941));
#34111=CARTESIAN_POINT('Ctrl Pts',(0.0689294256808382,-0.170465296791246,
-0.153413396444868));
#34112=CARTESIAN_POINT('Ctrl Pts',(0.18061377047412,-0.0344749710973018,
-0.142295613407796));
#34113=CARTESIAN_POINT('Ctrl Pts',(0.126870711401792,0.133092601640971,
-0.131177830370724));
#34114=CARTESIAN_POINT('Ctrl Pts',(-0.0430735388430987,0.178756644275882,
-0.120060047333651));
#34115=CARTESIAN_POINT('Ctrl Pts',(-0.173568889044906,0.0606991572905674,
-0.108942264296579));
#34116=CARTESIAN_POINT('Ctrl Pts',(-0.145084867506489,-0.11296141928049,
-0.0978244812595066));
#34117=CARTESIAN_POINT('Ctrl Pts',(0.016274431326597,-0.183144050045734,
-0.0867066982224341));
#34118=CARTESIAN_POINT('Ctrl Pts',(0.162746700955473,-0.0856111115207315,
-0.0755889151853617));
#34119=CARTESIAN_POINT('Ctrl Pts',(0.160120950075793,0.0903886722456795,
-0.0644711321482895));
#34120=CARTESIAN_POINT('Ctrl Pts',(0.0109069706335314,0.18349634534749,
-0.0533533491112173));
#34121=CARTESIAN_POINT('Ctrl Pts',(-0.148428680391759,0.108737123459702,
-0.0422355660741448));
#34122=CARTESIAN_POINT('Ctrl Pts',(-0.171557183147855,-0.066015722996037,
-0.0311177830370724));
#34123=CARTESIAN_POINT('Ctrl Pts',(-0.0826006812134621,-0.141598846131356,
-0.0237059276790242));
#34124=CARTESIAN_POINT('Ctrl Pts',(-0.0319621170202007,-0.152230829911641,
-0.02));
#34125=CARTESIAN_POINT('Ctrl Pts',(-0.0744392439309354,0.151537102412033,
-1.57993827215147));
#34126=CARTESIAN_POINT('Ctrl Pts',(-0.124847044325944,0.126775387360737,
-1.57623234447245));
#34127=CARTESIAN_POINT('Ctrl Pts',(-0.198137894813896,0.0234259443652476,
-1.5688204891144));
#34128=CARTESIAN_POINT('Ctrl Pts',(-0.126949727137059,-0.154167492477815,
-1.55770270607733));
#34129=CARTESIAN_POINT('Ctrl Pts',(0.0606789246064021,-0.1900667869665,
-1.54658492304025));
#34130=CARTESIAN_POINT('Ctrl Pts',(0.192645880859905,-0.0521269260237622,
-1.53546714000318));
#34131=CARTESIAN_POINT('Ctrl Pts',(0.148210276971067,0.133684398496491,
-1.52434935696611));
#34132=CARTESIAN_POINT('Ctrl Pts',(-0.0319965018674015,0.196985400300458,
-1.51323157392904));
#34133=CARTESIAN_POINT('Ctrl Pts',(-0.182884983438119,0.0798999096835992,
-1.50211379089196));
#34134=CARTESIAN_POINT('Ctrl Pts',(-0.166273026361208,-0.11038548084507,
-1.49099600785489));
#34135=CARTESIAN_POINT('Ctrl Pts',(0.00263407498332024,-0.199557581114583,
-1.47987822481782));
#34136=CARTESIAN_POINT('Ctrl Pts',(0.169126812148914,-0.105957238372422,
-1.46876044178075));
#34137=CARTESIAN_POINT('Ctrl Pts',(0.180714902576048,0.0846934808638075,
-1.45764265874367));
#34138=CARTESIAN_POINT('Ctrl Pts',(0.0267832286938344,0.197770864138438,
-1.4465248757066));
#34139=CARTESIAN_POINT('Ctrl Pts',(-0.151679315935036,0.129707923455094,
-1.43540709266953));
#34140=CARTESIAN_POINT('Ctrl Pts',(-0.191216817426186,-0.057156683129376,
-1.42428930963246));
#34141=CARTESIAN_POINT('Ctrl Pts',(-0.0556161256890393,-0.191670490560431,
-1.41317152659538));
#34142=CARTESIAN_POINT('Ctrl Pts',(0.130924105664016,-0.15063075786586,
-1.40205374355831));
#34143=CARTESIAN_POINT('Ctrl Pts',(0.197549161483521,0.0283738211519969,
-1.39093596052124));
#34144=CARTESIAN_POINT('Ctrl Pts',(0.0832362036722443,0.181390396164102,
-1.37981817748417));
#34145=CARTESIAN_POINT('Ctrl Pts',(-0.107313936358152,0.168269019611732,
-1.3687003944471));
#34146=CARTESIAN_POINT('Ctrl Pts',(-0.199573763938466,0.00102771760510595,
-1.35758261141002));
#34147=CARTESIAN_POINT('Ctrl Pts',(-0.109041225395815,-0.167154880839191,
-1.34646482837295));
#34148=CARTESIAN_POINT('Ctrl Pts',(0.0813636755300989,-0.182238019349389,
-1.33534704533588));
#34149=CARTESIAN_POINT('Ctrl Pts',(0.197246463586825,-0.0304068397613748,
-1.32422926229881));
#34150=CARTESIAN_POINT('Ctrl Pts',(0.132468493312827,0.149274383372008,
-1.31311147926173));
#34151=CARTESIAN_POINT('Ctrl Pts',(-0.0536391980130076,0.192233139030937,
-1.30199369622466));
#34152=CARTESIAN_POINT('Ctrl Pts',(-0.190618007687202,0.0591229095519548,
-1.29087591318759));
#34153=CARTESIAN_POINT('Ctrl Pts',(-0.153007153451631,-0.128138808625108,
-1.27975813015052));
#34154=CARTESIAN_POINT('Ctrl Pts',(0.0247450641999012,-0.198036423641172,
-1.26864034711344));
#34155=CARTESIAN_POINT('Ctrl Pts',(0.179832936063426,-0.0865497452034227,
-1.25752256407637));
#34156=CARTESIAN_POINT('Ctrl Pts',(0.170209339984542,0.104209039288979,
-1.2464047810393));
#34157=CARTESIAN_POINT('Ctrl Pts',(0.00468866043001303,0.199521326559181,
-1.23528699800223));
#34158=CARTESIAN_POINT('Ctrl Pts',(-0.165126427919824,0.11208927732182,
-1.22416921496515));
#34159=CARTESIAN_POINT('Ctrl Pts',(-0.183699942098113,-0.0780068879088045,
-1.21305143192808));
#34160=CARTESIAN_POINT('Ctrl Pts',(-0.0340201441448589,-0.196655467965102,
-1.20193364889101));
#34161=CARTESIAN_POINT('Ctrl Pts',(0.146819173328295,-0.135184590953742,
-1.19081586585394));
#34162=CARTESIAN_POINT('Ctrl Pts',(0.193184783761432,0.0501037185365196,
-1.17969808281687));
#34163=CARTESIAN_POINT('Ctrl Pts',(0.0626097846870554,0.189501340759367,
-1.16858029977979));
#34164=CARTESIAN_POINT('Ctrl Pts',(-0.125310380233048,0.155332069753783,
-1.15746251674272));
#34165=CARTESIAN_POINT('Ctrl Pts',(-0.198457038542795,-0.0211079876106242,
-1.14634473370565));
#34166=CARTESIAN_POINT('Ctrl Pts',(-0.0898341564306036,-0.178214947820184,
-1.13522695066857));
#34167=CARTESIAN_POINT('Ctrl Pts',(0.101069069319104,-0.172092377853052,
-1.1241091676315));
#34168=CARTESIAN_POINT('Ctrl Pts',(0.199401739668498,-0.0083480240371076,
-1.11299138459443));
#34169=CARTESIAN_POINT('Ctrl Pts',(0.115099604797503,0.163042400201931,
-1.10187360155736));
#34170=CARTESIAN_POINT('Ctrl Pts',(-0.0746238465478801,0.185100040017679,
-1.09075581852028));
#34171=CARTESIAN_POINT('Ctrl Pts',(-0.195998286988311,0.0376219986948521,
-1.07963803548322));
#34172=CARTESIAN_POINT('Ctrl Pts',(-0.137855191487726,-0.144314550437683,
-1.06852025244614));
#34173=CARTESIAN_POINT('Ctrl Pts',(0.0465513763769294,-0.194071411201035,
-1.05740246940907));
#34174=CARTESIAN_POINT('Ctrl Pts',(0.188320896182345,-0.0660755881489248,
-1.046284686372));
#34175=CARTESIAN_POINT('Ctrl Pts',(0.15760470823831,0.122439777969681,-1.03516690333492));
#34176=CARTESIAN_POINT('Ctrl Pts',(-0.0174638070162759,0.198810861706915,
-1.02404912029785));
#34177=CARTESIAN_POINT('Ctrl Pts',(-0.176536980414133,0.0930883335032248,
-1.01293133726078));
#34178=CARTESIAN_POINT('Ctrl Pts',(-0.173917497139423,-0.0978950840282937,
-1.00181355422371));
#34179=CARTESIAN_POINT('Ctrl Pts',(-0.0120045780738169,-0.199215043090168,
-0.990695771186635));
#34180=CARTESIAN_POINT('Ctrl Pts',(0.160903499719639,-0.118071194904261,
-0.979577988149561));
#34181=CARTESIAN_POINT('Ctrl Pts',(0.186437841559585,0.0712156901444556,
-0.96846020511249));
#34182=CARTESIAN_POINT('Ctrl Pts',(0.0412111913662969,0.195275141772624,
-0.957342422075417));
#34183=CARTESIAN_POINT('Ctrl Pts',(-0.141761357737385,0.140479396142641,
-0.946224639038345));
#34184=CARTESIAN_POINT('Ctrl Pts',(-0.194892722901607,-0.0429833671103725,
-0.935106856001272));
#34185=CARTESIAN_POINT('Ctrl Pts',(-0.0695191535292426,-0.187077071231953,
-0.9239890729642));
#34186=CARTESIAN_POINT('Ctrl Pts',(0.119527967964621,-0.159824304041645,
-0.912871289927129));
#34187=CARTESIAN_POINT('Ctrl Pts',(0.199097774045392,0.0138137488871811,
-0.901753506890054));
#34188=CARTESIAN_POINT('Ctrl Pts',(0.0963111812148712,0.174799598572606,
-0.890635723852983));
#34189=CARTESIAN_POINT('Ctrl Pts',(-0.0946881516397165,0.175684083590979,
-0.87951794081591));
#34190=CARTESIAN_POINT('Ctrl Pts',(-0.198961299656857,0.0156570919075729,
-0.868400157778838));
#34191=CARTESIAN_POINT('Ctrl Pts',(-0.121003047538591,-0.158710446330799,
-0.857282374741765));
#34192=CARTESIAN_POINT('Ctrl Pts',(0.0677835657315107,-0.18771289647989,
-0.846164591704693));
#34193=CARTESIAN_POINT('Ctrl Pts',(0.194486275696159,-0.0447865141977529,
-0.835046808667621));
#34194=CARTESIAN_POINT('Ctrl Pts',(0.143056321728893,0.139160454517608,
-0.823929025630549));
#34195=CARTESIAN_POINT('Ctrl Pts',(-0.0394008915688968,0.195648442446455,
-0.812811242593476));
#34196=CARTESIAN_POINT('Ctrl Pts',(-0.185770284523904,0.0729393218782279,
-0.801693459556404));
#34197=CARTESIAN_POINT('Ctrl Pts',(-0.161990110147327,-0.116575930202614,
-0.790575676519331));
#34198=CARTESIAN_POINT('Ctrl Pts',(0.0101590416693245,-0.199317678996392,
-0.779457893482259));
#34199=CARTESIAN_POINT('Ctrl Pts',(0.173003387020459,-0.0995016148994445,
-0.768340110445186));
#34200=CARTESIAN_POINT('Ctrl Pts',(0.177391542653899,0.0914493514630801,
-0.757222327408114));
#34201=CARTESIAN_POINT('Ctrl Pts',(0.0193043362659213,0.198640594767233,
-0.746104544371042));
#34202=CARTESIAN_POINT('Ctrl Pts',(-0.15646397811889,0.123894175970298,
-0.73498676133397));
#34203=CARTESIAN_POINT('Ctrl Pts',(-0.188924775652256,-0.0643286284082972,
-0.723868978296897));
#34204=CARTESIAN_POINT('Ctrl Pts',(-0.0483467638957979,-0.193631954255882,
-0.712751195259825));
#34205=CARTESIAN_POINT('Ctrl Pts',(0.136512716125805,-0.145585100968826,
-0.701633412222752));
#34206=CARTESIAN_POINT('Ctrl Pts',(0.19633831549425,0.0358051554532093,
-0.690515629185681));
#34207=CARTESIAN_POINT('Ctrl Pts',(0.0763349421205001,0.184400975864033,
-0.679397846148607));
#34208=CARTESIAN_POINT('Ctrl Pts',(-0.113584658207261,0.164101397642091,
-0.668280063111536));
#34209=CARTESIAN_POINT('Ctrl Pts',(-0.199470502549766,-0.00650091537335537,
-0.657162280074462));
#34210=CARTESIAN_POINT('Ctrl Pts',(-0.102658560799958,-0.171148950281995,
-0.646044497037391));
#34211=CARTESIAN_POINT('Ctrl Pts',(0.0881797735333642,-0.179039299673989,
-0.634926714000318));
#34212=CARTESIAN_POINT('Ctrl Pts',(0.198253036356188,-0.0229450836498757,
-0.623808930963246));
#34213=CARTESIAN_POINT('Ctrl Pts',(0.126743607175127,0.154164851144433,
-0.612691147926174));
#34214=CARTESIAN_POINT('Ctrl Pts',(-0.0608520409518781,0.190073071212465,
-0.601573364889101));
#34215=CARTESIAN_POINT('Ctrl Pts',(-0.192712464978101,0.0518907422399437,
-0.590455581852028));
#34216=CARTESIAN_POINT('Ctrl Pts',(-0.14806488278868,-0.133819033672054,
-0.579337798814956));
#34217=CARTESIAN_POINT('Ctrl Pts',(0.0321973689269302,-0.196962109864641,
-0.568220015777883));
#34218=CARTESIAN_POINT('Ctrl Pts',(0.182969606100265,-0.0797048714424761,
-0.557102232740812));
#34219=CARTESIAN_POINT('Ctrl Pts',(0.166157455961192,0.11055515870665,-0.545984449703739));
#34220=CARTESIAN_POINT('Ctrl Pts',(-0.00284060116063022,0.199556193271956,
-0.534866666666666));
#34221=CARTESIAN_POINT('Ctrl Pts',(-0.169236912477511,0.105780956429914,
-0.523748883629594));
#34222=CARTESIAN_POINT('Ctrl Pts',(-0.180626800090086,-0.0848805182439657,
-0.512631100592522));
#34223=CARTESIAN_POINT('Ctrl Pts',(-0.0265781087470362,-0.197798754858514,
-0.501513317555449));
#34224=CARTESIAN_POINT('Ctrl Pts',(0.151813839190521,-0.129550382162242,
-0.490395534518377));
#34225=CARTESIAN_POINT('Ctrl Pts',(0.191157396695698,0.0573549734257742,
-0.479277751481304));
#34226=CARTESIAN_POINT('Ctrl Pts',(0.0554172564859194,0.191728117321693,
-0.468159968444232));
#34227=CARTESIAN_POINT('Ctrl Pts',(-0.13108031372914,0.150494832605041,
-0.457042185407159));
#34228=CARTESIAN_POINT('Ctrl Pts',(-0.1975196156164,-0.0285787462093131,
-0.445924402370088));
#34229=CARTESIAN_POINT('Ctrl Pts',(-0.0830479756769845,-0.181476656967502,
-0.434806619333015));
#34230=CARTESIAN_POINT('Ctrl Pts',(0.107488451294552,-0.168157593127565,
-0.423688836295943));
#34231=CARTESIAN_POINT('Ctrl Pts',(0.199574722323279,-0.000820669071094855,
-0.41257105325887));
#34232=CARTESIAN_POINT('Ctrl Pts',(0.108867750930925,0.167267917113166,
-0.401453270221799));
#34233=CARTESIAN_POINT('Ctrl Pts',(-0.0815526959764324,0.18215350962083,
-0.390335487184724));
#34234=CARTESIAN_POINT('Ctrl Pts',(-0.197277903164835,0.0302021888437342,
-0.379217704147654));
#34235=CARTESIAN_POINT('Ctrl Pts',(-0.132313556297296,-0.149411733501928,
-0.368099921110581));
#34236=CARTESIAN_POINT('Ctrl Pts',(0.0538386027867795,-0.192177387167509,
-0.356982138073509));
#34237=CARTESIAN_POINT('Ctrl Pts',(0.190679242572821,-0.0589251197653465,
-0.345864355036436));
#34238=CARTESIAN_POINT('Ctrl Pts',(0.152874132607884,0.128297478024148,
-0.334746571999364));
#34239=CARTESIAN_POINT('Ctrl Pts',(-0.0249505051707323,0.198010645124367,
-0.323628788962291));
#34240=CARTESIAN_POINT('Ctrl Pts',(-0.179922630917619,0.0863631296730007,
-0.312511005925219));
#34241=CARTESIAN_POINT('Ctrl Pts',(-0.170101135999703,-0.104385568064449,
-0.301393222888146));
#34242=CARTESIAN_POINT('Ctrl Pts',(-0.00448166307377801,-0.199526083511052,
-0.290275439851074));
#34243=CARTESIAN_POINT('Ctrl Pts',(0.165242626810163,-0.111917905343786,
-0.279157656814001));
#34244=CARTESIAN_POINT('Ctrl Pts',(0.183618914547724,0.0781974265695377,
-0.26803987377693));
#34245=CARTESIAN_POINT('Ctrl Pts',(0.0338161040400543,0.196690656869379,
-0.256922090739857));
#34246=CARTESIAN_POINT('Ctrl Pts',(-0.146959342144907,0.135032199050898,
-0.245804307702785));
#34247=CARTESIAN_POINT('Ctrl Pts',(-0.193132700058226,-0.0503041114051506,
-0.234686524665712));
#34248=CARTESIAN_POINT('Ctrl Pts',(-0.0624131501309722,-0.189566195795832,
-0.22356874162864));
#34249=CARTESIAN_POINT('Ctrl Pts',(0.125471460551042,-0.155201978110864,
-0.212450958591567));
#34250=CARTESIAN_POINT('Ctrl Pts',(0.198435038047255,0.0213138594532229,
-0.201333175554495));
#34251=CARTESIAN_POINT('Ctrl Pts',(0.0896492083402993,0.178308065165666,
-0.190215392517423));
#34252=CARTESIAN_POINT('Ctrl Pts',(-0.101247535498635,0.171987403445101,
-0.17909760948035));
#34253=CARTESIAN_POINT('Ctrl Pts',(-0.199410327097406,0.0081412001484483,
-0.167979826443278));
#34254=CARTESIAN_POINT('Ctrl Pts',(-0.114930328622562,-0.163161821061985,
-0.156862043406206));
#34255=CARTESIAN_POINT('Ctrl Pts',(0.0748157165056128,-0.185022335422193,
-0.145744260369133));
#34256=CARTESIAN_POINT('Ctrl Pts',(0.196037447219847,-0.0374189925228408,
-0.134626477332061));
#34257=CARTESIAN_POINT('Ctrl Pts',(0.137704950873262,0.144458165072649,
-0.123508694294988));
#34258=CARTESIAN_POINT('Ctrl Pts',(-0.0467518427601612,0.194021730045504,
-0.112390911257916));
#34259=CARTESIAN_POINT('Ctrl Pts',(-0.188390961751301,0.0658826168813301,
-0.101273128220844));
#34260=CARTESIAN_POINT('Ctrl Pts',(-0.157474521358699,-0.122607862135579,
-0.090155345183771));
#34261=CARTESIAN_POINT('Ctrl Pts',(0.0176642011505863,-0.198783802310435,
-0.0790375621466987));
#34262=CARTESIAN_POINT('Ctrl Pts',(0.176644603094283,-0.0929219500380387,
-0.0679197791096262));
#34263=CARTESIAN_POINT('Ctrl Pts',(0.173794623836686,0.0981074948943239,
-0.056801996072554));
#34264=CARTESIAN_POINT('Ctrl Pts',(0.0118383812833686,0.199166182189015,
-0.0456842130354818));
#34265=CARTESIAN_POINT('Ctrl Pts',(-0.161103882178133,0.118022828741753,
-0.0345664299984093));
#34266=CARTESIAN_POINT('Ctrl Pts',(-0.186207464404562,-0.0716531955373244,
-0.0234486469613369));
#34267=CARTESIAN_POINT('Ctrl Pts',(-0.0896544413042297,-0.153690808026425,
-0.0160367916032887));
#34268=CARTESIAN_POINT('Ctrl Pts',(-0.0346915509926754,-0.165230719704803,
-0.0123308639242645));
#34269=CARTESIAN_POINT('Ctrl Pts',(-0.0802959149489957,0.163459616787393,
-1.57226913607574));
#34270=CARTESIAN_POINT('Ctrl Pts',(-0.134669659758104,0.136749719416661,
-1.56856320839671));
#34271=CARTESIAN_POINT('Ctrl Pts',(-0.213726828887605,0.0252690319920107,
-1.56115135303866));
#34272=CARTESIAN_POINT('Ctrl Pts',(-0.136937775757814,-0.166296958569109,
-1.55003357000159));
#34273=CARTESIAN_POINT('Ctrl Pts',(0.0654529722778036,-0.205020708902561,
-1.53891578696452));
#34274=CARTESIAN_POINT('Ctrl Pts',(0.20780271867287,-0.0562281264226708,
-1.52779800392744));
#34275=CARTESIAN_POINT('Ctrl Pts',(0.159871046047665,0.14420231217879,-1.51668022089037));
#34276=CARTESIAN_POINT('Ctrl Pts',(-0.0345138969304135,0.212483659336931,
-1.5055624378533));
#34277=CARTESIAN_POINT('Ctrl Pts',(-0.19727386120714,0.0861862105738098,
-1.49444465481623));
#34278=CARTESIAN_POINT('Ctrl Pts',(-0.179354921919933,-0.119070301006325,
-1.48332687177916));
#34279=CARTESIAN_POINT('Ctrl Pts',(0.00284131661823614,-0.215258212126264,
-1.47220908874208));
#34280=CARTESIAN_POINT('Ctrl Pts',(0.182433235572673,-0.114293656830746,
-1.46109130570501));
#34281=CARTESIAN_POINT('Ctrl Pts',(0.19493304446678,0.0913569264954411,
-1.44997352266794));
#34282=CARTESIAN_POINT('Ctrl Pts',(0.0288904580392435,0.213330921267592,
-1.43885573963087));
#34283=CARTESIAN_POINT('Ctrl Pts',(-0.163613019271682,0.1399129792294,-1.42773795659379));
#34284=CARTESIAN_POINT('Ctrl Pts',(-0.206261220534644,-0.0616536107161584,
-1.41662017355672));
#34285=CARTESIAN_POINT('Ctrl Pts',(-0.0599918465354529,-0.206750587399193,
-1.40550239051965));
#34286=CARTESIAN_POINT('Ctrl Pts',(0.141224847244886,-0.162481963593313,
-1.39438460748258));
#34287=CARTESIAN_POINT('Ctrl Pts',(0.213091775669342,0.0306061938527011,
-1.38326682444551));
#34288=CARTESIAN_POINT('Ctrl Pts',(0.0897849948200019,0.195661683996559,
-1.37214904140843));
#34289=CARTESIAN_POINT('Ctrl Pts',(-0.115757096010416,0.181507954323534,
-1.36103125837136));
#34290=CARTESIAN_POINT('Ctrl Pts',(-0.215275668169361,0.00110857554501473,
-1.34991347533429));
#34291=CARTESIAN_POINT('Ctrl Pts',(-0.117620283307016,-0.180306158235917,
-1.33879569229721));
#34292=CARTESIAN_POINT('Ctrl Pts',(0.0877651414133644,-0.196575995797707,
-1.32767790926014));
#34293=CARTESIAN_POINT('Ctrl Pts',(0.212765262350764,-0.0327991646665892,
-1.31656012622307));
#34294=CARTESIAN_POINT('Ctrl Pts',(0.142890742984133,0.161018873356952,
-1.305442343186));
#34295=CARTESIAN_POINT('Ctrl Pts',(-0.0578593797322928,0.207357503473944,
-1.29432456014893));
#34296=CARTESIAN_POINT('Ctrl Pts',(-0.205615298124191,0.0637745343212453,
-1.28320677711185));
#34297=CARTESIAN_POINT('Ctrl Pts',(-0.165045327321419,-0.138220410843686,
-1.27208899407478));
#34298=CARTESIAN_POINT('Ctrl Pts',(0.0266919364770298,-0.213617374247491,
-1.26097121103771));
#34299=CARTESIAN_POINT('Ctrl Pts',(0.193981687301585,-0.0933592365091615,
-1.24985342800064));
#34300=CARTESIAN_POINT('Ctrl Pts',(0.183600933663484,0.112407914344587,
-1.23873564496356));
#34301=CARTESIAN_POINT('Ctrl Pts',(0.00505755108773542,0.215219105164084,
-1.22761786192649));
#34302=CARTESIAN_POINT('Ctrl Pts',(-0.178118112327731,0.120908147413182,
-1.21650007888942));
#34303=CARTESIAN_POINT('Ctrl Pts',(-0.198152938529722,-0.0841442511529614,
-1.20538229585235));
#34304=CARTESIAN_POINT('Ctrl Pts',(-0.0366967537088725,-0.212127768850411,
-1.19426451281527));
#34305=CARTESIAN_POINT('Ctrl Pts',(0.158370494270313,-0.145820535572709,
-1.1831467297782));
#34306=CARTESIAN_POINT('Ctrl Pts',(0.208384020943847,0.0540457386425016,
-1.17202894674113));
#34307=CARTESIAN_POINT('Ctrl Pts',(0.0675357470163338,0.20441077497311,
-1.16091116370406));
#34308=CARTESIAN_POINT('Ctrl Pts',(-0.135169449635391,0.167553161520197,
-1.14979338066698));
#34309=CARTESIAN_POINT('Ctrl Pts',(-0.214071081950358,-0.0227687048984483,
-1.13867559762991));
#34310=CARTESIAN_POINT('Ctrl Pts',(-0.0969020560036732,-0.192236400279482,
-1.12755781459284));
#34311=CARTESIAN_POINT('Ctrl Pts',(0.109020900340556,-0.185632123672291,
-1.11644003155577));
#34312=CARTESIAN_POINT('Ctrl Pts',(0.215090109512111,-0.00900482316421355,
-1.1053222485187));
#34313=CARTESIAN_POINT('Ctrl Pts',(0.124155319015036,0.175870119151678,
-1.09420446548162));
#34314=CARTESIAN_POINT('Ctrl Pts',(-0.0804950415822979,0.199663192228349,
-1.08308668244455));
#34315=CARTESIAN_POINT('Ctrl Pts',(-0.211418882716809,0.0405819920768663,
-1.07196889940748));
#34316=CARTESIAN_POINT('Ctrl Pts',(-0.148701251469534,-0.155668814672513,
-1.06085111637041));
#34317=CARTESIAN_POINT('Ctrl Pts',(0.0502139081609773,-0.209340405744691,
-1.04973333333333));
#34318=CARTESIAN_POINT('Ctrl Pts',(0.203137456326208,-0.0712742301780164,
-1.03861555029626));
#34319=CARTESIAN_POINT('Ctrl Pts',(0.170004604829223,0.13207299643383,-1.02749776725919));
#34320=CARTESIAN_POINT('Ctrl Pts',(-0.0188378103915933,0.214452742929068,
-1.01637998422212));
#34321=CARTESIAN_POINT('Ctrl Pts',(-0.190426415102195,0.100412262605108,
-1.00526220118504));
#34322=CARTESIAN_POINT('Ctrl Pts',(-0.187600838227293,-0.105597194785504,
-0.994144418147971));
#34323=CARTESIAN_POINT('Ctrl Pts',(-0.0129490646211849,-0.214888724170412,
-0.9830266351109));
#34324=CARTESIAN_POINT('Ctrl Pts',(0.173562935975961,-0.127360705500382,
-0.971908852073825));
#34325=CARTESIAN_POINT('Ctrl Pts',(0.201106248244974,0.0768187409880018,
-0.960791069036756));
#34326=CARTESIAN_POINT('Ctrl Pts',(0.0444535723652056,0.210638842462928,
-0.94967328599968));
#34327=CARTESIAN_POINT('Ctrl Pts',(-0.152914743928569,0.151531921189599,
-0.93855550296261));
#34328=CARTESIAN_POINT('Ctrl Pts',(-0.210226335947272,-0.0463651779284336,
-0.927437719925536));
#34329=CARTESIAN_POINT('Ctrl Pts',(-0.0749887256282371,-0.201795770715849,
-0.916319936888466));
#34330=CARTESIAN_POINT('Ctrl Pts',(0.128932093380988,-0.172398832207608,
-0.905202153851391));
#34331=CARTESIAN_POINT('Ctrl Pts',(0.214762228725962,0.0149005759220357,
-0.894084370814321));
#34332=CARTESIAN_POINT('Ctrl Pts',(0.10388867493928,0.188552340928219,-0.882966587777247));
#34333=CARTESIAN_POINT('Ctrl Pts',(-0.102137949947401,0.189506414748137,
-0.871848804740174));
#34334=CARTESIAN_POINT('Ctrl Pts',(-0.214615016915151,0.016888948003362,
-0.860731021703104));
#34335=CARTESIAN_POINT('Ctrl Pts',(-0.130523228080374,-0.171197339294831,
-0.849613238666029));
#34336=CARTESIAN_POINT('Ctrl Pts',(0.0731165866483921,-0.202481620911723,
-0.838495455628959));
#34337=CARTESIAN_POINT('Ctrl Pts',(0.209787910615195,-0.0483101915734308,
-0.827377672591884));
#34338=CARTESIAN_POINT('Ctrl Pts',(0.154311592056428,0.150109208935231,
-0.816259889554814));
#34339=CARTESIAN_POINT('Ctrl Pts',(-0.0425008432550175,0.211041513387208,
-0.80514210651774));
#34340=CARTESIAN_POINT('Ctrl Pts',(-0.200386169693257,0.0786779832342944,
-0.794024323480669));
#34341=CARTESIAN_POINT('Ctrl Pts',(-0.17473503786573,-0.125747797564063,
-0.782906540443596));
#34342=CARTESIAN_POINT('Ctrl Pts',(0.0109583265864464,-0.214999435181992,
-0.771788757406523));
#34343=CARTESIAN_POINT('Ctrl Pts',(0.186614808486925,-0.107330123001603,
-0.760670974369452));
#34344=CARTESIAN_POINT('Ctrl Pts',(0.191348211903174,0.098644330053018,
-0.749553191332378));
#34345=CARTESIAN_POINT('Ctrl Pts',(0.0208231473225793,0.214269079863924,
-0.738435408295307));
#34346=CARTESIAN_POINT('Ctrl Pts',(-0.168774125262104,0.133641822391654,
-0.727317625258233));
#34347=CARTESIAN_POINT('Ctrl Pts',(-0.203788847339803,-0.0693898245426907,
-0.716199842221162));
#34348=CARTESIAN_POINT('Ctrl Pts',(-0.0521505517363663,-0.208866373559133,
-0.705082059184089));
#34349=CARTESIAN_POINT('Ctrl Pts',(0.147253153909839,-0.157039328557391,
-0.693964276147018));
#34350=CARTESIAN_POINT('Ctrl Pts',(0.211785663712306,0.0386222047025875,
-0.682846493109943));
#34351=CARTESIAN_POINT('Ctrl Pts',(0.0823407613574247,0.198909127666958,
-0.671728710072873));
#34352=CARTESIAN_POINT('Ctrl Pts',(-0.122521180674308,0.177012435541474,
-0.660610927035799));
#34353=CARTESIAN_POINT('Ctrl Pts',(-0.215164282464097,-0.00701238916926441,
-0.649493143998728));
#34354=CARTESIAN_POINT('Ctrl Pts',(-0.110735448554901,-0.184614469864892,
-0.638375360961654));
#34355=CARTESIAN_POINT('Ctrl Pts',(0.0951175108982293,-0.193125609826029,
-0.627257577924583));
#34356=CARTESIAN_POINT('Ctrl Pts',(0.21385102944364,-0.0247503385036721,
-0.61613979488751));
#34357=CARTESIAN_POINT('Ctrl Pts',(0.136715438855145,0.166294109423022,
-0.605022011850438));
#34358=CARTESIAN_POINT('Ctrl Pts',(-0.0656397089320004,0.205027487575381,
-0.593904228813365));
#34359=CARTESIAN_POINT('Ctrl Pts',(-0.207874541442814,0.0559733603608955,
-0.582786445776292));
#34360=CARTESIAN_POINT('Ctrl Pts',(-0.159714212658629,-0.14434754007251,
-0.571668662739221));
#34361=CARTESIAN_POINT('Ctrl Pts',(0.0347305676470442,-0.212458536474919,
-0.560550879702147));
#34362=CARTESIAN_POINT('Ctrl Pts',(0.197365141743099,-0.0859758272706753,
-0.549433096665076));
#34363=CARTESIAN_POINT('Ctrl Pts',(0.179230258764851,0.119253328646353,
-0.538315313628003));
#34364=CARTESIAN_POINT('Ctrl Pts',(-0.00306409169616951,0.215256715092069,
-0.527197530590932));
#34365=CARTESIAN_POINT('Ctrl Pts',(-0.182551998286452,0.114103505519217,
-0.516079747553858));
#34366=CARTESIAN_POINT('Ctrl Pts',(-0.194838010324222,-0.0915586794523007,
-0.504961964516786));
#34367=CARTESIAN_POINT('Ctrl Pts',(-0.0286691998300962,-0.213361006351331,
-0.493844181479714));
#34368=CARTESIAN_POINT('Ctrl Pts',(0.163758126439765,-0.139743043029301,
-0.482726398442641));
#34369=CARTESIAN_POINT('Ctrl Pts',(0.20619712474767,0.0618675019371596,
-0.471608615405569));
#34370=CARTESIAN_POINT('Ctrl Pts',(0.0597773308609723,0.206812748072472,
-0.460490832368497));
#34371=CARTESIAN_POINT('Ctrl Pts',(-0.141393345322637,0.162335344114046,
-0.449373049331423));
#34372=CARTESIAN_POINT('Ctrl Pts',(-0.21305990521623,-0.0308272418390084,
-0.438255266294353));
#34373=CARTESIAN_POINT('Ctrl Pts',(-0.0895819575737826,-0.195754731558133,
-0.427137483257279));
#34374=CARTESIAN_POINT('Ctrl Pts',(0.11594534129275,-0.181387761115983,
-0.416019700220208));
#34375=CARTESIAN_POINT('Ctrl Pts',(0.215276701957203,-0.000885237012819617,
-0.404901917183134));
#34376=CARTESIAN_POINT('Ctrl Pts',(0.117433160357574,0.180428087887024,
-0.393784134146063));
#34377=CARTESIAN_POINT('Ctrl Pts',(-0.087969033458487,0.196484837080633,
-0.382666351108989));
#34378=CARTESIAN_POINT('Ctrl Pts',(-0.212799175506629,0.0325784123884988,
-0.371548568071918));
#34379=CARTESIAN_POINT('Ctrl Pts',(-0.142723615958594,-0.161167029810026,
-0.360430785034845));
#34380=CARTESIAN_POINT('Ctrl Pts',(0.0580744731146232,-0.207297365210204,
-0.349313001997773));
#34381=CARTESIAN_POINT('Ctrl Pts',(0.205681350798936,-0.0635611829887412,
-0.3381952189607));
#34382=CARTESIAN_POINT('Ctrl Pts',(0.164901840770617,0.138391563906206,
-0.327077435923628));
#34383=CARTESIAN_POINT('Ctrl Pts',(-0.0269135409674812,0.213589567549256,
-0.315959652886555));
#34384=CARTESIAN_POINT('Ctrl Pts',(-0.194078439095441,0.0931579385919925,
-0.304841869849484));
#34385=CARTESIAN_POINT('Ctrl Pts',(-0.183484216492474,-0.112598331909203,
-0.293724086812411));
#34386=CARTESIAN_POINT('Ctrl Pts',(-0.0048342677598399,-0.215224236379592,
-0.282606303775339));
#34387=CARTESIAN_POINT('Ctrl Pts',(0.178243453420992,-0.120723292368367,
-0.271488520738266));
#34388=CARTESIAN_POINT('Ctrl Pts',(0.198065535958834,0.0843497808613357,
-0.260370737701194));
#34389=CARTESIAN_POINT('Ctrl Pts',(0.0364766603006594,0.212165726319023,
-0.249252954664121));
#34390=CARTESIAN_POINT('Ctrl Pts',(-0.158521691176445,0.145656153902189,
-0.238135171627049));
#34391=CARTESIAN_POINT('Ctrl Pts',(-0.208327839440892,-0.0542618978602245,
-0.227017388589977));
#34392=CARTESIAN_POINT('Ctrl Pts',(-0.0673236418046539,-0.204480732622019,
-0.215899605552904));
#34393=CARTESIAN_POINT('Ctrl Pts',(0.135343203301208,-0.167412834631532,
-0.204781822515832));
#34394=CARTESIAN_POINT('Ctrl Pts',(0.214047350517508,0.02299077416045,-0.19366403947876));
#34395=CARTESIAN_POINT('Ctrl Pts',(0.096702556716136,0.192336843836647,
-0.182546256441687));
#34396=CARTESIAN_POINT('Ctrl Pts',(-0.109213407738754,0.185518890172223,
-0.171428473404615));
#34397=CARTESIAN_POINT('Ctrl Pts',(-0.215099372575849,0.0087817269518365,
-0.160310690367542));
#34398=CARTESIAN_POINT('Ctrl Pts',(-0.123972724665226,-0.175998935710198,
-0.14919290733047));
#34399=CARTESIAN_POINT('Ctrl Pts',(0.0807020073303874,-0.19957937405314,
-0.138075124293397));
#34400=CARTESIAN_POINT('Ctrl Pts',(0.211461123965574,-0.0403630139483802,
-0.126957341256325));
#34401=CARTESIAN_POINT('Ctrl Pts',(0.148539190344733,0.155823728504327,
-0.115839558219253));
#34402=CARTESIAN_POINT('Ctrl Pts',(-0.0504301466772234,0.209286815815126,
-0.10472177518218));
#34403=CARTESIAN_POINT('Ctrl Pts',(-0.203213034457697,0.0710660764720931,
-0.0936039921451079));
#34404=CARTESIAN_POINT('Ctrl Pts',(-0.169864175210909,-0.132254304990668,
-0.0824862091080356));
#34405=CARTESIAN_POINT('Ctrl Pts',(0.0190539709745751,-0.214423554575135,
-0.0713684260709631));
#34406=CARTESIAN_POINT('Ctrl Pts',(0.190542505233092,-0.100232788555346,
-0.0602506430338908));
#34407=CARTESIAN_POINT('Ctrl Pts',(0.187468297597579,0.105826317542969,
-0.0491328599968185));
#34408=CARTESIAN_POINT('Ctrl Pts',(0.012769791933206,0.21483601903054,-0.0380150769597463));
#34409=CARTESIAN_POINT('Ctrl Pts',(-0.173779083964507,0.127308534023805,
-0.0268972939226738));
#34410=CARTESIAN_POINT('Ctrl Pts',(-0.200857745661268,-0.0772906680786118,
-0.0157795108856014));
#34411=CARTESIAN_POINT('Ctrl Pts',(-0.0967082013949975,-0.165782769921495,
-0.00836765552755316));
#34412=CARTESIAN_POINT('Ctrl Pts',(-0.03742098496515,-0.178230609497964,
-0.00466172784852903));
#34413=CARTESIAN_POINT('Ctrl Pts',(-0.0861525859670559,0.175382131162753,
-1.5646));
#34414=CARTESIAN_POINT('Ctrl Pts',(-0.144492275190263,0.146724051472585,
-1.56089407232098));
#34415=CARTESIAN_POINT('Ctrl Pts',(-0.229315762961314,0.0271121196187737,
-1.55348221696293));
#34416=CARTESIAN_POINT('Ctrl Pts',(-0.146925824378568,-0.178426424660404,
-1.54236443392585));
#34417=CARTESIAN_POINT('Ctrl Pts',(0.0702270199492049,-0.219974630838623,
-1.53124665088878));
#34418=CARTESIAN_POINT('Ctrl Pts',(0.222959556485836,-0.0603293268215795,
-1.52012886785171));
#34419=CARTESIAN_POINT('Ctrl Pts',(0.171531815124264,0.15472022586109,-1.50901108481464));
#34420=CARTESIAN_POINT('Ctrl Pts',(-0.0370312919934256,0.227981918373403,
-1.49789330177756));
#34421=CARTESIAN_POINT('Ctrl Pts',(-0.21166273897616,0.0924725114640206,
-1.48677551874049));
#34422=CARTESIAN_POINT('Ctrl Pts',(-0.192436817478659,-0.12775512116758,
-1.47565773570342));
#34423=CARTESIAN_POINT('Ctrl Pts',(0.00304855825315219,-0.230958843137944,
-1.46453995266635));
#34424=CARTESIAN_POINT('Ctrl Pts',(0.195739658996433,-0.122630075289071,
-1.45342216962928));
#34425=CARTESIAN_POINT('Ctrl Pts',(0.209151186357511,0.0980203721270748,
-1.4423043865922));
#34426=CARTESIAN_POINT('Ctrl Pts',(0.0309976873846526,0.228890978396746,
-1.43118660355513));
#34427=CARTESIAN_POINT('Ctrl Pts',(-0.175546722608327,0.150118035003706,
-1.42006882051806));
#34428=CARTESIAN_POINT('Ctrl Pts',(-0.221305623643101,-0.0661505383029409,
-1.40895103748099));
#34429=CARTESIAN_POINT('Ctrl Pts',(-0.0643675673818668,-0.221830684237955,
-1.39783325444391));
#34430=CARTESIAN_POINT('Ctrl Pts',(0.151525588825757,-0.174333169320765,
-1.38671547140684));
#34431=CARTESIAN_POINT('Ctrl Pts',(0.228634389855163,0.0328385665534054,
-1.37559768836977));
#34432=CARTESIAN_POINT('Ctrl Pts',(0.0963337859677596,0.209932971829016,
-1.3644799053327));
#34433=CARTESIAN_POINT('Ctrl Pts',(-0.124200255662681,0.194746889035336,
-1.35336212229563));
#34434=CARTESIAN_POINT('Ctrl Pts',(-0.230977572400255,0.00118943348492363,
-1.34224433925855));
#34435=CARTESIAN_POINT('Ctrl Pts',(-0.126199341218217,-0.193457435632643,
-1.33112655622148));
#34436=CARTESIAN_POINT('Ctrl Pts',(0.0941666072966302,-0.210913972246026,
-1.32000877318441));
#34437=CARTESIAN_POINT('Ctrl Pts',(0.228284061114703,-0.0351914895718038,
-1.30889099014733));
#34438=CARTESIAN_POINT('Ctrl Pts',(0.153312992655439,0.172763363341896,
-1.29777320711026));
#34439=CARTESIAN_POINT('Ctrl Pts',(-0.0620795614515782,0.222481867916951,
-1.28665542407319));
#34440=CARTESIAN_POINT('Ctrl Pts',(-0.22061258856118,0.0684261590905361,
-1.27553764103612));
#34441=CARTESIAN_POINT('Ctrl Pts',(-0.177083501191208,-0.148302013062266,
-1.26441985799905));
#34442=CARTESIAN_POINT('Ctrl Pts',(0.0286388087541587,-0.229198324853811,
-1.25330207496197));
#34443=CARTESIAN_POINT('Ctrl Pts',(0.208130438539744,-0.1001687278149,-1.2421842919249));
#34444=CARTESIAN_POINT('Ctrl Pts',(0.196992527342426,0.120606789400195,
-1.23106650888783));
#34445=CARTESIAN_POINT('Ctrl Pts',(0.00542644174545787,0.230916883768986,
-1.21994872585076));
#34446=CARTESIAN_POINT('Ctrl Pts',(-0.191109796735638,0.129727017504544,
-1.20883094281368));
#34447=CARTESIAN_POINT('Ctrl Pts',(-0.212605934961331,-0.0902816143971185,
-1.19771315977661));
#34448=CARTESIAN_POINT('Ctrl Pts',(-0.0393733632728863,-0.227600069735721,
-1.18659537673954));
#34449=CARTESIAN_POINT('Ctrl Pts',(0.169921815212332,-0.156456480191677,
-1.17547759370246));
#34450=CARTESIAN_POINT('Ctrl Pts',(0.223583258126262,0.0579877587484838,
-1.1643598106654));
#34451=CARTESIAN_POINT('Ctrl Pts',(0.0724617093456121,0.219320209186852,
-1.15324202762832));
#34452=CARTESIAN_POINT('Ctrl Pts',(-0.145028519037734,0.17977425328661,
-1.14212424459125));
#34453=CARTESIAN_POINT('Ctrl Pts',(-0.22968512535792,-0.0244294221862726,
-1.13100646155418));
#34454=CARTESIAN_POINT('Ctrl Pts',(-0.103969955576743,-0.20625785273878,
-1.11988867851711));
#34455=CARTESIAN_POINT('Ctrl Pts',(0.11697273136201,-0.199171869491529,
-1.10877089548003));
#34456=CARTESIAN_POINT('Ctrl Pts',(0.230778479355723,-0.00966162229131927,
-1.09765311244296));
#34457=CARTESIAN_POINT('Ctrl Pts',(0.13321103323257,0.188697838101425,-1.08653532940589));
#34458=CARTESIAN_POINT('Ctrl Pts',(-0.0863662366167158,0.21422634443902,
-1.07541754636882));
#34459=CARTESIAN_POINT('Ctrl Pts',(-0.226839478445307,0.0435419854588804,
-1.06429976333174));
#34460=CARTESIAN_POINT('Ctrl Pts',(-0.159547311451343,-0.167023078907342,
-1.05318198029467));
#34461=CARTESIAN_POINT('Ctrl Pts',(0.0538764399450253,-0.224609400288346,
-1.0420641972576));
#34462=CARTESIAN_POINT('Ctrl Pts',(0.21795401647007,-0.0764728722071082,
-1.03094641422052));
#34463=CARTESIAN_POINT('Ctrl Pts',(0.182404501420134,0.14170621489798,-1.01982863118345));
#34464=CARTESIAN_POINT('Ctrl Pts',(-0.0202118137669104,0.230094624151221,
-1.00871084814638));
#34465=CARTESIAN_POINT('Ctrl Pts',(-0.204315849790256,0.107736191706991,
-0.997593065109308));
#34466=CARTESIAN_POINT('Ctrl Pts',(-0.201284179315163,-0.113299305542715,
-0.986475282072236));
#34467=CARTESIAN_POINT('Ctrl Pts',(-0.0138935511685533,-0.230562405250654,
-0.975357499035163));
#34468=CARTESIAN_POINT('Ctrl Pts',(0.186222372232284,-0.136650216096502,
-0.964239715998091));
#34469=CARTESIAN_POINT('Ctrl Pts',(0.215774654930363,0.0824217918315482,
-0.953121932961018));
#34470=CARTESIAN_POINT('Ctrl Pts',(0.0476959533641147,0.226002543153232,
-0.942004149923947));
#34471=CARTESIAN_POINT('Ctrl Pts',(-0.164068130119753,0.162584446236557,
-0.930886366886873));
#34472=CARTESIAN_POINT('Ctrl Pts',(-0.225559948992936,-0.0497469887464949,
-0.919768583849802));
#34473=CARTESIAN_POINT('Ctrl Pts',(-0.0804582977272316,-0.216514470199744,
-0.908650800812729));
#34474=CARTESIAN_POINT('Ctrl Pts',(0.138336218797355,-0.18497336037357,
-0.897533017775658));
#34475=CARTESIAN_POINT('Ctrl Pts',(0.230426683406532,0.0159874029568902,
-0.886415234738584));
#34476=CARTESIAN_POINT('Ctrl Pts',(0.111466168663688,0.202305083283833,
-0.875297451701513));
#34477=CARTESIAN_POINT('Ctrl Pts',(-0.109587748255086,0.203328745905295,
-0.864179668664439));
#34478=CARTESIAN_POINT('Ctrl Pts',(-0.230268734173445,0.0181208040991509,
-0.853061885627368));
#34479=CARTESIAN_POINT('Ctrl Pts',(-0.140043408622157,-0.183684232258863,
-0.841944102590293));
#34480=CARTESIAN_POINT('Ctrl Pts',(0.0784496075652732,-0.217250345343557,
-0.830826319553223));
#34481=CARTESIAN_POINT('Ctrl Pts',(0.225089545534232,-0.0518338689491085,
-0.819708536516149));
#34482=CARTESIAN_POINT('Ctrl Pts',(0.165566862383964,0.161057963352855,
-0.808590753479078));
#34483=CARTESIAN_POINT('Ctrl Pts',(-0.0456007949411382,0.22643458432796,
-0.797472970442004));
#34484=CARTESIAN_POINT('Ctrl Pts',(-0.215002054862611,0.084416644590361,
-0.786355187404934));
#34485=CARTESIAN_POINT('Ctrl Pts',(-0.187479965584133,-0.134919664925512,
-0.77523740436786));
#34486=CARTESIAN_POINT('Ctrl Pts',(0.0117576115035681,-0.230681191367592,
-0.764119621330788));
#34487=CARTESIAN_POINT('Ctrl Pts',(0.200226229953391,-0.115158631103761,
-0.753001838293715));
#34488=CARTESIAN_POINT('Ctrl Pts',(0.205304881152449,0.105839308642956,
-0.741884055256644));
#34489=CARTESIAN_POINT('Ctrl Pts',(0.0223419583792376,0.229897564960615,
-0.73076627221957));
#34490=CARTESIAN_POINT('Ctrl Pts',(-0.181084272405317,0.143389468813009,
-0.719648489182499));
#34491=CARTESIAN_POINT('Ctrl Pts',(-0.21865291902735,-0.0744510206770842,
-0.708530706145426));
#34492=CARTESIAN_POINT('Ctrl Pts',(-0.0559543395769349,-0.224100792862384,
-0.697412923108353));
#34493=CARTESIAN_POINT('Ctrl Pts',(0.157993591693872,-0.168493556145955,
-0.686295140071281));
#34494=CARTESIAN_POINT('Ctrl Pts',(0.227233011930364,0.0414392539519657,
-0.675177357034209));
#34495=CARTESIAN_POINT('Ctrl Pts',(0.0883465805943492,0.213417279469883,
-0.664059573997136));
#34496=CARTESIAN_POINT('Ctrl Pts',(-0.131457703141354,0.189923473440857,
-0.652941790960065));
#34497=CARTESIAN_POINT('Ctrl Pts',(-0.230858062378427,-0.00752386296517325,
-0.64182400792299));
#34498=CARTESIAN_POINT('Ctrl Pts',(-0.118812336309844,-0.19807998944779,
-0.630706224885921));
#34499=CARTESIAN_POINT('Ctrl Pts',(0.102055248263095,-0.20721191997807,
-0.619588441848847));
#34500=CARTESIAN_POINT('Ctrl Pts',(0.229449022531091,-0.0265555933574688,
-0.608470658811775));
#34501=CARTESIAN_POINT('Ctrl Pts',(0.146687270535163,0.178423367701611,
-0.597352875774702));
#34502=CARTESIAN_POINT('Ctrl Pts',(-0.0704273769121229,0.219981903938297,
-0.58623509273763));
#34503=CARTESIAN_POINT('Ctrl Pts',(-0.223036617907527,0.0600559784818474,
-0.575117309700557));
#34504=CARTESIAN_POINT('Ctrl Pts',(-0.171363542528578,-0.154876046472966,
-0.563999526663486));
#34505=CARTESIAN_POINT('Ctrl Pts',(0.0372637663671585,-0.227954963085198,
-0.552881743626412));
#34506=CARTESIAN_POINT('Ctrl Pts',(0.211760677385933,-0.0922467830988746,
-0.541763960589341));
#34507=CARTESIAN_POINT('Ctrl Pts',(0.192303061568511,0.127951498586056,
-0.530646177552267));
#34508=CARTESIAN_POINT('Ctrl Pts',(-0.00328758223170905,0.230957236912183,
-0.519528394515196));
#34509=CARTESIAN_POINT('Ctrl Pts',(-0.195867084095393,0.122426054608521,
-0.508410611478123));
#34510=CARTESIAN_POINT('Ctrl Pts',(-0.209049220558358,-0.0982368406606357,
-0.497292828441051));
#34511=CARTESIAN_POINT('Ctrl Pts',(-0.0307602909131559,-0.228923257844148,
-0.486175045403978));
#34512=CARTESIAN_POINT('Ctrl Pts',(0.175702413689009,-0.14993570389636,
-0.475057262366906));
#34513=CARTESIAN_POINT('Ctrl Pts',(0.221236852799642,0.0663800304485451,
-0.463939479329834));
#34514=CARTESIAN_POINT('Ctrl Pts',(0.0641374052360248,0.221897378823251,
-0.452821696292761));
#34515=CARTESIAN_POINT('Ctrl Pts',(-0.151706376916133,0.174175855623051,
-0.441703913255688));
#34516=CARTESIAN_POINT('Ctrl Pts',(-0.228600194816059,-0.0330757374687038,
-0.430586130218617));
#34517=CARTESIAN_POINT('Ctrl Pts',(-0.0961159394705803,-0.210032806148765,
-0.419468347181543));
#34518=CARTESIAN_POINT('Ctrl Pts',(0.124402231290949,-0.194617929104401,
-0.408350564144472));
#34519=CARTESIAN_POINT('Ctrl Pts',(0.230978681591128,-0.000949804954544109,
-0.397232781107399));
#34520=CARTESIAN_POINT('Ctrl Pts',(0.125998569784222,0.193588258660883,
-0.386114998070328));
#34521=CARTESIAN_POINT('Ctrl Pts',(-0.094385370940541,0.210816164540436,
-0.374997215033254));
#34522=CARTESIAN_POINT('Ctrl Pts',(-0.228320447848423,0.034954635933263,
-0.363879431996183));
#34523=CARTESIAN_POINT('Ctrl Pts',(-0.153133675619892,-0.172922326118124,
-0.352761648959109));
#34524=CARTESIAN_POINT('Ctrl Pts',(0.062310343442467,-0.2224173432529,-0.341643865922038));
#34525=CARTESIAN_POINT('Ctrl Pts',(0.22068345902505,-0.0681972462121358,
-0.330526082884965));
#34526=CARTESIAN_POINT('Ctrl Pts',(0.176929548933351,0.148485649788263,
-0.319408299847893));
#34527=CARTESIAN_POINT('Ctrl Pts',(-0.0288765767642302,0.229168489974145,
-0.30829051681082));
#34528=CARTESIAN_POINT('Ctrl Pts',(-0.208234247273263,0.0999527475109843,
-0.297172733773748));
#34529=CARTESIAN_POINT('Ctrl Pts',(-0.196867296985244,-0.120811095753957,
-0.286054950736675));
#34530=CARTESIAN_POINT('Ctrl Pts',(-0.00518687244590196,-0.230922389248131,
-0.274937167699603));
#34531=CARTESIAN_POINT('Ctrl Pts',(0.191244280031821,-0.129528679392947,
-0.263819384662531));
#34532=CARTESIAN_POINT('Ctrl Pts',(0.212512157369943,0.090502135153134,
-0.252701601625458));
#34533=CARTESIAN_POINT('Ctrl Pts',(0.0391372165612645,0.227640795768667,
-0.241583818588386));
#34534=CARTESIAN_POINT('Ctrl Pts',(-0.170084040207984,0.156280108753479,
-0.230466035551313));
#34535=CARTESIAN_POINT('Ctrl Pts',(-0.223522978823559,-0.0582196843152984,
-0.219348252514241));
#34536=CARTESIAN_POINT('Ctrl Pts',(-0.0722341334783348,-0.219395269448206,
-0.208230469477168));
#34537=CARTESIAN_POINT('Ctrl Pts',(0.145214946051373,-0.1796236911522,-0.197112686440096));
#34538=CARTESIAN_POINT('Ctrl Pts',(0.229659662987761,0.0246676888676773,
-0.185994903403024));
#34539=CARTESIAN_POINT('Ctrl Pts',(0.103755905091973,0.206365622507627,
-0.174877120365952));
#34540=CARTESIAN_POINT('Ctrl Pts',(-0.117179279978873,0.199050376899346,
-0.163759337328879));
#34541=CARTESIAN_POINT('Ctrl Pts',(-0.230788418054293,0.00942225375522446,
-0.152641554291807));
#34542=CARTESIAN_POINT('Ctrl Pts',(-0.13301512070789,-0.188836050358411,
-0.141523771254734));
#34543=CARTESIAN_POINT('Ctrl Pts',(0.086588298155162,-0.214136412684086,
-0.130405988217662));
#34544=CARTESIAN_POINT('Ctrl Pts',(0.226884800711301,-0.0433070353739192,
-0.11928820518059));
#34545=CARTESIAN_POINT('Ctrl Pts',(0.159373429816203,0.167189291936005,
-0.108170422143517));
#34546=CARTESIAN_POINT('Ctrl Pts',(-0.0541084505942859,0.224551901584748,
-0.0970526391064448));
#34547=CARTESIAN_POINT('Ctrl Pts',(-0.218035107164092,0.0762495360628558,
-0.0859348560693726));
#34548=CARTESIAN_POINT('Ctrl Pts',(-0.182253829063119,-0.141900747845757,
-0.0748170730323));
#34549=CARTESIAN_POINT('Ctrl Pts',(0.0204437407985646,-0.230063306839836,
-0.0636992899952277));
#34550=CARTESIAN_POINT('Ctrl Pts',(0.204440407371902,-0.107543627072653,
-0.0525815069581553));
#34551=CARTESIAN_POINT('Ctrl Pts',(0.201141971358471,0.113545140191613,
-0.041463723921083));
#34552=CARTESIAN_POINT('Ctrl Pts',(0.0137012025830432,0.230505855872065,
-0.0303459408840108));
#34553=CARTESIAN_POINT('Ctrl Pts',(-0.186454285750881,0.136594239305857,
-0.0192281578469384));
#34554=CARTESIAN_POINT('Ctrl Pts',(-0.215508026917975,-0.0829281406198991,
-0.00811037480986591));
#34555=CARTESIAN_POINT('Ctrl Pts',(-0.103761961485765,-0.177874731816565,
-0.000698519451817671));
#34556=CARTESIAN_POINT('Ctrl Pts',(-0.0401504189376247,-0.191230499291126,
0.00300740822720647));
#34557=CARTESIAN_POINT('Ctrl Pts',(-0.195211655640432,0.00014838930625368,
-0.0821869692124233));
#34558=CARTESIAN_POINT('Ctrl Pts',(-0.194905158848201,-0.0430319431973475,
-0.0797303371523822));
#34559=CARTESIAN_POINT('Ctrl Pts',(-0.18078209130478,-0.0863940405347896,
-0.0772737050923411));
#34560=CARTESIAN_POINT('Ctrl Pts',(-0.154434447103001,-0.120236127026668,
-0.0748170730323));
#34561=CARTESIAN_POINT('Ctrl Pts',(-0.114687972442558,-0.17128826751045,
-0.0711111453532758));
#34562=CARTESIAN_POINT('Ctrl Pts',(-0.0471221158219972,-0.200675787175143,
-0.0674052176742518));
#34563=CARTESIAN_POINT('Ctrl Pts',(0.0173269235838404,-0.194949600379625,
-0.0636992899952276));
#34564=CARTESIAN_POINT('Ctrl Pts',(0.0817759629896761,-0.189223413584108,
-0.0599933623162036));
#34565=CARTESIAN_POINT('Ctrl Pts',(0.143108185180787,-0.148383520328383,
-0.0562874346371796));
#34566=CARTESIAN_POINT('Ctrl Pts',(0.173224556940772,-0.0911154458231427,
-0.0525815069581555));
#34567=CARTESIAN_POINT('Ctrl Pts',(0.203340928700759,-0.0338473713179008,
-0.0488755792791313));
#34568=CARTESIAN_POINT('Ctrl Pts',(0.202241450029616,0.0398488844368553,
-0.0451696516001073));
#34569=CARTESIAN_POINT('Ctrl Pts',(0.170451582564806,0.0961904649276424,
-0.0414637239210832));
#34570=CARTESIAN_POINT('Ctrl Pts',(0.138661715099997,0.152532045418428,
-0.0377577962420592));
#34571=CARTESIAN_POINT('Ctrl Pts',(0.0761814588415184,0.191518950645247,
-0.0340518685630348));
#34572=CARTESIAN_POINT('Ctrl Pts',(0.0115820826566276,0.195360467164288,
-0.0303459408840108));
#34573=CARTESIAN_POINT('Ctrl Pts',(-0.0485325395593545,0.198935289831578,
-0.0268972939226739));
#34574=CARTESIAN_POINT('Ctrl Pts',(-0.110482259223248,0.172075207744509,
-0.0234486469613371));
#34575=CARTESIAN_POINT('Ctrl Pts',(-0.149578925757925,0.126231591330479,
-0.0200000000000002));
#34576=CARTESIAN_POINT('',(-0.0903606778650182,-0.126612599672285,-1.5646));
#34577=CARTESIAN_POINT('Ctrl Pts',(-0.0905548925879826,-0.126791816255572,
-1.5646));
#34578=CARTESIAN_POINT('Ctrl Pts',(-0.0937532001918452,-0.125081815778544,
-1.5646));
#34579=CARTESIAN_POINT('Ctrl Pts',(-0.0968817208862554,-0.123255435291712,
-1.5646));
#34580=CARTESIAN_POINT('Ctrl Pts',(-0.0999333552098715,-0.121314098198218,
-1.5646));
#34581=CARTESIAN_POINT('Ctrl Pts',(-0.107358826195873,-0.116590287697651,
-1.5646));
#34582=CARTESIAN_POINT('Ctrl Pts',(-0.114329742086453,-0.111187533769295,
-1.5646));
#34583=CARTESIAN_POINT('Ctrl Pts',(-0.120819049765463,-0.10520686979309,
-1.5646));
#34584=CARTESIAN_POINT('Ctrl Pts',(-0.123912141625436,-0.102356220081739,
-1.5646));
#34585=CARTESIAN_POINT('Ctrl Pts',(-0.126895620400741,-0.0993734486954757,
-1.5646));
#34586=CARTESIAN_POINT('Ctrl Pts',(-0.129756065809199,-0.0962799395198511,
-1.5646));
#34587=CARTESIAN_POINT('Ctrl Pts',(-0.13505492992586,-0.0905493338187916,
-1.5646));
#34588=CARTESIAN_POINT('Ctrl Pts',(-0.139941342179991,-0.0844312047867337,
-1.5646));
#34589=CARTESIAN_POINT('Ctrl Pts',(-0.144395973511904,-0.0779901114787239,
-1.5646));
#34590=CARTESIAN_POINT('Ctrl Pts',(-0.146717425902047,-0.0746334495372757,
-1.5646));
#34591=CARTESIAN_POINT('Ctrl Pts',(-0.148922318893028,-0.0711875248212428,
-1.5646));
#34592=CARTESIAN_POINT('Ctrl Pts',(-0.151004655746733,-0.0676646554325792,
-1.5646));
#34593=CARTESIAN_POINT('Ctrl Pts',(-0.156939281662135,-0.0576245353946859,
-1.5646));
#34594=CARTESIAN_POINT('Ctrl Pts',(-0.161845187410773,-0.0470244648230485,
-1.5646));
#34595=CARTESIAN_POINT('Ctrl Pts',(-0.165663065915722,-0.0360640028289907,
-1.5646));
#34596=CARTESIAN_POINT('Ctrl Pts',(-0.168575860309324,-0.0277018791505693,
-1.5646));
#34597=CARTESIAN_POINT('Ctrl Pts',(-0.170855019541254,-0.0191286573412821,
-1.5646));
#34598=CARTESIAN_POINT('Ctrl Pts',(-0.172459025338206,-0.0104201269361194,
-1.5646));
#34599=CARTESIAN_POINT('Ctrl Pts',(-0.173099136546176,-0.00694481037062258,
-1.5646));
#34600=CARTESIAN_POINT('Ctrl Pts',(-0.173631215439875,-0.00344800373498262,
-1.5646));
#34601=CARTESIAN_POINT('Ctrl Pts',(-0.174051082244989,5.13592542474017E-5,
-1.5646));
#34602=CARTESIAN_POINT('Ctrl Pts',(-0.174868285791271,0.00686230932149219,
-1.5646));
#34603=CARTESIAN_POINT('Ctrl Pts',(-0.175263381326914,0.0136958974655043,
-1.5646));
#34604=CARTESIAN_POINT('Ctrl Pts',(-0.175222363933104,0.0205158229853707,
-1.5646));
#34605=CARTESIAN_POINT('Ctrl Pts',(-0.175176056838249,0.0282152623845594,
-1.5646));
#34606=CARTESIAN_POINT('Ctrl Pts',(-0.174574248416374,0.035897416489142,
-1.5646));
#34607=CARTESIAN_POINT('Ctrl Pts',(-0.173452468406207,0.0435229784332608,
-1.5646));
#34608=CARTESIAN_POINT('Ctrl Pts',(-0.172769676803301,0.0481644140228602,
-1.5646));
#34609=CARTESIAN_POINT('Ctrl Pts',(-0.171894043795892,0.0527849303693672,
-1.5646));
#34610=CARTESIAN_POINT('Ctrl Pts',(-0.170831789993684,0.0573757738448648,
-1.5646));
#34611=CARTESIAN_POINT('Ctrl Pts',(-0.1700259113612,0.060858616320261,-1.5646));
#34612=CARTESIAN_POINT('Ctrl Pts',(-0.169112472680126,0.0643237115920012,
-1.5646));
#34613=CARTESIAN_POINT('Ctrl Pts',(-0.168098483581223,0.0677542609967512,
-1.5646));
#34614=CARTESIAN_POINT('Ctrl Pts',(-0.164843308212733,0.0787672392771043,
-1.5646));
#34615=CARTESIAN_POINT('Ctrl Pts',(-0.160547607684451,0.0894588682215987,
-1.5646));
#34616=CARTESIAN_POINT('Ctrl Pts',(-0.15532132364043,0.0997061301383391,
-1.5646));
#34617=CARTESIAN_POINT('Ctrl Pts',(-0.152112604778659,0.105997518497027,
-1.5646));
#34618=CARTESIAN_POINT('Ctrl Pts',(-0.14855224829291,0.112121534649242,
-1.5646));
#34619=CARTESIAN_POINT('Ctrl Pts',(-0.144658388961414,0.11804872209353,
-1.5646));
#34620=CARTESIAN_POINT('Ctrl Pts',(-0.141735673513408,0.122497645598941,
-1.5646));
#34621=CARTESIAN_POINT('Ctrl Pts',(-0.138620900433489,0.126840131680051,
-1.5646));
#34622=CARTESIAN_POINT('Ctrl Pts',(-0.135341984423439,0.131036730447831,
-1.5646));
#34623=CARTESIAN_POINT('Ctrl Pts',(-0.127445990316296,0.141142606609001,
-1.5646));
#34624=CARTESIAN_POINT('Ctrl Pts',(-0.118587414130911,0.150430178036819,
-1.5646));
#34625=CARTESIAN_POINT('Ctrl Pts',(-0.108883967809866,0.158736266807026,
-1.5646));
#34626=CARTESIAN_POINT('Ctrl Pts',(-0.101753616243006,0.16483980271763,
-1.5646));
#34627=CARTESIAN_POINT('Ctrl Pts',(-0.0941658812525659,0.170413396666743,
-1.5646));
#34628=CARTESIAN_POINT('Ctrl Pts',(-0.0861525859670562,0.175382131162753,
-1.5646));
#34629=CARTESIAN_POINT('Ctrl Pts',(-0.0905548925879821,-0.126791816255572,
-1.5646));
#34630=CARTESIAN_POINT('Ctrl Pts',(-0.0513799502789448,-0.154465111057779,
-1.56115135303866));
#34631=CARTESIAN_POINT('Ctrl Pts',(0.058718500965293,-0.172171894665568,
-1.5539967783983));
#34632=CARTESIAN_POINT('Ctrl Pts',(0.177489043046939,-0.0480257256248533,
-1.54313627607892));
#34633=CARTESIAN_POINT('Ctrl Pts',(0.136549507894468,0.123166484814191,
-1.53201849304185));
#34634=CARTESIAN_POINT('Ctrl Pts',(-0.0294791068043894,0.181487141263986,
-1.52090071000477));
#34635=CARTESIAN_POINT('Ctrl Pts',(-0.141282213466497,0.0947308729275798,
-1.51195933813737));
#34636=CARTESIAN_POINT('Ctrl Pts',(-0.155414140615138,0.0214996094033827,
-1.50672389394899));
#34637=CARTESIAN_POINT('Ctrl Pts',(-0.155325699155423,7.24743171158018E-5,
-1.50519437743963));
#34638=CARTESIAN_POINT('Origin',(-2.59090492670967E-17,0.,-1.5646));
#34639=CARTESIAN_POINT('',(-0.1954,-2.39295984553393E-17,-1.5646));
#34640=CARTESIAN_POINT('Origin',(0.,0.,-1.5646));
#34641=CARTESIAN_POINT('Origin',(0.,0.,-1.5646));
#34642=CARTESIAN_POINT('',(0.0903606778650233,-0.126612599672282,-1.5646));
#34643=CARTESIAN_POINT('Ctrl Pts',(0.0863567411264547,0.175643900344958,
-1.5646));
#34644=CARTESIAN_POINT('Ctrl Pts',(0.0901946439528806,0.173286650680855,
-1.5646));
#34645=CARTESIAN_POINT('Ctrl Pts',(0.0939395416005596,0.170790644243054,
-1.5646));
#34646=CARTESIAN_POINT('Ctrl Pts',(0.0975828366931286,0.168155421712109,
-1.5646));
#34647=CARTESIAN_POINT('Ctrl Pts',(0.104715013233486,0.162996665191902,
-1.5646));
#34648=CARTESIAN_POINT('Ctrl Pts',(0.111458438257504,0.157304747156973,
-1.5646));
#34649=CARTESIAN_POINT('Ctrl Pts',(0.1177825331303,0.151141812734413,-1.5646));
#34650=CARTESIAN_POINT('Ctrl Pts',(0.120981747064298,0.148024126160198,
-1.5646));
#34651=CARTESIAN_POINT('Ctrl Pts',(0.124075275555252,0.144783758201481,
-1.5646));
#34652=CARTESIAN_POINT('Ctrl Pts',(0.127052171083901,0.14143511287228,-1.5646));
#34653=CARTESIAN_POINT('Ctrl Pts',(0.135245602155662,0.13221849965071,-1.5646));
#34654=CARTESIAN_POINT('Ctrl Pts',(0.142538985144231,0.122207558577474,
-1.5646));
#34655=CARTESIAN_POINT('Ctrl Pts',(0.14884096310014,0.111572087435399,-1.5646));
#34656=CARTESIAN_POINT('Ctrl Pts',(0.150925188381918,0.10805466512878,-1.5646));
#34657=CARTESIAN_POINT('Ctrl Pts',(0.152901721781693,0.104466619547691,
-1.5646));
#34658=CARTESIAN_POINT('Ctrl Pts',(0.154762551889738,0.10082101919008,-1.5646));
#34659=CARTESIAN_POINT('Ctrl Pts',(0.160363871395494,0.0898473293808975,
-1.5646));
#34660=CARTESIAN_POINT('Ctrl Pts',(0.164897520476248,0.0784015119881915,
-1.5646));
#34661=CARTESIAN_POINT('Ctrl Pts',(0.168269747317322,0.0666527387236212,
-1.5646));
#34662=CARTESIAN_POINT('Ctrl Pts',(0.17053544204992,0.0587591019801492,
-1.5646));
#34663=CARTESIAN_POINT('Ctrl Pts',(0.172275892452234,0.0507282896369748,
-1.5646));
#34664=CARTESIAN_POINT('Ctrl Pts',(0.173448974571123,0.0426121852966646,
-1.5646));
#34665=CARTESIAN_POINT('Ctrl Pts',(0.174147941571219,0.0377763012508139,
-1.5646));
#34666=CARTESIAN_POINT('Ctrl Pts',(0.174645109427981,0.0329053571363106,
-1.5646));
#34667=CARTESIAN_POINT('Ctrl Pts',(0.174929105367026,0.0280403292564174,
-1.5646));
#34668=CARTESIAN_POINT('Ctrl Pts',(0.175316356965979,0.021406467406935,
-1.5646));
#34669=CARTESIAN_POINT('Ctrl Pts',(0.175309624504317,0.0147741099420037,
-1.5646));
#34670=CARTESIAN_POINT('Ctrl Pts',(0.174889543081871,0.00817125191888272,
-1.5646));
#34671=CARTESIAN_POINT('Ctrl Pts',(0.174139516163367,-0.00361770372585117,
-1.5646));
#34672=CARTESIAN_POINT('Ctrl Pts',(0.172074020516654,-0.0153146206873486,
-1.5646));
#34673=CARTESIAN_POINT('Ctrl Pts',(0.168782371632102,-0.0267416672032861,
-1.5646));
#34674=CARTESIAN_POINT('Ctrl Pts',(0.167753283826731,-0.0303141728481449,
-1.5646));
#34675=CARTESIAN_POINT('Ctrl Pts',(0.166603407781752,-0.0338609610831103,
-1.5646));
#34676=CARTESIAN_POINT('Ctrl Pts',(0.165341255244092,-0.0373603852761497,
-1.5646));
#34677=CARTESIAN_POINT('Ctrl Pts',(0.161969828859879,-0.0467079488248741,
-1.5646));
#34678=CARTESIAN_POINT('Ctrl Pts',(0.157791865228321,-0.0557463282631995,
-1.5646));
#34679=CARTESIAN_POINT('Ctrl Pts',(0.152867464919401,-0.0643714118638176,
-1.5646));
#34680=CARTESIAN_POINT('Ctrl Pts',(0.150136227847812,-0.0691551716310509,
-1.5646));
#34681=CARTESIAN_POINT('Ctrl Pts',(0.147174947330489,-0.0738115070429787,
-1.5646));
#34682=CARTESIAN_POINT('Ctrl Pts',(0.14399136084734,-0.0783197279550166,
-1.5646));
#34683=CARTESIAN_POINT('Ctrl Pts',(0.142004455648795,-0.0811333495147673,
-1.5646));
#34684=CARTESIAN_POINT('Ctrl Pts',(0.139930928123689,-0.0838892324174092,
-1.5646));
#34685=CARTESIAN_POINT('Ctrl Pts',(0.137772411698158,-0.0865818092317733,
-1.5646));
#34686=CARTESIAN_POINT('Ctrl Pts',(0.135523663129691,-0.0893869434365289,
-1.5646));
#34687=CARTESIAN_POINT('Ctrl Pts',(0.133187545061614,-0.0921171125955211,
-1.5646));
#34688=CARTESIAN_POINT('Ctrl Pts',(0.130770515703773,-0.0947630325834097,
-1.5646));
#34689=CARTESIAN_POINT('Ctrl Pts',(0.123527059508787,-0.102692437936115,
-1.5646));
#34690=CARTESIAN_POINT('Ctrl Pts',(0.115548451594148,-0.109881057155588,
-1.5646));
#34691=CARTESIAN_POINT('Ctrl Pts',(0.10689716230252,-0.116171310827943,
-1.5646));
#34692=CARTESIAN_POINT('Ctrl Pts',(0.101630903118588,-0.120000347755809,
-1.5646));
#34693=CARTESIAN_POINT('Ctrl Pts',(0.0961149067122779,-0.123495713824771,
-1.5646));
#34694=CARTESIAN_POINT('Ctrl Pts',(0.0903606778650246,-0.126612599672281,
-1.5646));
#34695=CARTESIAN_POINT('Origin',(0.,0.,-1.5646));
#34696=CARTESIAN_POINT('Origin',(0.,0.,-1.69400562256037));
#34697=CARTESIAN_POINT('Ctrl Pts',(0.0903606778650232,-0.126612599672282,
-1.5646));
#34698=CARTESIAN_POINT('Ctrl Pts',(0.132477509652,-0.0965547264460079,-1.56089407232098));
#34699=CARTESIAN_POINT('Ctrl Pts',(0.183629629053462,0.00837163889085661,
-1.55348221696293));
#34700=CARTESIAN_POINT('Ctrl Pts',(0.0923230570238932,0.159158029769189,
-1.54236443392586));
#34701=CARTESIAN_POINT('Ctrl Pts',(-0.0836206488085049,0.163699342626539,
-1.53124665088878));
#34702=CARTESIAN_POINT('Ctrl Pts',(-0.153174468253431,0.0620393558697811,
-1.52346038043362));
#34703=CARTESIAN_POINT('Ctrl Pts',(-0.155774899534441,0.00530901775232087,
-1.51938003765748));
#34704=CARTESIAN_POINT('Ctrl Pts',(-0.155739242772632,9.98782012467418E-5,
-1.51900562256037));
#34705=CARTESIAN_POINT('Ctrl Pts',(0.113509973994377,-0.159049193030949,
-1.58760740822721));
#34706=CARTESIAN_POINT('Ctrl Pts',(0.166416620932181,-0.121290861765029,
-1.58390148054818));
#34707=CARTESIAN_POINT('Ctrl Pts',(0.230673285226915,0.0105163499792544,
-1.57648962519013));
#34708=CARTESIAN_POINT('Ctrl Pts',(0.11597509059768,0.199932362693021,-1.56537184215306));
#34709=CARTESIAN_POINT('Ctrl Pts',(-0.105043232254462,0.205637104141601,
-1.55425405911599));
#34710=CARTESIAN_POINT('Ctrl Pts',(-0.229800035323766,0.0232923379007898,
-1.54313627607892));
#34711=CARTESIAN_POINT('Ctrl Pts',(-0.144106605593727,-0.180540291081365,
-1.53201849304185));
#34712=CARTESIAN_POINT('Ctrl Pts',(0.0735901299731223,-0.218932805076657,
-1.52090071000477));
#34713=CARTESIAN_POINT('Ctrl Pts',(0.223877253749246,-0.0568441566047822,
-1.5097829269677));
#34714=CARTESIAN_POINT('Ctrl Pts',(0.169115997122617,0.157331121656424,
-1.49866514393063));
#34715=CARTESIAN_POINT('Ctrl Pts',(-0.0405429768310065,0.227392947574501,
-1.48754736089356));
#34716=CARTESIAN_POINT('Ctrl Pts',(-0.213067006103068,0.0891885853239147,
-1.47642957785648));
#34717=CARTESIAN_POINT('Ctrl Pts',(-0.190440587625236,-0.13070806461951,
-1.46531179481941));
#34718=CARTESIAN_POINT('Ctrl Pts',(0.00661328935441616,-0.23088569648881,
-1.45419401178234));
#34719=CARTESIAN_POINT('Ctrl Pts',(0.197609807773384,-0.119592824631789,
-1.44307622874526));
#34720=CARTESIAN_POINT('Ctrl Pts',(0.207612857862459,0.101237234431652,
-1.43195844570819));
#34721=CARTESIAN_POINT('Ctrl Pts',(0.0274603833141874,0.229342467105821,
-1.42084066267112));
#34722=CARTESIAN_POINT('Ctrl Pts',(-0.177843412717356,0.14738989847531,
-1.40972287963405));
#34723=CARTESIAN_POINT('Ctrl Pts',(-0.220257984554934,-0.0695591802067529,
-1.39860509659698));
#34724=CARTESIAN_POINT('Ctrl Pts',(-0.0609352224241326,-0.222798010068075,
-1.38748731355991));
#34725=CARTESIAN_POINT('Ctrl Pts',(0.154198947593458,-0.171973086531601,
-1.37636953052283));
#34726=CARTESIAN_POINT('Ctrl Pts',(0.228100175195862,0.0363643701443694,
-1.36525174748576));
#34727=CARTESIAN_POINT('Ctrl Pts',(0.093081303520226,0.211395193176495,
-1.35413396444868));
#34728=CARTESIAN_POINT('Ctrl Pts',(-0.127192018150192,0.192806244125044,
-1.34301618141162));
#34729=CARTESIAN_POINT('Ctrl Pts',(-0.230968415323631,-0.00237660618670745,
-1.33189839837454));
#34730=CARTESIAN_POINT('Ctrl Pts',(-0.123197653274959,-0.195382689342334,
-1.32078061533747));
#34731=CARTESIAN_POINT('Ctrl Pts',(0.0974115395374693,-0.209435071331169,
-1.3096628323004));
#34732=CARTESIAN_POINT('Ctrl Pts',(0.228800158988753,-0.0316629809566973,
-1.29854504926333));
#34733=CARTESIAN_POINT('Ctrl Pts',(0.150627555230227,0.175109670534308,
-1.28742726622625));
#34734=CARTESIAN_POINT('Ctrl Pts',(-0.0655069051000644,0.221496958226608,
-1.27630948318918));
#34735=CARTESIAN_POINT('Ctrl Pts',(-0.221642687021708,0.0650121250644202,
-1.26519170015211));
#34736=CARTESIAN_POINT('Ctrl Pts',(-0.174772873101609,-0.151018210632965,
-1.25407391711503));
#34737=CARTESIAN_POINT('Ctrl Pts',(0.0321738272563805,-0.228728883082269,
-1.24295613407796));
#34738=CARTESIAN_POINT('Ctrl Pts',(0.209652075213801,-0.0969436149227984,
-1.23183835104089));
#34739=CARTESIAN_POINT('Ctrl Pts',(0.195107094163994,0.123633648019485,
-1.22072056800382));
#34740=CARTESIAN_POINT('Ctrl Pts',(0.00186083298014342,0.230973146526896,
-1.20960278496674));
#34741=CARTESIAN_POINT('Ctrl Pts',(-0.193089790810889,0.12676115256821,
-1.19848500192967));
#34742=CARTESIAN_POINT('Ctrl Pts',(-0.21118681044866,-0.0935531304037486,
-1.1873672188926));
#34743=CARTESIAN_POINT('Ctrl Pts',(-0.0358549158978023,-0.228180810152399,
-1.17624943585553));
#34744=CARTESIAN_POINT('Ctrl Pts',(0.172316990942207,-0.153814536856734,
-1.16513165281846));
#34745=CARTESIAN_POINT('Ctrl Pts',(0.222661387705244,0.0614325934745175,
-1.15401386978138));
#34746=CARTESIAN_POINT('Ctrl Pts',(0.0690671466145953,0.22041276363757,
-1.14289608674431));
#34747=CARTESIAN_POINT('Ctrl Pts',(-0.147786647226476,0.1775138417628,-1.13177830370724));
#34748=CARTESIAN_POINT('Ctrl Pts',(-0.229280611332588,-0.027972457575022,
-1.12066052067017));
#34749=CARTESIAN_POINT('Ctrl Pts',(-0.100773299315656,-0.207838396983976,
-1.10954273763309));
#34750=CARTESIAN_POINT('Ctrl Pts',(0.120033668273633,-0.197342280306596,
-1.09842495459602));
#34751=CARTESIAN_POINT('Ctrl Pts',(0.23090014255785,-0.00609764566010633,
-1.08730717155895));
#34752=CARTESIAN_POINT('Ctrl Pts',(0.130281989719349,0.190731906797471,
-1.07618938852188));
#34753=CARTESIAN_POINT('Ctrl Pts',(-0.0896632354690507,0.212867473609881,
-1.0650716054848));
#34754=CARTESIAN_POINT('Ctrl Pts',(-0.227484665887432,0.0400347836501573,
-1.05395382244773));
#34755=CARTESIAN_POINT('Ctrl Pts',(-0.156949751401061,-0.169466317157649,
-1.04283603941066));
#34756=CARTESIAN_POINT('Ctrl Pts',(0.0573376063898475,-0.223750879348696,
-1.03171825637359));
#34757=CARTESIAN_POINT('Ctrl Pts',(0.219108659196544,-0.0730989232542078,
-1.02060047333651));
#34758=CARTESIAN_POINT('Ctrl Pts',(0.180195067220354,0.144505345455744,
-1.00948269029944));
#34759=CARTESIAN_POINT('Ctrl Pts',(-0.0237616736179114,0.229755174006392,
-0.99836490726237));
#34760=CARTESIAN_POINT('Ctrl Pts',(-0.205954769664849,0.104569067931823,
-0.987247124225297));
#34761=CARTESIAN_POINT('Ctrl Pts',(-0.199511049882178,-0.116393290574426,
-0.976129341188227));
#34762=CARTESIAN_POINT('Ctrl Pts',(-0.0103324061458603,-0.230749427949602,
-0.965011558151152));
#34763=CARTESIAN_POINT('Ctrl Pts',(0.188309830972563,-0.1337589797917,-0.953893775114082));
#34764=CARTESIAN_POINT('Ctrl Pts',(0.214476495119882,0.0857431639078181,
-0.942775992077007));
#34765=CARTESIAN_POINT('Ctrl Pts',(0.0442011774886412,0.22671196047948,
-0.931658209039936));
#34766=CARTESIAN_POINT('Ctrl Pts',(-0.166558608605968,0.160032143693309,
-0.920540426002863));
#34767=CARTESIAN_POINT('Ctrl Pts',(-0.224765066474341,-0.0532233220366446,
-0.909422642965791));
#34768=CARTESIAN_POINT('Ctrl Pts',(-0.0771060980724411,-0.21773081260096,
-0.898304859928718));
#34769=CARTESIAN_POINT('Ctrl Pts',(0.141175409662247,-0.182815647094357,
-0.887187076891647));
#34770=CARTESIAN_POINT('Ctrl Pts',(0.230152411385913,0.0195428925464229,
-0.876069293854574));
#34771=CARTESIAN_POINT('Ctrl Pts',(0.108329643286355,0.204001827200844,
-0.864951510817501));
#34772=CARTESIAN_POINT('Ctrl Pts',(-0.112713740110191,0.201612672980158,
-0.85383372778043));
#34773=CARTESIAN_POINT('Ctrl Pts',(-0.230521053425755,0.0145636892067859,
-0.842715944743356));
#34774=CARTESIAN_POINT('Ctrl Pts',(-0.137190952586333,-0.185824378498318,
-0.831598161706284));
#34775=CARTESIAN_POINT('Ctrl Pts',(0.0817942350404951,-0.216013333454145,
-0.820480378669212));
#34776=CARTESIAN_POINT('Ctrl Pts',(0.225862953986525,-0.0483526951918151,
-0.80936259563214));
#34777=CARTESIAN_POINT('Ctrl Pts',(0.163060676338395,0.163594843891539,
-0.798244812595066));
#34778=CARTESIAN_POINT('Ctrl Pts',(-0.0490911250986347,0.225703607752251,
-0.787127029557995));
#34779=CARTESIAN_POINT('Ctrl Pts',(-0.216279687572231,0.0810873224338431,
-0.776009246520923));
#34780=CARTESIAN_POINT('Ctrl Pts',(-0.185374699415074,-0.137797960553133,
-0.764891463483849));
#34781=CARTESIAN_POINT('Ctrl Pts',(0.0153175342131884,-0.230472189778852,
-0.753773680446778));
#34782=CARTESIAN_POINT('Ctrl Pts',(0.201980226864861,-0.112053759738131,
-0.742655897409705));
#34783=CARTESIAN_POINT('Ctrl Pts',(0.203646442288396,0.108996255252695,
-0.731538114372633));
#34784=CARTESIAN_POINT('Ctrl Pts',(0.0187900707826508,0.230215095846938,
-0.720420331335561));
#34785=CARTESIAN_POINT('Ctrl Pts',(-0.183276385866645,0.140576753055022,
-0.709302548298488));
#34786=CARTESIAN_POINT('Ctrl Pts',(-0.217477471381767,-0.0778177778995558,
-0.698184765261416));
#34787=CARTESIAN_POINT('Ctrl Pts',(-0.0524879395448804,-0.224937932146103,
-0.687066982224343));
#34788=CARTESIAN_POINT('Ctrl Pts',(0.160576020484737,-0.166034330067962,
-0.675949199187271));
#34789=CARTESIAN_POINT('Ctrl Pts',(0.226566187311492,0.0449424062881105,
-0.664831416150198));
#34790=CARTESIAN_POINT('Ctrl Pts',(0.0850412564367271,0.214755772493999,
-0.653713633113127));
#34791=CARTESIAN_POINT('Ctrl Pts',(-0.134374134826396,0.187871362920188,
-0.642595850076053));
#34792=CARTESIAN_POINT('Ctrl Pts',(-0.230714401562136,-0.0110870206844455,
-0.631478067038982));
#34793=CARTESIAN_POINT('Ctrl Pts',(-0.115740163916463,-0.199890649036972,
-0.620360284001908));
#34794=CARTESIAN_POINT('Ctrl Pts',(0.105242087140735,-0.205611673331291,
-0.609242500964837));
#34795=CARTESIAN_POINT('Ctrl Pts',(0.229831658184759,-0.0230101284628302,
-0.598124717927765));
#34796=CARTESIAN_POINT('Ctrl Pts',(0.143915241689072,0.180666710617666,
-0.587006934890691));
#34797=CARTESIAN_POINT('Ctrl Pts',(-0.0738151307822532,0.218868416139539,
-0.575889151853619));
#34798=CARTESIAN_POINT('Ctrl Pts',(-0.223937206279105,0.056605518809929,
-0.564771368816547));
#34799=CARTESIAN_POINT('Ctrl Pts',(-0.168952104083443,-0.157503154386219,
-0.553653585779474));
#34800=CARTESIAN_POINT('Ctrl Pts',(0.0407785618778789,-0.227352514846447,
-0.542535802742403));
#34801=CARTESIAN_POINT('Ctrl Pts',(0.213159580247783,-0.08896656936412,
-0.531418019705329));
#34802=CARTESIAN_POINT('Ctrl Pts',(0.190304797344661,0.130905084788328,
-0.520300236668258));
#34803=CARTESIAN_POINT('Ctrl Pts',(-0.00685277576144637,0.230878965218131,
-0.509182453631185));
#34804=CARTESIAN_POINT('Ctrl Pts',(-0.197733796975422,0.119387615142923,
-0.498064670594113));
#34805=CARTESIAN_POINT('Ctrl Pts',(-0.207507704700154,-0.101452499259039,
-0.48694688755704));
#34806=CARTESIAN_POINT('Ctrl Pts',(-0.027222441965051,-0.229370869487148,
-0.475829104519968));
#34807=CARTESIAN_POINT('Ctrl Pts',(0.177996231051109,-0.147205294902844,
-0.464711321482895));
#34808=CARTESIAN_POINT('Ctrl Pts',(0.220185699597794,0.0697876408002185,
-0.453593538445824));
#34809=CARTESIAN_POINT('Ctrl Pts',(0.0607040471943301,0.222861113184999,
-0.44247575540875));
#34810=CARTESIAN_POINT('Ctrl Pts',(-0.154377279785012,0.171813016392891,
-0.431357972371679));
#34811=CARTESIAN_POINT('Ctrl Pts',(-0.228062325714473,-0.0366009932313942,
-0.420240189334605));
#34812=CARTESIAN_POINT('Ctrl Pts',(-0.0928619401316778,-0.211491648040283,
-0.409122406297534));
#34813=CARTESIAN_POINT('Ctrl Pts',(0.127391977965817,-0.19267418370366,
-0.398004623260461));
#34814=CARTESIAN_POINT('Ctrl Pts',(0.230965825361851,0.00261622450151,-0.386886840223389));
#34815=CARTESIAN_POINT('Ctrl Pts',(0.122994885849355,0.195510396579458,
-0.375769057186316));
#34816=CARTESIAN_POINT('Ctrl Pts',(-0.0976287670138966,0.209333898276729,
-0.364651274149244));
#34817=CARTESIAN_POINT('Ctrl Pts',(-0.228832884833302,0.0314255936116178,
-0.353533491112171));
#34818=CARTESIAN_POINT('Ctrl Pts',(-0.150445805414977,-0.175265845927362,
-0.3424157080751));
#34819=CARTESIAN_POINT('Ctrl Pts',(0.0657366634319771,-0.221428878424336,
-0.331297925038026));
#34820=CARTESIAN_POINT('Ctrl Pts',(0.221710015017261,-0.0647821453049757,
-0.320180142000955));
#34821=CARTESIAN_POINT('Ctrl Pts',(0.17461610416282,0.151199448687295,-0.309062358963882));
#34822=CARTESIAN_POINT('Ctrl Pts',(-0.0324111063717073,0.22869538106904,
-0.29794457592681));
#34823=CARTESIAN_POINT('Ctrl Pts',(-0.209752537145294,0.096726057648452,
-0.286826792889737));
#34824=CARTESIAN_POINT('Ctrl Pts',(-0.194978724715305,-0.123835996553786,
-0.275709009852665));
#34825=CARTESIAN_POINT('Ctrl Pts',(-0.00162120698158336,-0.230974953063417,
-0.264591226815592));
#34826=CARTESIAN_POINT('Ctrl Pts',(0.193221195612131,-0.126560761412732,
-0.253473443778521));
#34827=CARTESIAN_POINT('Ctrl Pts',(0.211089640462245,0.0937721762032856,
-0.242355660741447));
#34828=CARTESIAN_POINT('Ctrl Pts',(0.0356181668760191,0.228217887376357,
-0.231237877704376));
#34829=CARTESIAN_POINT('Ctrl Pts',(-0.172476470490578,0.153635678633855,
-0.220120094667302));
#34830=CARTESIAN_POINT('Ctrl Pts',(-0.222597541227211,-0.0616635544778054,
-0.209002311630231));
#34831=CARTESIAN_POINT('Ctrl Pts',(-0.0688384273015429,-0.220484313605681,
-0.197884528593158));
#34832=CARTESIAN_POINT('Ctrl Pts',(0.147970705227284,-0.177360396550321,
-0.186766745556086));
#34833=CARTESIAN_POINT('Ctrl Pts',(0.22925151616086,0.0282102591823235,
-0.175648962519013));
#34834=CARTESIAN_POINT('Ctrl Pts',(0.100557529478573,0.207942932307904,
-0.164531179481941));
#34835=CARTESIAN_POINT('Ctrl Pts',(-0.120238162331385,0.197217455511372,
-0.153413396444869));
#34836=CARTESIAN_POINT('Ctrl Pts',(-0.23090667834121,0.00585845278655507,
-0.142295613407796));
#34837=CARTESIAN_POINT('Ctrl Pts',(-0.130083407741252,-0.19086765014593,
-0.131177830370724));
#34838=CARTESIAN_POINT('Ctrl Pts',(0.0898828181189855,-0.212773035377908,
-0.120060047333651));
#34839=CARTESIAN_POINT('Ctrl Pts',(0.227528380768991,-0.0398012345171181,
-0.108942264296579));
#34840=CARTESIAN_POINT('Ctrl Pts',(0.156769469656559,0.16963377101867,-0.0978244812595063));
#34841=CARTESIAN_POINT('Ctrl Pts',(-0.0575613644483651,0.223682296329051,
-0.086706698222434));
#34842=CARTESIAN_POINT('Ctrl Pts',(-0.219200259963039,0.0728886583195608,
-0.0755889151853618));
#34843=CARTESIAN_POINT('Ctrl Pts',(-0.18001480464987,-0.144724771019191,
-0.0644711321482894));
#34844=CARTESIAN_POINT('Ctrl Pts',(0.023942282457509,-0.229668165736859,
-0.0533533491112173));
#34845=CARTESIAN_POINT('Ctrl Pts',(0.206174498061778,-0.104476062522128,
-0.0422355660741447));
#34846=CARTESIAN_POINT('Ctrl Pts',(0.199165675931825,0.11684944015648,-0.0311177830370723));
#34847=CARTESIAN_POINT('Ctrl Pts',(0.0734746804820682,0.192373169122532,
-0.0237059276790242));
#34848=CARTESIAN_POINT('Ctrl Pts',(0.00853826423429785,0.19521336543348,
-0.02));
#34849=CARTESIAN_POINT('Ctrl Pts',(0.105793541951259,-0.148236995244726,
-1.57993827215147));
#34850=CARTESIAN_POINT('Ctrl Pts',(0.155103583838787,-0.113045483325355,
-1.57623234447245));
#34851=CARTESIAN_POINT('Ctrl Pts',(0.214992066502431,0.00980144628312182,
-1.5688204891144));
#34852=CARTESIAN_POINT('Ctrl Pts',(0.108091079406417,0.186340918385077,
-1.55770270607733));
#34853=CARTESIAN_POINT('Ctrl Pts',(-0.0979023711058095,0.191657850303247,
-1.54658492304025));
#34854=CARTESIAN_POINT('Ctrl Pts',(-0.214178180312418,0.0217089198432209,
-1.53546714000318));
#34855=CARTESIAN_POINT('Ctrl Pts',(-0.134310208062321,-0.168267123903623,
-1.52434935696611));
#34856=CARTESIAN_POINT('Ctrl Pts',(0.06858745737089,-0.204049706676274,
-1.51323157392904));
#34857=CARTESIAN_POINT('Ctrl Pts',(0.208658030682192,-0.0529798788144361,
-1.50211379089197));
#34858=CARTESIAN_POINT('Ctrl Pts',(0.157619455864793,0.146635718725669,
-1.49099600785489));
#34859=CARTESIAN_POINT('Ctrl Pts',(-0.0377868566899024,0.211934726897524,
-1.47987822481782));
#34860=CARTESIAN_POINT('Ctrl Pts',(-0.198582665957713,0.0831255264273637,
-1.46876044178075));
#34861=CARTESIAN_POINT('Ctrl Pts',(-0.177494396194213,-0.121822502737751,
-1.45764265874368));
#34862=CARTESIAN_POINT('Ctrl Pts',(0.00616371654518196,-0.215190038001811,
-1.4465248757066));
#34863=CARTESIAN_POINT('Ctrl Pts',(0.184176251240171,-0.111462879115622,
-1.43540709266953));
#34864=CARTESIAN_POINT('Ctrl Pts',(0.193499291868227,0.0943551058200843,
-1.42428930963246));
#34865=CARTESIAN_POINT('Ctrl Pts',(0.0255936206477411,0.213751717678719,
-1.41317152659539));
#34866=CARTESIAN_POINT('Ctrl Pts',(-0.165753579901275,0.137370301999293,
-1.40205374355831));
#34867=CARTESIAN_POINT('Ctrl Pts',(-0.2052848001733,-0.0648305324223128,
-1.39093596052124));
#34868=CARTESIAN_POINT('Ctrl Pts',(-0.056792833113996,-0.207652154214761,
-1.37981817748417));
#34869=CARTESIAN_POINT('Ctrl Pts',(0.143716470518058,-0.160282319731389,
-1.3687003944471));
#34870=CARTESIAN_POINT('Ctrl Pts',(0.212593877035584,0.0338923125697315,
-1.35758261141002));
#34871=CARTESIAN_POINT('Ctrl Pts',(0.0867536168172552,0.19702450322753,
-1.34646482837295));
#34872=CARTESIAN_POINT('Ctrl Pts',(-0.118545477851173,0.179699234864752,
-1.33534704533588));
#34873=CARTESIAN_POINT('Ctrl Pts',(-0.215267133592743,-0.00221504399540788,
-1.32422926229881));
#34874=CARTESIAN_POINT('Ctrl Pts',(-0.114822650745093,-0.18210053279117,
-1.31311147926173));
#34875=CARTESIAN_POINT('Ctrl Pts',(0.0907894824740647,-0.195197630879878,
-1.30199369622466));
#34876=CARTESIAN_POINT('Ctrl Pts',(0.213246275782165,-0.0295105248135298,
-1.29087591318759));
#34877=CARTESIAN_POINT('Ctrl Pts',(0.140387862163143,0.163205678090104,
-1.27975813015052));
#34878=CARTESIAN_POINT('Ctrl Pts',(-0.0610537318345626,0.206439548152691,
-1.26864034711344));
#34879=CARTESIAN_POINT('Ctrl Pts',(-0.206575370273473,0.0605925870504019,
-1.25752256407637));
#34880=CARTESIAN_POINT('Ctrl Pts',(-0.162891776218123,-0.140751960728968,
-1.2464047810393));
#34881=CARTESIAN_POINT('Ctrl Pts',(0.0299866436737017,-0.213179845226881,
-1.23528699800223));
#34882=CARTESIAN_POINT('Ctrl Pts',(0.195399882792665,-0.0903533674736788,
-1.22416921496516));
#34883=CARTESIAN_POINT('Ctrl Pts',(0.181843672631351,0.115229006474661,
-1.21305143192808));
#34884=CARTESIAN_POINT('Ctrl Pts',(0.00173433316052722,0.215271543167809,
-1.20193364889101));
#34885=CARTESIAN_POINT('Ctrl Pts',(-0.179963505986915,0.118143902602595,
-1.19081586585394));
#34886=CARTESIAN_POINT('Ctrl Pts',(-0.196830286401612,-0.0871933688094308,
-1.17969808281686));
#34887=CARTESIAN_POINT('Ctrl Pts',(-0.0334174911306108,-0.212669030410719,
-1.16858029977979));
#34888=CARTESIAN_POINT('Ctrl Pts',(0.160602845447415,-0.143358192104532,
-1.15746251674272));
#34889=CARTESIAN_POINT('Ctrl Pts',(0.207524819469055,0.057256392775167,
-1.14634473370565));
#34890=CARTESIAN_POINT('Ctrl Pts',(0.06437194737783,0.205429057341158,-1.13522695066858));
#34891=CARTESIAN_POINT('Ctrl Pts',(-0.13774007968643,0.165446413249924,
-1.1241091676315));
#34892=CARTESIAN_POINT('Ctrl Pts',(-0.213694066874035,-0.0260708839920053,
-1.11299138459443));
#34893=CARTESIAN_POINT('Ctrl Pts',(-0.0939227091114099,-0.193709498792555,
-1.10187360155736));
#34894=CARTESIAN_POINT('Ctrl Pts',(0.111873754113442,-0.183926910347166,
-1.09075581852029));
#34895=CARTESIAN_POINT('Ctrl Pts',(0.215203502024021,-0.00568312641828513,
-1.07963803548321));
#34896=CARTESIAN_POINT('Ctrl Pts',(0.12142539249943,0.177765911427496,-1.06852025244614));
#34897=CARTESIAN_POINT('Ctrl Pts',(-0.0835679097552307,0.19839669772562,
-1.05740246940907));
#34898=CARTESIAN_POINT('Ctrl Pts',(-0.212020210180141,0.0373132105889854,
-1.04628468637199));
#34899=CARTESIAN_POINT('Ctrl Pts',(-0.146280274100937,-0.15794596106974,
-1.03516690333492));
#34900=CARTESIAN_POINT('Ctrl Pts',(0.0534397837787334,-0.208540247240122,
-1.02404912029785));
#34901=CARTESIAN_POINT('Ctrl Pts',(0.204213606195892,-0.0681296429886322,
-1.01293133726078));
#34902=CARTESIAN_POINT('Ctrl Pts',(0.167945368433709,0.134681841504173,
-1.00181355422371));
#34903=CARTESIAN_POINT('Ctrl Pts',(-0.0221463500190146,0.214136368676889,
-0.990695771186635));
#34904=CARTESIAN_POINT('Ctrl Pts',(-0.191953920857029,0.0974604405741237,
-0.979577988149561));
#34905=CARTESIAN_POINT('Ctrl Pts',(-0.185948246508236,-0.108480850060283,
-0.968460205112491));
#34906=CARTESIAN_POINT('Ctrl Pts',(-0.0096300069904304,-0.215063033026724,
-0.957342422075416));
#34907=CARTESIAN_POINT('Ctrl Pts',(0.175508488829512,-0.124666016051169,
-0.946224639038346));
#34908=CARTESIAN_POINT('Ctrl Pts',(0.199896337613012,0.0799143254879507,
-0.935106856001272));
#34909=CARTESIAN_POINT('Ctrl Pts',(0.0411963720930036,0.211300033449274,
-0.923989072964201));
#34910=CARTESIAN_POINT('Ctrl Pts',(-0.155235919160475,0.149153124713134,
-0.912871289927127));
#34911=CARTESIAN_POINT('Ctrl Pts',(-0.209485489710434,-0.0496051893461636,
-0.901753506890056));
#34912=CARTESIAN_POINT('Ctrl Pts',(-0.0718644092150764,-0.202929425903335,
-0.890635723852983));
#34913=CARTESIAN_POINT('Ctrl Pts',(0.131578275450305,-0.170387800733541,
-0.879517940815911));
#34914=CARTESIAN_POINT('Ctrl Pts',(0.214506601775322,0.0182143625771726,
-0.868400157778838));
#34915=CARTESIAN_POINT('Ctrl Pts',(0.100965371220572,0.190133739834837,
-0.857282374741766));
#34916=CARTESIAN_POINT('Ctrl Pts',(-0.105051436214949,0.187907000823454,
-0.846164591704694));
#34917=CARTESIAN_POINT('Ctrl Pts',(-0.214850183451316,0.0135736465338231,
-0.835046808667621));
#34918=CARTESIAN_POINT('Ctrl Pts',(-0.12786468260925,-0.173191997940219,
-0.82392902563055));
#34919=CARTESIAN_POINT('Ctrl Pts',(0.0762338456403528,-0.201328701352221,
-0.812811242593475));
#34920=CARTESIAN_POINT('Ctrl Pts',(0.210508742597301,-0.0450656687445377,
-0.801693459556405));
#34921=CARTESIAN_POINT('Ctrl Pts',(0.151975777068376,0.152473631798264,
-0.79057567651933));
#34922=CARTESIAN_POINT('Ctrl Pts',(-0.0457539000300912,0.210360228753739,
-0.77945789348226));
#34923=CARTESIAN_POINT('Ctrl Pts',(-0.201576948661017,0.0755749891022346,
-0.768340110445186));
#34924=CARTESIAN_POINT('Ctrl Pts',(-0.172772888136174,-0.128430426046067,
-0.757222327408115));
#34925=CARTESIAN_POINT('Ctrl Pts',(0.0142762449972293,-0.214804641565465,
-0.746104544371042));
#34926=CARTESIAN_POINT('Ctrl Pts',(0.188249568317327,-0.104436321448188,
-0.73498676133397));
#34927=CARTESIAN_POINT('Ctrl Pts',(0.189802514063912,0.101586666764432,
-0.723868978296898));
#34928=CARTESIAN_POINT('Ctrl Pts',(0.0175127177961463,0.214565024933426,
-0.712751195259824));
#34929=CARTESIAN_POINT('Ctrl Pts',(-0.170817218386628,0.131020315645873,
-0.701633412222753));
#34930=CARTESIAN_POINT('Ctrl Pts',(-0.202693306873811,-0.0725277088970024,
-0.69051562918568));
#34931=CARTESIAN_POINT('Ctrl Pts',(-0.0489197983117454,-0.209646603937262,
-0.679397846148608));
#34932=CARTESIAN_POINT('Ctrl Pts',(0.149660028645235,-0.154747281188384,
-0.668280063111535));
#34933=CARTESIAN_POINT('Ctrl Pts',(0.211164169972081,0.041887212001893,
-0.657162280074463));
#34934=CARTESIAN_POINT('Ctrl Pts',(0.0792601338352194,0.20015662965216,
-0.646044497037391));
#34935=CARTESIAN_POINT('Ctrl Pts',(-0.125239352716482,0.175099827928087,
-0.634926714000318));
#34936=CARTESIAN_POINT('Ctrl Pts',(-0.215030387740486,-0.0103333226730591,
-0.623808930963246));
#34937=CARTESIAN_POINT('Ctrl Pts',(-0.107872123090684,-0.18630204043219,
-0.612691147926174));
#34938=CARTESIAN_POINT('Ctrl Pts',(0.0980877077948493,-0.191634148284802,
-0.6015733648891));
#34939=CARTESIAN_POINT('Ctrl Pts',(0.214207653444632,-0.0214458950625499,
-0.590455581852029));
#34940=CARTESIAN_POINT('Ctrl Pts',(0.134131853116384,0.168384949413105,
-0.579337798814955));
#34941=CARTESIAN_POINT('Ctrl Pts',(-0.0687971625774212,0.203989694912721,
-0.568220015777885));
#34942=CARTESIAN_POINT('Ctrl Pts',(-0.208713907626388,0.0527574636673564,
-0.557102232740811));
#34943=CARTESIAN_POINT('Ctrl Pts',(-0.157466704309091,-0.146796056634102,
-0.545984449703739));
#34944=CARTESIAN_POINT('Ctrl Pts',(0.0380064266154546,-0.211897042794876,
-0.534866666666667));
#34945=CARTESIAN_POINT('Ctrl Pts',(0.198668946892488,-0.0829186031594792,
-0.523748883629593));
#34946=CARTESIAN_POINT('Ctrl Pts',(0.177367836965635,0.122006129433817,
-0.512631100592523));
#34947=CARTESIAN_POINT('Ctrl Pts',(-0.00638692261560318,0.215183764324336,
-0.501513317555449));
#34948=CARTESIAN_POINT('Ctrl Pts',(-0.184291811630027,0.111271619811218,
-0.490395534518377));
#34949=CARTESIAN_POINT('Ctrl Pts',(-0.193401287040138,-0.09455573689897,
-0.479277751481305));
#34950=CARTESIAN_POINT('Ctrl Pts',(-0.0253718546018513,-0.213778189260156,
-0.468159968444233));
#34951=CARTESIAN_POINT('Ctrl Pts',(0.165896009612375,-0.137198247816732,
-0.457042185407159));
#34952=CARTESIAN_POINT('Ctrl Pts',(0.205217429162836,0.065043462216308,
-0.445924402370089));
#34953=CARTESIAN_POINT('Ctrl Pts',(0.0565773732252167,0.207710967568448,
-0.434806619333014));
#34954=CARTESIAN_POINT('Ctrl Pts',(-0.143882679649508,0.160133131194568,
-0.423688836295944));
#34955=CARTESIAN_POINT('Ctrl Pts',(-0.212558600569946,-0.0341128499692469,
-0.41257105325887));
#34956=CARTESIAN_POINT('Ctrl Pts',(-0.0865491657982631,-0.197114401069274,
-0.401453270221798));
#34957=CARTESIAN_POINT('Ctrl Pts',(0.118731844356234,-0.179576151938748,
-0.390335487184726));
#34958=CARTESIAN_POINT('Ctrl Pts',(0.215264719697113,0.00243837300648307,
-0.379217704147653));
#34959=CARTESIAN_POINT('Ctrl Pts',(0.114633667491973,0.182219558463301,
-0.368099921110581));
#34960=CARTESIAN_POINT('Ctrl Pts',(-0.0909919427806939,0.19510333559108,
-0.356982138073508));
#34961=CARTESIAN_POINT('Ctrl Pts',(-0.213276776916879,0.0292892751103837,
-0.345864355036436));
#34962=CARTESIAN_POINT('Ctrl Pts',(-0.140218467738779,-0.163351236646902,
-0.334746571999364));
#34963=CARTESIAN_POINT('Ctrl Pts',(0.0612678711464706,-0.206376096429779,
-0.323628788962291));
#34964=CARTESIAN_POINT('Ctrl Pts',(0.206638121297647,-0.0603782413636525,
-0.312511005925219));
#34965=CARTESIAN_POINT('Ctrl Pts',(0.162745664464955,0.140920878182027,
-0.301393222888146));
#34966=CARTESIAN_POINT('Ctrl Pts',(-0.0302077925045763,0.213148620687599,
-0.290275439851075));
#34967=CARTESIAN_POINT('Ctrl Pts',(-0.195493515300804,0.0901505997888629,
-0.279157656814001));
#34968=CARTESIAN_POINT('Ctrl Pts',(-0.181724029764938,-0.115417599312797,
-0.26803987377693));
#34969=CARTESIAN_POINT('Ctrl Pts',(-0.0015109969880378,-0.215273226895595,
-0.256922090739857));
#34970=CARTESIAN_POINT('Ctrl Pts',(0.180085977861972,-0.117957134080256,
-0.245804307702785));
#34971=CARTESIAN_POINT('Ctrl Pts',(0.196739722051428,0.08739752382918,-0.234686524665712));
#34972=CARTESIAN_POINT('Ctrl Pts',(0.0331968363574083,0.212703587117149,
-0.22356874162864));
#34973=CARTESIAN_POINT('Ctrl Pts',(-0.160751483542354,0.143191492701478,
-0.212450958591567));
#34974=CARTESIAN_POINT('Ctrl Pts',(-0.207465313288104,-0.0574716530005959,
-0.201333175554495));
#34975=CARTESIAN_POINT('Ctrl Pts',(-0.0641587764520602,-0.205495743327301,
-0.190215392517423));
#34976=CARTESIAN_POINT('Ctrl Pts',(0.137911625385409,-0.165303399275447,
-0.17909760948035));
#34977=CARTESIAN_POINT('Ctrl Pts',(0.213666949598236,0.02629251979574,-0.167979826443278));
#34978=CARTESIAN_POINT('Ctrl Pts',(0.0937216073534937,0.19380692778305,
-0.156862043406205));
#34979=CARTESIAN_POINT('Ctrl Pts',(-0.112064346621891,0.183810571167925,
-0.145744260369133));
#34980=CARTESIAN_POINT('Ctrl Pts',(-0.215209593503446,0.00546019392687473,
-0.134626477332061));
#34981=CARTESIAN_POINT('Ctrl Pts',(-0.121240310166211,-0.177892426914413,
-0.123508694294988));
#34982=CARTESIAN_POINT('Ctrl Pts',(0.0837725651301739,-0.198308679424633,
-0.112390911257916));
#34983=CARTESIAN_POINT('Ctrl Pts',(0.212060953314804,-0.0370955381754129,
-0.101273128220843));
#34984=CARTESIAN_POINT('Ctrl Pts',(0.146112247947562,0.158102031381867,
-0.090155345183771));
#34985=CARTESIAN_POINT('Ctrl Pts',(-0.0536483307171008,0.208476326508661,
-0.0790375621466985));
#34986=CARTESIAN_POINT('Ctrl Pts',(-0.204298979922905,0.0679336719087199,
-0.0679197791096263));
#34987=CARTESIAN_POINT('Ctrl Pts',(-0.167777360150897,-0.134886350471401,
-0.0568019960725539));
#34988=CARTESIAN_POINT('Ctrl Pts',(0.0223146810314913,-0.214055275247924,
-0.0456842130354818));
#34989=CARTESIAN_POINT('Ctrl Pts',(0.192158712071056,-0.0973737576918526,
-0.0345664299984093));
#34990=CARTESIAN_POINT('Ctrl Pts',(0.185626351152085,0.108905990497259,
-0.0234486469613368));
#34991=CARTESIAN_POINT('Ctrl Pts',(0.0684798561606579,0.179295600392521,
-0.0160367916032887));
#34992=CARTESIAN_POINT('Ctrl Pts',(0.0079578312255345,0.181942719557458,
-0.0123308639242645));
#34993=CARTESIAN_POINT('Ctrl Pts',(0.098077109908141,-0.137424797458504,
-1.57226913607574));
#34994=CARTESIAN_POINT('Ctrl Pts',(0.143790546745394,-0.104800104885681,
-1.56856320839671));
#34995=CARTESIAN_POINT('Ctrl Pts',(0.199310847777946,0.00908654258698918,
-1.56115135303866));
#34996=CARTESIAN_POINT('Ctrl Pts',(0.100207068215156,0.172749474077133,
-1.55003357000159));
#34997=CARTESIAN_POINT('Ctrl Pts',(-0.0907615099571574,0.177678596464893,
-1.53891578696452));
#34998=CARTESIAN_POINT('Ctrl Pts',(-0.19855632530107,0.0201255017856523,
-1.52779800392744));
#34999=CARTESIAN_POINT('Ctrl Pts',(-0.124513810530915,-0.155993956725882,
-1.51668022089038));
#35000=CARTESIAN_POINT('Ctrl Pts',(0.0635847847686578,-0.18916660827589,
-1.5055624378533));
#35001=CARTESIAN_POINT('Ctrl Pts',(0.193438807615137,-0.0491156010240898,
-1.49444465481623));
#35002=CARTESIAN_POINT('Ctrl Pts',(0.146122914606969,0.135940315794915,
-1.48332687177916));
#35003=CARTESIAN_POINT('Ctrl Pts',(-0.0350307365487982,0.196476506220547,
-1.47220908874208));
#35004=CARTESIAN_POINT('Ctrl Pts',(-0.184098325812358,0.0770624675308122,
-1.46109130570501));
#35005=CARTESIAN_POINT('Ctrl Pts',(-0.16454820476319,-0.112936940855992,
-1.44997352266794));
#35006=CARTESIAN_POINT('Ctrl Pts',(0.00571414373594752,-0.199494379514811,
-1.43885573963087));
#35007=CARTESIAN_POINT('Ctrl Pts',(0.170742694706959,-0.103332933599455,
-1.42773795659379));
#35008=CARTESIAN_POINT('Ctrl Pts',(0.179385725873994,0.0874729772085164,
-1.41662017355672));
#35009=CARTESIAN_POINT('Ctrl Pts',(0.0237268579812951,0.198160968251618,
-1.40550239051965));
#35010=CARTESIAN_POINT('Ctrl Pts',(-0.153663747085195,0.127350705523275,
-1.39438460748258));
#35011=CARTESIAN_POINT('Ctrl Pts',(-0.190311615791665,-0.0601018846378727,
-1.38326682444551));
#35012=CARTESIAN_POINT('Ctrl Pts',(-0.0526504438038595,-0.192506298361447,
-1.37214904140843));
#35013=CARTESIAN_POINT('Ctrl Pts',(0.133233993442659,-0.148591552931176,
-1.36103125837136));
#35014=CARTESIAN_POINT('Ctrl Pts',(0.197087578875306,0.0314202549950935,
-1.34991347533429));
#35015=CARTESIAN_POINT('Ctrl Pts',(0.0804259301142846,0.182653813278565,
-1.33879569229721));
#35016=CARTESIAN_POINT('Ctrl Pts',(-0.109898937552154,0.16659222560446,
-1.32767790926015));
#35017=CARTESIAN_POINT('Ctrl Pts',(-0.199565851861855,-0.00205348180410804,
-1.31656012622307));
#35018=CARTESIAN_POINT('Ctrl Pts',(-0.106447648215227,-0.168818376240007,
-1.305442343186));
#35019=CARTESIAN_POINT('Ctrl Pts',(0.0841674254106597,-0.180960190428586,
-1.29432456014892));
#35020=CARTESIAN_POINT('Ctrl Pts',(0.197692392575578,-0.0273580686703621,
-1.28320677711186));
#35021=CARTESIAN_POINT('Ctrl Pts',(0.130148169096058,0.151301685645901,
-1.27208899407478));
#35022=CARTESIAN_POINT('Ctrl Pts',(-0.0566005585690605,0.191382138078774,
-1.26097121103771));
#35023=CARTESIAN_POINT('Ctrl Pts',(-0.191508053525239,0.0561730490363835,
-1.24985342800064));
#35024=CARTESIAN_POINT('Ctrl Pts',(-0.151010679334637,-0.13048571082497,
-1.23873564496356));
#35025=CARTESIAN_POINT('Ctrl Pts',(0.0277994600910228,-0.197630807371493,
-1.22761786192649));
#35026=CARTESIAN_POINT('Ctrl Pts',(0.181147690371529,-0.0837631200245593,
-1.21650007888942));
#35027=CARTESIAN_POINT('Ctrl Pts',(0.168580251098708,0.106824364929836,
-1.20538229585234));
#35028=CARTESIAN_POINT('Ctrl Pts',(0.00160783334091074,0.199569939808722,
-1.19426451281528));
#35029=CARTESIAN_POINT('Ctrl Pts',(-0.166837221162941,0.10952665263698,
-1.1831467297782));
#35030=CARTESIAN_POINT('Ctrl Pts',(-0.182473762354565,-0.080833607215113,
-1.17202894674113));
#35031=CARTESIAN_POINT('Ctrl Pts',(-0.0309800663634189,-0.197157250669039,
-1.16091116370406));
#35032=CARTESIAN_POINT('Ctrl Pts',(0.148888699952624,-0.132901847352329,
-1.14979338066698));
#35033=CARTESIAN_POINT('Ctrl Pts',(0.192388251232866,0.0530801920758167,
-1.13867559762991));
#35034=CARTESIAN_POINT('Ctrl Pts',(0.0596767481410642,0.190445351044745,
-1.12755781459284));
#35035=CARTESIAN_POINT('Ctrl Pts',(-0.127693512146385,0.153378984737048,
-1.11644003155577));
#35036=CARTESIAN_POINT('Ctrl Pts',(-0.198107522415482,-0.0241693104089889,
-1.1053222485187));
#35037=CARTESIAN_POINT('Ctrl Pts',(-0.0870721189071633,-0.179580600601133,
-1.09420446548162));
#35038=CARTESIAN_POINT('Ctrl Pts',(0.103713839953251,-0.170511540387736,
-1.08308668244455));
#35039=CARTESIAN_POINT('Ctrl Pts',(0.199506861490193,-0.00526860717646393,
-1.07196889940748));
#35040=CARTESIAN_POINT('Ctrl Pts',(0.112568795279511,0.164799916057522,
-1.06085111637041));
#35041=CARTESIAN_POINT('Ctrl Pts',(-0.0774725840414104,0.183925921841359,
-1.04973333333333));
#35042=CARTESIAN_POINT('Ctrl Pts',(-0.19655575447285,0.0345916375278131,
-1.03861555029626));
#35043=CARTESIAN_POINT('Ctrl Pts',(-0.135610796800813,-0.146425604981832,
-1.02749776725919));
#35044=CARTESIAN_POINT('Ctrl Pts',(0.0495419611676193,-0.193329615131549,
-1.01637998422212));
#35045=CARTESIAN_POINT('Ctrl Pts',(0.18931855319524,-0.0631603627230562,
-1.00526220118505));
#35046=CARTESIAN_POINT('Ctrl Pts',(0.155695669647064,0.124858337552601,
-0.99414441814797));
#35047=CARTESIAN_POINT('Ctrl Pts',(-0.0205310264201175,0.198517563347386,
-0.9830266351109));
#35048=CARTESIAN_POINT('Ctrl Pts',(-0.177953072049209,0.0903518132164242,
-0.971908852073826));
#35049=CARTESIAN_POINT('Ctrl Pts',(-0.172385443134293,-0.100568409546141,
-0.960791069036755));
#35050=CARTESIAN_POINT('Ctrl Pts',(-0.00892760783500083,-0.199376638103845,
-0.949673285999682));
#35051=CARTESIAN_POINT('Ctrl Pts',(0.162707146686461,-0.115573052310637,
-0.938555502962609));
#35052=CARTESIAN_POINT('Ctrl Pts',(0.185316180106141,0.0740854870680833,
-0.927437719925537));
#35053=CARTESIAN_POINT('Ctrl Pts',(0.0381915666973661,0.195888106419067,
-0.916319936888465));
#35054=CARTESIAN_POINT('Ctrl Pts',(-0.143913229714983,0.138274105732958,
-0.905202153851392));
#35055=CARTESIAN_POINT('Ctrl Pts',(-0.194205912946527,-0.0459870566556826,
-0.89408437081432));
#35056=CARTESIAN_POINT('Ctrl Pts',(-0.0666227203577119,-0.188128039205709,
-0.882966587777248));
#35057=CARTESIAN_POINT('Ctrl Pts',(0.121981141238363,-0.157959954372725,
-0.871848804740174));
#35058=CARTESIAN_POINT('Ctrl Pts',(0.19886079216473,0.0168858326079224,
-0.860731021703104));
#35059=CARTESIAN_POINT('Ctrl Pts',(0.0936010991547904,0.176265652468829,
-0.84961323866603));
#35060=CARTESIAN_POINT('Ctrl Pts',(-0.0973891323197074,0.174201328666751,
-0.838495455628959));
#35061=CARTESIAN_POINT('Ctrl Pts',(-0.199179313476877,0.0125836038608601,
-0.827377672591885));
#35062=CARTESIAN_POINT('Ctrl Pts',(-0.118538412632168,-0.160559617382119,
-0.816259889554814));
#35063=CARTESIAN_POINT('Ctrl Pts',(0.0706734562402105,-0.186644069250297,
-0.80514210651774));
#35064=CARTESIAN_POINT('Ctrl Pts',(0.195154531208078,-0.0417786422972597,
-0.794024323480671));
#35065=CARTESIAN_POINT('Ctrl Pts',(0.140890877798356,0.14135241970499,-0.782906540443595));
#35066=CARTESIAN_POINT('Ctrl Pts',(-0.0424166749615475,0.195016849755228,
-0.771788757406524));
#35067=CARTESIAN_POINT('Ctrl Pts',(-0.186874209749804,0.0700626557706258,
-0.760670974369452));
#35068=CARTESIAN_POINT('Ctrl Pts',(-0.160171076857274,-0.119062891539001,
-0.749553191332379));
#35069=CARTESIAN_POINT('Ctrl Pts',(0.0132349557812702,-0.199137093352079,
-0.738435408295307));
#35070=CARTESIAN_POINT('Ctrl Pts',(0.174518909769793,-0.0968188831582442,
-0.727317625258234));
#35071=CARTESIAN_POINT('Ctrl Pts',(0.175958585839427,0.0941770782761695,
-0.716199842221161));
#35072=CARTESIAN_POINT('Ctrl Pts',(0.0162353648096416,0.198914954019915,
-0.70508205918409));
#35073=CARTESIAN_POINT('Ctrl Pts',(-0.158358050906612,0.121463878236724,
-0.693964276147017));
#35074=CARTESIAN_POINT('Ctrl Pts',(-0.187909142365856,-0.0672376398944485,
-0.682846493109945));
#35075=CARTESIAN_POINT('Ctrl Pts',(-0.0453516570786103,-0.194355275728422,
-0.671728710072871));
#35076=CARTESIAN_POINT('Ctrl Pts',(0.138744036805732,-0.143460232308806,
-0.660610927035801));
#35077=CARTESIAN_POINT('Ctrl Pts',(0.195762152632669,0.0388320177156751,
-0.649493143998727));
#35078=CARTESIAN_POINT('Ctrl Pts',(0.0734790112337116,0.185557486810322,
-0.638375360961656));
#35079=CARTESIAN_POINT('Ctrl Pts',(-0.116104570606568,0.162328292935986,
-0.627257577924582));
#35080=CARTESIAN_POINT('Ctrl Pts',(-0.199346373918836,-0.00957962466167244,
-0.616139794887511));
#35081=CARTESIAN_POINT('Ctrl Pts',(-0.100004082264906,-0.172713431827408,
-0.605022011850438));
#35082=CARTESIAN_POINT('Ctrl Pts',(0.0909333284489641,-0.177656623238313,
-0.593904228813366));
#35083=CARTESIAN_POINT('Ctrl Pts',(0.198583648704504,-0.01988166166227,
-0.582786445776293));
#35084=CARTESIAN_POINT('Ctrl Pts',(0.124348464543696,0.156103188208544,
-0.571668662739221));
#35085=CARTESIAN_POINT('Ctrl Pts',(-0.0637791943725893,0.189110973685903,
-0.560550879702148));
#35086=CARTESIAN_POINT('Ctrl Pts',(-0.193490608973672,0.0489094085247839,
-0.549433096665077));
#35087=CARTESIAN_POINT('Ctrl Pts',(-0.145981304534738,-0.136088958881986,
-0.538315313628003));
#35088=CARTESIAN_POINT('Ctrl Pts',(0.0352342913530302,-0.196441570743304,
-0.527197530590931));
#35089=CARTESIAN_POINT('Ctrl Pts',(0.184178313537193,-0.0768706369548383,
-0.516079747553859));
#35090=CARTESIAN_POINT('Ctrl Pts',(0.164430876586609,0.113107174079306,
-0.504961964516787));
#35091=CARTESIAN_POINT('Ctrl Pts',(-0.00592106946976007,0.199488563430541,
-0.493844181479714));
#35092=CARTESIAN_POINT('Ctrl Pts',(-0.170849826284632,0.103155624479512,
-0.482726398442642));
#35093=CARTESIAN_POINT('Ctrl Pts',(-0.179294869380122,-0.087658974538901,
-0.471608615405569));
#35094=CARTESIAN_POINT('Ctrl Pts',(-0.0235212672386517,-0.198185509033164,
-0.460490832368497));
#35095=CARTESIAN_POINT('Ctrl Pts',(0.15379578817364,-0.127191200730621,
-0.449373049331425));
#35096=CARTESIAN_POINT('Ctrl Pts',(0.190249158727879,0.0602992836323975,
-0.438255266294352));
#35097=CARTESIAN_POINT('Ctrl Pts',(0.052450699256103,0.192560821951897,
-0.42713748325728));
#35098=CARTESIAN_POINT('Ctrl Pts',(-0.133388079514004,0.148453245996245,
-0.416019700220208));
#35099=CARTESIAN_POINT('Ctrl Pts',(-0.197054875425419,-0.0316247067070998,
-0.404901917183135));
#35100=CARTESIAN_POINT('Ctrl Pts',(-0.0802363914648483,-0.182737154098266,
-0.393784134146063));
#35101=CARTESIAN_POINT('Ctrl Pts',(0.110071710746651,-0.166478120173837,
-0.38266635110899));
#35102=CARTESIAN_POINT('Ctrl Pts',(0.199563614032374,0.00226052151145618,
-0.371548568071918));
#35103=CARTESIAN_POINT('Ctrl Pts',(0.106272449134592,0.168928720347144,
-0.360430785034846));
#35104=CARTESIAN_POINT('Ctrl Pts',(-0.0843551185474909,0.18087277290543,
-0.349313001997773));
#35105=CARTESIAN_POINT('Ctrl Pts',(-0.197720669000457,0.0271529566091497,
-0.338195218960701));
#35106=CARTESIAN_POINT('Ctrl Pts',(-0.129991130062581,-0.151436627366443,
-0.327077435923628));
#35107=CARTESIAN_POINT('Ctrl Pts',(0.056799078860964,-0.191323314435221,
-0.315959652886556));
#35108=CARTESIAN_POINT('Ctrl Pts',(0.191566227578033,-0.055974337422329,
-0.304841869849484));
#35109=CARTESIAN_POINT('Ctrl Pts',(0.150875224767089,0.130642307676758,
-0.293724086812411));
#35110=CARTESIAN_POINT('Ctrl Pts',(-0.0280044786374454,0.197601860306157,
-0.282606303775339));
#35111=CARTESIAN_POINT('Ctrl Pts',(-0.181234493456315,0.0835751419292736,
-0.271488520738266));
#35112=CARTESIAN_POINT('Ctrl Pts',(-0.168469334814571,-0.106999202071807,
-0.260370737701194));
#35113=CARTESIAN_POINT('Ctrl Pts',(-0.00140078699449221,-0.199571500727773,
-0.249252954664122));
#35114=CARTESIAN_POINT('Ctrl Pts',(0.166950760111813,-0.109353506747779,
-0.238135171627049));
#35115=CARTESIAN_POINT('Ctrl Pts',(0.182389803640612,0.0810228714550746,
-0.227017388589977));
#35116=CARTESIAN_POINT('Ctrl Pts',(0.0307755058387974,0.197189286857941,
-0.215899605552904));
#35117=CARTESIAN_POINT('Ctrl Pts',(-0.149026496594129,0.132747306769101,
-0.204781822515832));
#35118=CARTESIAN_POINT('Ctrl Pts',(-0.192333085348998,-0.0532797515233865,
-0.19366403947876));
#35119=CARTESIAN_POINT('Ctrl Pts',(-0.0594791256025773,-0.190507173048921,
-0.182546256441687));
#35120=CARTESIAN_POINT('Ctrl Pts',(0.127852545543535,-0.153246402000575,
-0.171428473404615));
#35121=CARTESIAN_POINT('Ctrl Pts',(0.198082383035612,0.0243747804091565,
-0.160310690367542));
#35122=CARTESIAN_POINT('Ctrl Pts',(0.0868856852284144,0.179670923258195,
-0.14919290733047));
#35123=CARTESIAN_POINT('Ctrl Pts',(-0.103890530912397,0.170403686824479,
-0.138075124293398));
#35124=CARTESIAN_POINT('Ctrl Pts',(-0.199512508665682,0.00506193506719449,
-0.126957341256325));
#35125=CARTESIAN_POINT('Ctrl Pts',(-0.112397212591169,-0.164917203682897,
-0.115839558219253));
#35126=CARTESIAN_POINT('Ctrl Pts',(0.0776623121413626,-0.183844323471358,
-0.10472177518218));
#35127=CARTESIAN_POINT('Ctrl Pts',(0.196593525860617,-0.034389841833708,
-0.0936039921451079));
#35128=CARTESIAN_POINT('Ctrl Pts',(0.135455026238565,0.146570291745065,
-0.0824862091080354));
#35129=CARTESIAN_POINT('Ctrl Pts',(-0.049735296985837,0.19327035668827,
-0.0713684260709631));
#35130=CARTESIAN_POINT('Ctrl Pts',(-0.18939769988277,0.0629786854978793,
-0.0602506430338908));
#35131=CARTESIAN_POINT('Ctrl Pts',(-0.155539915651925,-0.125047929923611,
-0.0491328599968184));
#35132=CARTESIAN_POINT('Ctrl Pts',(0.0206870796054742,-0.198442384758988,
-0.0380150769597463));
#35133=CARTESIAN_POINT('Ctrl Pts',(0.178142926080333,-0.0902714528615779,
-0.0268972939226737));
#35134=CARTESIAN_POINT('Ctrl Pts',(0.172087026372346,0.100962540838038,
-0.0157795108856014));
#35135=CARTESIAN_POINT('Ctrl Pts',(0.0634850318392476,0.166218031662509,
-0.00836765552755316));
#35136=CARTESIAN_POINT('Ctrl Pts',(0.00737739821677115,0.168672073681436,
-0.00466172784852903));
#35137=CARTESIAN_POINT('Ctrl Pts',(0.0903606778650232,-0.126612599672282,
-1.5646));
#35138=CARTESIAN_POINT('Ctrl Pts',(0.132477509652,-0.0965547264460079,-1.56089407232098));
#35139=CARTESIAN_POINT('Ctrl Pts',(0.183629629053462,0.00837163889085661,
-1.55348221696293));
#35140=CARTESIAN_POINT('Ctrl Pts',(0.0923230570238932,0.159158029769189,
-1.54236443392586));
#35141=CARTESIAN_POINT('Ctrl Pts',(-0.0836206488085049,0.163699342626539,
-1.53124665088878));
#35142=CARTESIAN_POINT('Ctrl Pts',(-0.182934470289723,0.0185420837280834,
-1.52012886785171));
#35143=CARTESIAN_POINT('Ctrl Pts',(-0.114717412999509,-0.14372078954814,
-1.50901108481464));
#35144=CARTESIAN_POINT('Ctrl Pts',(0.0585821121664253,-0.174283509875506,
-1.49789330177756));
#35145=CARTESIAN_POINT('Ctrl Pts',(0.178219584548083,-0.0452513232337437,
-1.4867755187405));
#35146=CARTESIAN_POINT('Ctrl Pts',(0.134626373349144,0.125244912864161,
-1.47565773570342));
#35147=CARTESIAN_POINT('Ctrl Pts',(-0.0322746164076941,0.18101828554357,
-1.46453995266635));
#35148=CARTESIAN_POINT('Ctrl Pts',(-0.169613985667002,0.0709994086342611,
-1.45342216962927));
#35149=CARTESIAN_POINT('Ctrl Pts',(-0.151602013332166,-0.104051378974232,
-1.4423043865922));
#35150=CARTESIAN_POINT('Ctrl Pts',(0.00526457092671344,-0.183798721027812,
-1.43118660355513));
#35151=CARTESIAN_POINT('Ctrl Pts',(0.157309138173746,-0.095202988083288,
-1.42006882051806));
#35152=CARTESIAN_POINT('Ctrl Pts',(0.165272159879762,0.0805908485969487,
-1.40895103748099));
#35153=CARTESIAN_POINT('Ctrl Pts',(0.021860095314849,0.182570218824516,
-1.39783325444391));
#35154=CARTESIAN_POINT('Ctrl Pts',(-0.141573914269114,0.117331109047258,
-1.38671547140684));
#35155=CARTESIAN_POINT('Ctrl Pts',(-0.17533843141003,-0.0553732368534328,
-1.37559768836977));
#35156=CARTESIAN_POINT('Ctrl Pts',(-0.048508054493723,-0.177360442508133,
-1.3644799053327));
#35157=CARTESIAN_POINT('Ctrl Pts',(0.12275151636726,-0.136900786130964,
-1.35336212229563));
#35158=CARTESIAN_POINT('Ctrl Pts',(0.181581280715027,0.0289481974204555,
-1.34224433925855));
#35159=CARTESIAN_POINT('Ctrl Pts',(0.0740982434113141,0.1682831233296,-1.33112655622148));
#35160=CARTESIAN_POINT('Ctrl Pts',(-0.101252397253136,0.153485216344168,
-1.32000877318441));
#35161=CARTESIAN_POINT('Ctrl Pts',(-0.183864570130966,-0.00189191961280822,
-1.30889099014733));
#35162=CARTESIAN_POINT('Ctrl Pts',(-0.0980726456853608,-0.155536219688844,
-1.29777320711026));
#35163=CARTESIAN_POINT('Ctrl Pts',(0.0775453683472552,-0.166722749977294,
-1.28665542407319));
#35164=CARTESIAN_POINT('Ctrl Pts',(0.18213850936899,-0.025205612527195,
-1.27553764103612));
#35165=CARTESIAN_POINT('Ctrl Pts',(0.119908476028974,0.139397693201698,
-1.26441985799905));
#35166=CARTESIAN_POINT('Ctrl Pts',(-0.0521473853035587,0.176324728004856,
-1.25330207496197));
#35167=CARTESIAN_POINT('Ctrl Pts',(-0.176440736777005,0.0517535110223655,
-1.2421842919249));
#35168=CARTESIAN_POINT('Ctrl Pts',(-0.139129582451151,-0.120219460920973,
-1.23106650888783));
#35169=CARTESIAN_POINT('Ctrl Pts',(0.0256122765083437,-0.182081769516105,
-1.21994872585076));
#35170=CARTESIAN_POINT('Ctrl Pts',(0.166895497950393,-0.0771728725754398,
-1.20883094281368));
#35171=CARTESIAN_POINT('Ctrl Pts',(0.155316829566065,0.0984197233850115,
-1.19771315977661));
#35172=CARTESIAN_POINT('Ctrl Pts',(0.00148133352129465,0.183868336449635,
-1.18659537673954));
#35173=CARTESIAN_POINT('Ctrl Pts',(-0.153710936338967,0.100909402671365,
-1.17547759370247));
#35174=CARTESIAN_POINT('Ctrl Pts',(-0.168117238307517,-0.0744738456207954,
-1.16435981066539));
#35175=CARTESIAN_POINT('Ctrl Pts',(-0.0285426415962272,-0.181645470927358,
-1.15324202762832));
#35176=CARTESIAN_POINT('Ctrl Pts',(0.137174554457832,-0.122445502600127,
-1.14212424459125));
#35177=CARTESIAN_POINT('Ctrl Pts',(0.177251682996677,0.0489039913764663,
-1.13100646155418));
#35178=CARTESIAN_POINT('Ctrl Pts',(0.0549815489042986,0.175461644748333,
-1.11988867851711));
#35179=CARTESIAN_POINT('Ctrl Pts',(-0.117646944606339,0.141311556224172,
-1.10877089548003));
#35180=CARTESIAN_POINT('Ctrl Pts',(-0.182520977956929,-0.0222677368259724,
-1.09765311244296));
#35181=CARTESIAN_POINT('Ctrl Pts',(-0.0802215287029169,-0.165451702409712,
-1.08653532940589));
#35182=CARTESIAN_POINT('Ctrl Pts',(0.0955539257930597,-0.157096170428305,
-1.07541754636882));
#35183=CARTESIAN_POINT('Ctrl Pts',(0.183810220956364,-0.00485408793464279,
-1.06429976333174));
#35184=CARTESIAN_POINT('Ctrl Pts',(0.103712198059592,0.151833920687547,
-1.05318198029467));
#35185=CARTESIAN_POINT('Ctrl Pts',(-0.0713772583275903,0.169455145957098,
-1.0420641972576));
#35186=CARTESIAN_POINT('Ctrl Pts',(-0.181091298765559,0.031870064466641,
-1.03094641422053));
#35187=CARTESIAN_POINT('Ctrl Pts',(-0.12494131950069,-0.134905248893923,
-1.01982863118345));
#35188=CARTESIAN_POINT('Ctrl Pts',(0.0456441385565052,-0.178118983022976,
-1.00871084814638));
#35189=CARTESIAN_POINT('Ctrl Pts',(0.174423500194588,-0.0581910824574806,
-0.997593065109308));
#35190=CARTESIAN_POINT('Ctrl Pts',(0.143445970860419,0.11503483360103,-0.986475282072236));
#35191=CARTESIAN_POINT('Ctrl Pts',(-0.0189157028212204,0.182898758017883,
-0.975357499035165));
#35192=CARTESIAN_POINT('Ctrl Pts',(-0.163952223241389,0.0832431858587246,
-0.96423971599809));
#35193=CARTESIAN_POINT('Ctrl Pts',(-0.158822639760351,-0.0926559690319977,
-0.95312193296102));
#35194=CARTESIAN_POINT('Ctrl Pts',(-0.00822520867957112,-0.183690243180965,
-0.942004149923946));
#35195=CARTESIAN_POINT('Ctrl Pts',(0.14990580454341,-0.106480088570106,
-0.930886366886874));
#35196=CARTESIAN_POINT('Ctrl Pts',(0.170736022599271,0.0682566486482162,
-0.919768583849802));
#35197=CARTESIAN_POINT('Ctrl Pts',(0.0351867613017287,0.18047617938886,
-0.908650800812729));
#35198=CARTESIAN_POINT('Ctrl Pts',(-0.132590540269491,0.127395086752784,
-0.897533017775657));
#35199=CARTESIAN_POINT('Ctrl Pts',(-0.178926336182619,-0.0423689239652017,
-0.886415234738584));
#35200=CARTESIAN_POINT('Ctrl Pts',(-0.0613810315003473,-0.173326652508083,
-0.875297451701512));
#35201=CARTESIAN_POINT('Ctrl Pts',(0.112384007026421,-0.145532108011909,
-0.86417966866444));
#35202=CARTESIAN_POINT('Ctrl Pts',(0.183214982554139,0.0155573026386719,
-0.853061885627367));
#35203=CARTESIAN_POINT('Ctrl Pts',(0.086236827089008,0.162397565102822,
-0.841944102590294));
#35204=CARTESIAN_POINT('Ctrl Pts',(-0.0897268284244655,0.160495656510048,
-0.830826319553223));
#35205=CARTESIAN_POINT('Ctrl Pts',(-0.183508443502437,0.0115935611878976,
-0.819708536516149));
#35206=CARTESIAN_POINT('Ctrl Pts',(-0.109212142655086,-0.14792723682402,
-0.808590753479079));
#35207=CARTESIAN_POINT('Ctrl Pts',(0.0651130668400682,-0.171959437148373,
-0.797472970442005));
#35208=CARTESIAN_POINT('Ctrl Pts',(0.179800319818854,-0.0384916158499819,
-0.786355187404933));
#35209=CARTESIAN_POINT('Ctrl Pts',(0.129805978528337,0.130231207611715,
-0.775237404367861));
#35210=CARTESIAN_POINT('Ctrl Pts',(-0.039079449893004,0.179673470756717,
-0.764119621330788));
#35211=CARTESIAN_POINT('Ctrl Pts',(-0.172171470838591,0.0645503224390171,
-0.753001838293716));
#35212=CARTESIAN_POINT('Ctrl Pts',(-0.147569265578375,-0.109695357031935,
-0.741884055256643));
#35213=CARTESIAN_POINT('Ctrl Pts',(0.0121936665653112,-0.183469545138692,
-0.730766272219571));
#35214=CARTESIAN_POINT('Ctrl Pts',(0.160788251222258,-0.0892014448683006,
-0.719648489182499));
#35215=CARTESIAN_POINT('Ctrl Pts',(0.162114657614943,0.0867674897879067,
-0.708530706145426));
#35216=CARTESIAN_POINT('Ctrl Pts',(0.014958011823137,0.183264883106403,
-0.697412923108354));
#35217=CARTESIAN_POINT('Ctrl Pts',(-0.145898883426596,0.111907440827576,
-0.686295140071281));
#35218=CARTESIAN_POINT('Ctrl Pts',(-0.1731249778579,-0.0619475708918949,
-0.675177357034209));
#35219=CARTESIAN_POINT('Ctrl Pts',(-0.041783515845475,-0.179063947519582,
-0.664059573997137));
#35220=CARTESIAN_POINT('Ctrl Pts',(0.127828044966229,-0.132173183429228,
-0.652941790960064));
#35221=CARTESIAN_POINT('Ctrl Pts',(0.180360135293257,0.0357768234294574,
-0.641824007922992));
#35222=CARTESIAN_POINT('Ctrl Pts',(0.0676978886322038,0.170958343968484,
-0.630706224885919));
#35223=CARTESIAN_POINT('Ctrl Pts',(-0.106969788496654,0.149556757943885,
-0.619588441848848));
#35224=CARTESIAN_POINT('Ctrl Pts',(-0.183662360097186,-0.00882592665028588,
-0.608470658811774));
#35225=CARTESIAN_POINT('Ctrl Pts',(-0.0921360414391275,-0.159124823222627,
-0.597352875774703));
#35226=CARTESIAN_POINT('Ctrl Pts',(0.0837789491030789,-0.163679098191823,
-0.58623509273763));
#35227=CARTESIAN_POINT('Ctrl Pts',(0.182959643964377,-0.01831742826199,
-0.575117309700558));
#35228=CARTESIAN_POINT('Ctrl Pts',(0.114565075971008,0.143821427003983,
-0.563999526663485));
#35229=CARTESIAN_POINT('Ctrl Pts',(-0.0587612261677574,0.174232252459085,
-0.552881743626413));
#35230=CARTESIAN_POINT('Ctrl Pts',(-0.178267310320956,0.0450613533822114,
-0.54176396058934));
#35231=CARTESIAN_POINT('Ctrl Pts',(-0.134495904760386,-0.12538186112987,
-0.530646177552268));
#35232=CARTESIAN_POINT('Ctrl Pts',(0.032462156090606,-0.180986098691733,
-0.519528394515196));
#35233=CARTESIAN_POINT('Ctrl Pts',(0.169687680181897,-0.0708226707501974,
-0.508410611478123));
#35234=CARTESIAN_POINT('Ctrl Pts',(0.151493916207583,0.104208218724794,
-0.497292828441051));
#35235=CARTESIAN_POINT('Ctrl Pts',(-0.00545521632391679,0.183793362536746,
-0.486175045403978));
#35236=CARTESIAN_POINT('Ctrl Pts',(-0.157407840939238,0.0950396291478065,
-0.475057262366907));
#35237=CARTESIAN_POINT('Ctrl Pts',(-0.165188451720106,-0.0807622121788323,
-0.463939479329833));
#35238=CARTESIAN_POINT('Ctrl Pts',(-0.0216706798754521,-0.182592828806171,
-0.452821696292762));
#35239=CARTESIAN_POINT('Ctrl Pts',(0.141695566734905,-0.117184153644509,
-0.441703913255688));
#35240=CARTESIAN_POINT('Ctrl Pts',(0.175280888292921,0.0555551050484869,
-0.430586130218617));
#35241=CARTESIAN_POINT('Ctrl Pts',(0.0483240252869895,0.177410676335346,
-0.419468347181544));
#35242=CARTESIAN_POINT('Ctrl Pts',(-0.1228934793785,0.136773360797922,-0.408350564144472));
#35243=CARTESIAN_POINT('Ctrl Pts',(-0.181551150280891,-0.0291365634449526,
-0.397232781107399));
#35244=CARTESIAN_POINT('Ctrl Pts',(-0.0739236171314337,-0.168359907127257,
-0.386114998070327));
#35245=CARTESIAN_POINT('Ctrl Pts',(0.101411577137068,-0.153380088408926,
-0.374997215033255));
#35246=CARTESIAN_POINT('Ctrl Pts',(0.183862508367636,0.00208267001642915,
-0.363879431996182));
#35247=CARTESIAN_POINT('Ctrl Pts',(0.0979112307772101,0.155637882230987,
-0.35276164895911));
#35248=CARTESIAN_POINT('Ctrl Pts',(-0.0777182943142881,0.166642210219781,
-0.341643865922037));
#35249=CARTESIAN_POINT('Ctrl Pts',(-0.182164561084034,0.025016638107916,
-0.330526082884965));
#35250=CARTESIAN_POINT('Ctrl Pts',(-0.119763792386384,-0.139522018085984,
-0.319408299847893));
#35251=CARTESIAN_POINT('Ctrl Pts',(0.0523302865754574,-0.176270532440662,
-0.30829051681082));
#35252=CARTESIAN_POINT('Ctrl Pts',(0.176494333858419,-0.0515704334810062,
-0.297172733773748));
#35253=CARTESIAN_POINT('Ctrl Pts',(0.139004785069224,0.12036373717149,-0.286054950736676));
#35254=CARTESIAN_POINT('Ctrl Pts',(-0.0258011647703144,0.182055099924714,
-0.274937167699603));
#35255=CARTESIAN_POINT('Ctrl Pts',(-0.166975471611825,0.0769996840696845,
-0.26381938466253));
#35256=CARTESIAN_POINT('Ctrl Pts',(-0.155214639864204,-0.0985808048308175,
-0.252701601625459));
#35257=CARTESIAN_POINT('Ctrl Pts',(-0.0012905770009465,-0.183869774559952,
-0.241583818588386));
#35258=CARTESIAN_POINT('Ctrl Pts',(0.153815542361654,-0.100749879415303,
-0.230466035551314));
#35259=CARTESIAN_POINT('Ctrl Pts',(0.168039885229795,0.0746482190809691,
-0.219348252514241));
#35260=CARTESIAN_POINT('Ctrl Pts',(0.0283541753201865,0.181674986598733,
-0.208230469477169));
#35261=CARTESIAN_POINT('Ctrl Pts',(-0.137301509645904,0.122303120836724,
-0.197112686440096));
#35262=CARTESIAN_POINT('Ctrl Pts',(-0.177200857409891,-0.0490878500461769,
-0.185994903403024));
#35263=CARTESIAN_POINT('Ctrl Pts',(-0.0547994747530945,-0.175518602770541,
-0.174877120365952));
#35264=CARTESIAN_POINT('Ctrl Pts',(0.11779346570166,-0.141189404725702,
-0.163759337328879));
#35265=CARTESIAN_POINT('Ctrl Pts',(0.182497816472988,0.0224570410225731,
-0.152641554291807));
#35266=CARTESIAN_POINT('Ctrl Pts',(0.080049763103335,0.16553491873334,-0.141523771254734));
#35267=CARTESIAN_POINT('Ctrl Pts',(-0.0957167152029026,0.156996802481032,
-0.130405988217662));
#35268=CARTESIAN_POINT('Ctrl Pts',(-0.183815423827918,0.00466367620751416,
-0.11928820518059));
#35269=CARTESIAN_POINT('Ctrl Pts',(-0.103554115016128,-0.15194198045138,
-0.108170422143517));
#35270=CARTESIAN_POINT('Ctrl Pts',(0.0715520591525512,-0.169379967518084,
-0.0970526391064447));
#35271=CARTESIAN_POINT('Ctrl Pts',(0.181126098406431,-0.0316841454920027,
-0.0859348560693724));
#35272=CARTESIAN_POINT('Ctrl Pts',(0.124797804529567,0.135038552108262,
-0.0748170730322999));
#35273=CARTESIAN_POINT('Ctrl Pts',(-0.0458222632545728,0.17806438686788,
-0.0636992899952276));
#35274=CARTESIAN_POINT('Ctrl Pts',(-0.174496419842635,0.0580236990870384,
-0.0525815069581552));
#35275=CARTESIAN_POINT('Ctrl Pts',(-0.143302471152953,-0.115209509375821,
-0.0414637239210829));
#35276=CARTESIAN_POINT('Ctrl Pts',(0.0190594781794568,-0.182829494270053,
-0.0303459408840108));
#35277=CARTESIAN_POINT('Ctrl Pts',(0.16412714008961,-0.083169148031303,
-0.0192281578469382));
#35278=CARTESIAN_POINT('Ctrl Pts',(0.158547701592606,0.0930190911788169,
-0.00811037480986587));
#35279=CARTESIAN_POINT('Ctrl Pts',(0.0584902075178373,0.153140462932497,
-0.000698519451817671));
#35280=CARTESIAN_POINT('Ctrl Pts',(0.0067969652080078,0.155401427805413,
0.00300740822720647));
#35281=CARTESIAN_POINT('Ctrl Pts',(0.00853826423430342,0.195213365433479,
-0.0200000000000003));
#35282=CARTESIAN_POINT('Ctrl Pts',(0.0734746804820721,0.19237316912253,
-0.0237059276790243));
#35283=CARTESIAN_POINT('Ctrl Pts',(0.136320178206947,0.154611304639505,
-0.0274118553580483));
#35284=CARTESIAN_POINT('Ctrl Pts',(0.168911064091045,0.0988427886182253,
-0.0311177830370723));
#35285=CARTESIAN_POINT('Ctrl Pts',(0.201501949975142,0.0430742725969455,
-0.0348237107160964));
#35286=CARTESIAN_POINT('Ctrl Pts',(0.203838224018461,-0.0307008949625867,
-0.0385296383951203));
#35287=CARTESIAN_POINT('Ctrl Pts',(0.174634325106077,-0.0884538292781432,
-0.0422355660741444));
#35288=CARTESIAN_POINT('Ctrl Pts',(0.145430426193693,-0.146206763593701,
-0.0459414937531686));
#35289=CARTESIAN_POINT('Ctrl Pts',(0.0846863543255994,-0.187937464665282,
-0.049647421432193));
#35290=CARTESIAN_POINT('Ctrl Pts',(0.0203214705403238,-0.194645582748126,
-0.0533533491112172));
#35291=CARTESIAN_POINT('Ctrl Pts',(-0.0440434132449519,-0.20135370083097,
-0.0570592767902414));
#35292=CARTESIAN_POINT('Ctrl Pts',(-0.112029108947411,-0.17303923592508,
-0.0607652044692654));
#35293=CARTESIAN_POINT('Ctrl Pts',(-0.152552866017503,-0.122613098582343,
-0.0644711321482895));
#35294=CARTESIAN_POINT('Ctrl Pts',(-0.180042705249534,-0.0884058456307822,
-0.0669850983613853));
#35295=CARTESIAN_POINT('Ctrl Pts',(-0.194895189472664,-0.0440233075995439,
-0.069499064574481));
#35296=CARTESIAN_POINT('Ctrl Pts',(-0.195234571671998,0.00015548015543182,
-0.0720130307875768));
#35297=CARTESIAN_POINT('Origin',(0.,0.,-0.02));
#35298=CARTESIAN_POINT('',(-0.2154,2.6378892053634E-17,0.));
#35299=CARTESIAN_POINT('Origin',(-0.2154,-2.6378892053634E-17,-0.02));
#35300=CARTESIAN_POINT('Origin',(0.,0.,0.));
#35301=CARTESIAN_POINT('Origin',(0.,0.,-0.02));
#35302=CARTESIAN_POINT('Origin',(0.,0.,-0.78));
#35303=CARTESIAN_POINT('Origin',(0.35,0.,0.));
#35304=CARTESIAN_POINT('',(0.330485534147499,-0.115235895966675,0.));
#35305=CARTESIAN_POINT('',(0.317616105825637,-0.115602808444076,0.));
#35306=CARTESIAN_POINT('',(0.335441504501922,-0.115094599297143,0.));
#35307=CARTESIAN_POINT('',(0.327238813083405,-0.124156188777542,0.));
#35308=CARTESIAN_POINT('',(0.318650451154949,-0.116522211763823,0.));
#35309=CARTESIAN_POINT('',(0.305454212950408,-0.170873414523286,0.));
#35310=CARTESIAN_POINT('Origin',(0.,0.,0.));
#35311=CARTESIAN_POINT('',(0.29271658647914,-0.169,0.));
#35312=CARTESIAN_POINT('',(0.308586965898532,-0.171334171076645,-2.77555756156289E-17));
#35313=CARTESIAN_POINT('',(0.300707824283758,-0.179094400846393,0.));
#35314=CARTESIAN_POINT('',(0.279811089486919,-0.152697987352333,0.));
#35315=CARTESIAN_POINT('',(0.27114182006011,-0.221319030845725,0.));
#35316=CARTESIAN_POINT('Origin',(0.,0.,0.));
#35317=CARTESIAN_POINT('',(0.258923021774215,-0.21726221207405,0.));
#35318=CARTESIAN_POINT('',(0.267454002283238,-0.22009462169896,-2.77555756156289E-17));
#35319=CARTESIAN_POINT('',(0.265039980408751,-0.228590920171666,0.));
#35320=CARTESIAN_POINT('',(0.236940191931664,-0.176549649291667,5.55111512312578E-17));
#35321=CARTESIAN_POINT('',(0.228590920171666,-0.265039980408751,0.));
#35322=CARTESIAN_POINT('Origin',(0.,0.,0.));
#35323=CARTESIAN_POINT('',(0.21726221207405,-0.258923021774215,0.));
#35324=CARTESIAN_POINT('',(0.214525877254124,-0.257445532305909,0.));
#35325=CARTESIAN_POINT('',(0.221319030845725,-0.27114182006011,0.));
#35326=CARTESIAN_POINT('',(0.193859348761916,-0.188435558020616,-2.77555756156289E-17));
#35327=CARTESIAN_POINT('',(0.179094400846393,-0.300707824283758,0.));
#35328=CARTESIAN_POINT('Origin',(0.,0.,0.));
#35329=CARTESIAN_POINT('',(0.169,-0.29271658647914,0.));
#35330=CARTESIAN_POINT('',(0.153407416225873,-0.280372709232379,0.));
#35331=CARTESIAN_POINT('',(0.170873414523285,-0.305454212950408,0.));
#35332=CARTESIAN_POINT('',(0.153874180716026,-0.189873871363808,0.));
#35333=CARTESIAN_POINT('',(0.124156188777542,-0.327238813083405,0.));
#35334=CARTESIAN_POINT('Origin',(0.,0.,0.));
#35335=CARTESIAN_POINT('',(0.115602808444076,-0.317616105825637,0.));
#35336=CARTESIAN_POINT('',(0.0884746524536336,-0.287096440691874,0.));
#35337=CARTESIAN_POINT('',(0.115235895966675,-0.330485534147499,0.));
#35338=CARTESIAN_POINT('',(0.119433076204517,-0.183269744138128,2.77555756156289E-17));
#35339=CARTESIAN_POINT('',(0.0654455537387477,-0.343826816138341,0.));
#35340=CARTESIAN_POINT('Origin',(0.,0.,0.));
#35341=CARTESIAN_POINT('',(0.0586930840514223,-0.332865020518126,0.));
#35342=CARTESIAN_POINT('',(0.0244380373436002,-0.277256207985893,2.77555756156289E-17));
#35343=CARTESIAN_POINT('',(0.0560969930232948,-0.345475219623267,0.));
#35344=CARTESIAN_POINT('',(0.0919040248701096,-0.171546880416256,0.));
#35345=CARTESIAN_POINT('',(0.00474638866665021,-0.349967815369678,0.));
#35346=CARTESIAN_POINT('Origin',(0.,0.,0.));
#35347=CARTESIAN_POINT('',(-6.20895927167708E-17,-0.338,0.));
#35348=CARTESIAN_POINT('',(-0.0341308674003153,-0.251940482303103,-2.77555756156289E-17));
#35349=CARTESIAN_POINT('',(-0.00474638866665032,-0.349967815369678,0.));
#35350=CARTESIAN_POINT('',(0.0714942725679436,-0.157730259324412,0.));
#35351=CARTESIAN_POINT('',(-0.0560969930232949,-0.345475219623267,0.));
#35352=CARTESIAN_POINT('Origin',(0.,0.,0.));
#35353=CARTESIAN_POINT('',(-0.0586930840514224,-0.332865020518126,0.));
#35354=CARTESIAN_POINT('',(-0.0832550096107083,-0.213558429049481,0.));
#35355=CARTESIAN_POINT('',(-0.0654455537387478,-0.343826816138341,0.));
#35356=CARTESIAN_POINT('',(0.0573199163702635,-0.144532327622448,5.55111512312578E-17));
#35357=CARTESIAN_POINT('',(-0.115235895966675,-0.330485534147499,0.));
#35358=CARTESIAN_POINT('Origin',(0.,0.,0.));
#35359=CARTESIAN_POINT('',(-0.115602808444076,-0.317616105825637,0.));
#35360=CARTESIAN_POINT('',(-0.11993773416091,-0.1655689032104,0.));
#35361=CARTESIAN_POINT('',(-0.124156188777542,-0.327238813083405,0.));
#35362=CARTESIAN_POINT('',(0.0476141712835098,-0.13399405767813,0.));
#35363=CARTESIAN_POINT('',(-0.170873414523286,-0.305454212950408,0.));
#35364=CARTESIAN_POINT('Origin',(0.,0.,0.));
#35365=CARTESIAN_POINT('',(-0.169,-0.29271658647914,0.));
#35366=CARTESIAN_POINT('',(-0.142435244588531,-0.112098828088702,0.));
#35367=CARTESIAN_POINT('',(-0.179094400846393,-0.300707824283758,0.));
#35368=CARTESIAN_POINT('',(0.0400460999029137,-0.127225130188389,0.));
#35369=CARTESIAN_POINT('',(-0.221319030845725,-0.27114182006011,0.));
#35370=CARTESIAN_POINT('Origin',(0.,0.,0.));
#35371=CARTESIAN_POINT('',(-0.21726221207405,-0.258923021774215,0.));
#35372=CARTESIAN_POINT('',(-0.150385479533696,-0.0574959058685693,0.));
#35373=CARTESIAN_POINT('',(-0.228590920171666,-0.265039980408751,0.));
#35374=CARTESIAN_POINT('',(0.0321081520112096,-0.124274994069283,0.));
#35375=CARTESIAN_POINT('',(-0.265039980408751,-0.228590920171666,0.));
#35376=CARTESIAN_POINT('Origin',(0.,0.,0.));
#35377=CARTESIAN_POINT('',(-0.258923021774215,-0.21726221207405,0.));
#35378=CARTESIAN_POINT('',(-0.144780334443528,-0.00586807595124715,0.));
#35379=CARTESIAN_POINT('',(-0.27114182006011,-0.221319030845725,0.));
#35380=CARTESIAN_POINT('',(0.0215225383940517,-0.124150206596651,0.));
#35381=CARTESIAN_POINT('',(-0.300707824283758,-0.179094400846393,0.));
#35382=CARTESIAN_POINT('Origin',(0.,0.,0.));
#35383=CARTESIAN_POINT('',(-0.29271658647914,-0.169,0.));
#35384=CARTESIAN_POINT('',(-0.127786749933849,0.0393366710293742,0.));
#35385=CARTESIAN_POINT('',(-0.305454212950408,-0.170873414523285,0.));
#35386=CARTESIAN_POINT('',(0.00661426644602217,-0.124975254227913,-2.77555756156289E-17));
#35387=CARTESIAN_POINT('',(-0.327238813083405,-0.124156188777542,0.));
#35388=CARTESIAN_POINT('Origin',(0.,0.,0.));
#35389=CARTESIAN_POINT('',(-0.317616105825637,-0.115602808444076,0.));
#35390=CARTESIAN_POINT('',(-0.102440047215055,0.0756617305936987,0.));
#35391=CARTESIAN_POINT('',(-0.330485534147499,-0.115235895966675,0.));
#35392=CARTESIAN_POINT('',(-0.0133971428466065,-0.124276211068284,-2.77555756156289E-17));
#35393=CARTESIAN_POINT('',(-0.343826816138341,-0.0654455537387478,0.));
#35394=CARTESIAN_POINT('Origin',(0.,0.,0.));
#35395=CARTESIAN_POINT('',(-0.332865020518126,-0.0586930840514225,0.));
#35396=CARTESIAN_POINT('',(-0.0722478752597442,0.101847162667754,0.));
#35397=CARTESIAN_POINT('',(-0.345475219623267,-0.0560969930232949,0.));
#35398=CARTESIAN_POINT('',(-0.0382251670489203,-0.119351276181666,0.));
#35399=CARTESIAN_POINT('',(-0.349967815369678,-0.0047463886666502,0.));
#35400=CARTESIAN_POINT('Origin',(0.,0.,0.));
#35401=CARTESIAN_POINT('',(-0.338,4.13930618111805E-17,0.));
#35402=CARTESIAN_POINT('',(-0.0407534494926875,0.117886816845732,0.));
#35403=CARTESIAN_POINT('',(-0.349967815369678,0.00474638866665025,0.));
#35404=CARTESIAN_POINT('',(-0.0664862087698295,-0.107681305378358,-2.77555756156289E-17));
#35405=CARTESIAN_POINT('',(-0.345475219623267,0.0560969930232949,0.));
#35406=CARTESIAN_POINT('Origin',(0.,0.,0.));
#35407=CARTESIAN_POINT('',(-0.332865020518126,0.0586930840514224,0.));
#35408=CARTESIAN_POINT('',(-0.0111111777379252,0.124933296243372,0.));
#35409=CARTESIAN_POINT('',(-0.343826816138341,0.0654455537387477,0.));
#35410=CARTESIAN_POINT('',(-0.0958175276338027,-0.087328249096412,2.77555756156289E-17));
#35411=CARTESIAN_POINT('',(-0.330485534147499,0.115235895966675,0.));
#35412=CARTESIAN_POINT('Origin',(0.,0.,0.));
#35413=CARTESIAN_POINT('',(-0.317616105825637,0.115602808444076,0.));
#35414=CARTESIAN_POINT('',(0.0142742316533668,0.125065132869389,-2.77555756156289E-17));
#35415=CARTESIAN_POINT('',(-0.327238813083405,0.124156188777542,0.));
#35416=CARTESIAN_POINT('',(-0.123130440725462,-0.0572705647603282,0.));
#35417=CARTESIAN_POINT('',(-0.305454212950408,0.170873414523285,0.));
#35418=CARTESIAN_POINT('Origin',(0.,0.,0.));
#35419=CARTESIAN_POINT('',(-0.29271658647914,0.169,0.));
#35420=CARTESIAN_POINT('',(0.0340022454231837,0.1209471067787,5.55111512312578E-17));
#35421=CARTESIAN_POINT('',(-0.300707824283758,0.179094400846393,0.));
#35422=CARTESIAN_POINT('',(-0.144969217443638,-0.017632059201444,0.));
#35423=CARTESIAN_POINT('',(-0.27114182006011,0.221319030845725,0.));
#35424=CARTESIAN_POINT('Origin',(0.,0.,0.));
#35425=CARTESIAN_POINT('',(-0.258923021774215,0.21726221207405,0.));
#35426=CARTESIAN_POINT('',(0.0477949519661669,0.115427383119028,-2.77555756156289E-17));
#35427=CARTESIAN_POINT('',(-0.265039980408751,0.228590920171666,0.));
#35428=CARTESIAN_POINT('',(-0.157932795372159,0.0302266501264093,0.));
#35429=CARTESIAN_POINT('',(-0.228590920171666,0.265039980408751,0.));
#35430=CARTESIAN_POINT('Origin',(0.,0.,0.));
#35431=CARTESIAN_POINT('',(-0.21726221207405,0.258923021774215,0.));
#35432=CARTESIAN_POINT('',(0.0564667261863714,0.111122533140651,0.));
#35433=CARTESIAN_POINT('',(-0.221319030845725,0.27114182006011,0.));
#35434=CARTESIAN_POINT('',(-0.15910830301132,0.0837683194406838,0.));
#35435=CARTESIAN_POINT('',(-0.179094400846393,0.300707824283758,0.));
#35436=CARTESIAN_POINT('Origin',(0.,0.,0.));
#35437=CARTESIAN_POINT('',(-0.169,0.29271658647914,0.));
#35438=CARTESIAN_POINT('',(0.0617507117308451,0.110042662678602,-2.77555756156289E-17));
#35439=CARTESIAN_POINT('',(-0.170873414523285,0.305454212950408,0.));
#35440=CARTESIAN_POINT('',(-0.146463392037742,0.139486807065864,2.77555756156289E-17));
#35441=CARTESIAN_POINT('',(-0.124156188777542,0.327238813083405,0.));
#35442=CARTESIAN_POINT('Origin',(0.,0.,0.));
#35443=CARTESIAN_POINT('',(-0.115602808444076,0.317616105825637,0.));
#35444=CARTESIAN_POINT('',(0.0660053371168799,0.113303664167723,0.));
#35445=CARTESIAN_POINT('',(-0.115235895966675,0.330485534147499,0.));
#35446=CARTESIAN_POINT('',(-0.119148812359806,0.193240277710374,-2.77555756156289E-17));
#35447=CARTESIAN_POINT('',(-0.0654455537387477,0.343826816138341,0.));
#35448=CARTESIAN_POINT('Origin',(0.,0.,0.));
#35449=CARTESIAN_POINT('',(-0.0586930840514224,0.332865020518126,0.));
#35450=CARTESIAN_POINT('',(0.0718388299416056,0.12096267524839,0.));
#35451=CARTESIAN_POINT('',(-0.0560969930232949,0.345475219623267,0.));
#35452=CARTESIAN_POINT('',(-0.0776729895490008,0.240672418360475,0.));
#35453=CARTESIAN_POINT('',(-0.00474638866665024,0.349967815369678,0.));
#35454=CARTESIAN_POINT('Origin',(0.,0.,0.));
#35455=CARTESIAN_POINT('',(2.06965309055903E-17,0.338,0.));
#35456=CARTESIAN_POINT('',(0.0816997840353174,0.13199750004727,0.));
#35457=CARTESIAN_POINT('',(0.00474638866665027,0.349967815369678,0.));
#35458=CARTESIAN_POINT('',(-0.0239253559329411,0.277673241580245,0.));
#35459=CARTESIAN_POINT('',(0.0560969930232949,0.345475219623267,0.));
#35460=CARTESIAN_POINT('Origin',(0.,0.,0.));
#35461=CARTESIAN_POINT('',(0.0586930840514225,0.332865020518126,0.));
#35462=CARTESIAN_POINT('',(0.0974860449318179,0.144432891105261,-2.77555756156289E-17));
#35463=CARTESIAN_POINT('',(0.0654455537387478,0.343826816138341,0.));
#35464=CARTESIAN_POINT('',(0.0389569509149426,0.300825860359951,5.55111512312578E-17));
#35465=CARTESIAN_POINT('',(0.115235895966675,0.330485534147499,0.));
#35466=CARTESIAN_POINT('Origin',(0.,0.,0.));
#35467=CARTESIAN_POINT('',(0.115602808444076,0.317616105825637,0.));
#35468=CARTESIAN_POINT('',(0.120221998005621,0.155598369638155,-2.77555756156289E-17));
#35469=CARTESIAN_POINT('',(0.124156188777542,0.327238813083405,0.));
#35470=CARTESIAN_POINT('',(0.106865818287004,0.307786834202281,2.77555756156289E-17));
#35471=CARTESIAN_POINT('',(0.170873414523285,0.305454212950408,0.));
#35472=CARTESIAN_POINT('Origin',(0.,0.,0.));
#35473=CARTESIAN_POINT('',(0.169,0.29271658647914,0.));
#35474=CARTESIAN_POINT('',(0.149846033266815,0.162485892386646,0.));
#35475=CARTESIAN_POINT('',(0.179094400846393,0.300707824283758,0.));
#35476=CARTESIAN_POINT('',(0.175112028053804,0.297555176742166,0.));
#35477=CARTESIAN_POINT('',(0.221319030845725,0.27114182006011,0.));
#35478=CARTESIAN_POINT('Origin',(0.,0.,0.));
#35479=CARTESIAN_POINT('',(0.21726221207405,0.258923021774215,0.));
#35480=CARTESIAN_POINT('',(0.185136525284291,0.162163144448502,0.));
#35481=CARTESIAN_POINT('',(0.228590920171666,0.265039980408751,0.));
#35482=CARTESIAN_POINT('',(0.238884451429285,0.27059799323454,2.77555756156289E-17));
#35483=CARTESIAN_POINT('',(0.265039980408751,0.228590920171666,0.));
#35484=CARTESIAN_POINT('Origin',(0.,0.,0.));
#35485=CARTESIAN_POINT('',(0.258923021774215,0.21726221207405,0.));
#35486=CARTESIAN_POINT('',(0.223787731003033,0.152191075116504,0.));
#35487=CARTESIAN_POINT('',(0.27114182006011,0.221319030845725,0.));
#35488=CARTESIAN_POINT('',(0.293726415855352,0.228817445176584,0.));
#35489=CARTESIAN_POINT('',(0.300707824283758,0.179094400846393,0.));
#35490=CARTESIAN_POINT('Origin',(0.,0.,0.));
#35491=CARTESIAN_POINT('',(0.29271658647914,0.169,0.));
#35492=CARTESIAN_POINT('',(0.262628621977131,0.130993375524403,0.));
#35493=CARTESIAN_POINT('',(0.305454212950408,0.170873414523285,0.));
#35494=CARTESIAN_POINT('',(0.335974944875694,0.175362318525856,0.));
#35495=CARTESIAN_POINT('',(0.327238813083405,0.124156188777542,0.));
#35496=CARTESIAN_POINT('Origin',(0.,0.,0.));
#35497=CARTESIAN_POINT('',(0.317616105825637,0.115602808444076,0.));
#35498=CARTESIAN_POINT('',(0.297960057644542,0.098131045930453,-2.77555756156289E-17));
#35499=CARTESIAN_POINT('',(0.330485534147499,0.115235895966675,0.));
#35500=CARTESIAN_POINT('',(0.363112879001896,0.114305677496039,-2.77555756156289E-17));
#35501=CARTESIAN_POINT('',(0.343826816138341,0.0654455537387478,0.));
#35502=CARTESIAN_POINT('Origin',(0.,0.,0.));
#35503=CARTESIAN_POINT('',(0.332865020518126,0.0586930840514224,0.));
#35504=CARTESIAN_POINT('',(0.325971007974539,0.0544463700697488,2.77555756156289E-17));
#35505=CARTESIAN_POINT('',(0.345475219623267,0.0560969930232949,0.));
#35506=CARTESIAN_POINT('',(0.37399413172781,0.050225738237446,0.));
#35507=CARTESIAN_POINT('',(0.349967815369678,0.00474638866665024,0.));
#35508=CARTESIAN_POINT('Origin',(0.,0.,0.));
#35509=CARTESIAN_POINT('',(0.338,0.,0.));
#35510=CARTESIAN_POINT('',(0.343184532857686,0.00205616541009999,0.));
#35511=CARTESIAN_POINT('',(0.349967815369678,-0.00474638866665023,0.));
#35512=CARTESIAN_POINT('',(0.368917292134828,-0.012261676877474,0.));
#35513=CARTESIAN_POINT('',(0.345475219623267,-0.0560969930232949,0.));
#35514=CARTESIAN_POINT('Origin',(0.,0.,0.));
#35515=CARTESIAN_POINT('',(0.332865020518126,-0.0586930840514225,0.));
#35516=CARTESIAN_POINT('',(0.346880142416816,-0.0558077582991534,0.));
#35517=CARTESIAN_POINT('',(0.343826816138341,-0.0654455537387478,0.));
#35518=CARTESIAN_POINT('',(0.349540660348596,-0.0689652836410913,2.77555756156289E-17));
#35519=CARTESIAN_POINT('Origin',(0.,0.,0.));
#35520=CARTESIAN_POINT('Origin',(0.,0.,0.201));
#35521=CARTESIAN_POINT('',(0.0866025403784438,-0.15,0.201));
#35522=CARTESIAN_POINT('',(-0.086602540378444,-0.15,0.201));
#35523=CARTESIAN_POINT('',(0.0433012701892219,-0.15,0.201));
#35524=CARTESIAN_POINT('Origin',(0.,0.,0.201));
#35525=CARTESIAN_POINT('Origin',(0.,0.,0.201));
#35526=CARTESIAN_POINT('',(-0.173205080756888,8.32667268468867E-17,0.201));
#35527=CARTESIAN_POINT('',(-0.108253175473055,-0.1125,0.201));
#35528=CARTESIAN_POINT('Origin',(0.,0.,0.201));
#35529=CARTESIAN_POINT('Origin',(0.,0.,0.201));
#35530=CARTESIAN_POINT('',(-0.0866025403784438,0.15,0.201));
#35531=CARTESIAN_POINT('',(-0.151554445662277,0.0375,0.201));
#35532=CARTESIAN_POINT('Origin',(0.,0.,0.201));
#35533=CARTESIAN_POINT('Origin',(0.,0.,0.201));
#35534=CARTESIAN_POINT('',(0.0866025403784439,0.15,0.201));
#35535=CARTESIAN_POINT('',(-0.0433012701892219,0.15,0.201));
#35536=CARTESIAN_POINT('Origin',(0.,0.,0.201));
#35537=CARTESIAN_POINT('Origin',(0.,0.,0.201));
#35538=CARTESIAN_POINT('',(0.173205080756888,0.,0.201));
#35539=CARTESIAN_POINT('',(0.108253175473055,0.1125,0.201));
#35540=CARTESIAN_POINT('Origin',(0.,0.,0.201));
#35541=CARTESIAN_POINT('Origin',(0.,0.,0.201));
#35542=CARTESIAN_POINT('',(0.151554445662277,-0.0375,0.201));
#35543=CARTESIAN_POINT('Origin',(0.,0.,0.201));
#35544=CARTESIAN_POINT('Origin',(0.,0.,0.148538475772934));
#35545=CARTESIAN_POINT('',(0.,0.,0.0960769515458673));
#35546=CARTESIAN_POINT('',(-0.171554298747513,-2.1009342284111E-17,0.2));
#35547=CARTESIAN_POINT('',(-0.0866025403784439,-1.06057523872491E-17,0.148538475772934));
#35548=CARTESIAN_POINT('',(-0.171529756258877,-0.0029017471497188,0.2));
#35549=CARTESIAN_POINT('Origin',(0.,0.,0.2));
#35550=CARTESIAN_POINT('Ctrl Pts',(-0.173205080756888,-1.52655665885959E-16,
0.201));
#35551=CARTESIAN_POINT('Ctrl Pts',(-0.172363407600995,-0.00145782066937349,
0.200490136704233));
#35552=CARTESIAN_POINT('Ctrl Pts',(-0.171529756258877,-0.00290174714971882,
0.2));
#35553=CARTESIAN_POINT('',(-0.0882778648764544,-0.147098252850281,0.2));
#35554=CARTESIAN_POINT('Ctrl Pts',(-0.0882778648764544,-0.147098252850281,
0.2));
#35555=CARTESIAN_POINT('Ctrl Pts',(-0.0874442135343418,-0.148542179330618,
0.20049013670423));
#35556=CARTESIAN_POINT('Ctrl Pts',(-0.0866025403784441,-0.15,0.201));
#35557=CARTESIAN_POINT('',(-0.0832518913824231,-0.15,0.2));
#35558=CARTESIAN_POINT('Origin',(0.,0.,0.2));
#35559=CARTESIAN_POINT('Ctrl Pts',(-0.0866025403784439,-0.15,0.201));
#35560=CARTESIAN_POINT('Ctrl Pts',(-0.0849191940666532,-0.15,0.200490136704232));
#35561=CARTESIAN_POINT('Ctrl Pts',(-0.0832518913824231,-0.15,0.2));
#35562=CARTESIAN_POINT('',(0.0832518913824231,-0.15,0.2));
#35563=CARTESIAN_POINT('Ctrl Pts',(0.0832518913824231,-0.15,0.2));
#35564=CARTESIAN_POINT('Ctrl Pts',(0.084919194066652,-0.15,0.200490136704231));
#35565=CARTESIAN_POINT('Ctrl Pts',(0.0866025403784438,-0.15,0.201));
#35566=CARTESIAN_POINT('',(0.0882778648764543,-0.147098252850281,0.2));
#35567=CARTESIAN_POINT('Origin',(0.,0.,0.2));
#35568=CARTESIAN_POINT('Ctrl Pts',(0.0866025403784439,-0.15,0.201));
#35569=CARTESIAN_POINT('Ctrl Pts',(0.0874442135343394,-0.148542179330622,
0.200490136704231));
#35570=CARTESIAN_POINT('Ctrl Pts',(0.0882778648764543,-0.147098252850281,
0.2));
#35571=CARTESIAN_POINT('',(0.171529756258877,-0.00290174714971884,0.2));
#35572=CARTESIAN_POINT('Ctrl Pts',(0.171529756258877,-0.00290174714971883,
0.2));
#35573=CARTESIAN_POINT('Ctrl Pts',(0.172363407600991,-0.00145782066937972,
0.200490136704231));
#35574=CARTESIAN_POINT('Ctrl Pts',(0.173205080756888,-1.38777878078145E-17,
0.201));
#35575=CARTESIAN_POINT('',(0.171529756258877,0.00290174714971882,0.2));
#35576=CARTESIAN_POINT('Origin',(0.,0.,0.2));
#35577=CARTESIAN_POINT('Ctrl Pts',(0.173205080756888,-4.16333634234434E-17,
0.201));
#35578=CARTESIAN_POINT('Ctrl Pts',(0.172363407600995,0.00145782066937251,
0.200490136704233));
#35579=CARTESIAN_POINT('Ctrl Pts',(0.171529756258877,0.00290174714971887,
0.2));
#35580=CARTESIAN_POINT('',(0.0882778648764543,0.147098252850281,0.2));
#35581=CARTESIAN_POINT('Ctrl Pts',(0.0882778648764543,0.147098252850281,
0.2));
#35582=CARTESIAN_POINT('Ctrl Pts',(0.0874442135343416,0.148542179330618,
0.20049013670423));
#35583=CARTESIAN_POINT('Ctrl Pts',(0.0866025403784439,0.15,0.201));
#35584=CARTESIAN_POINT('',(0.0832518913824231,0.15,0.2));
#35585=CARTESIAN_POINT('Origin',(0.,0.,0.2));
#35586=CARTESIAN_POINT('Ctrl Pts',(0.0866025403784438,0.15,0.201));
#35587=CARTESIAN_POINT('Ctrl Pts',(0.0849191940666536,0.15,0.200490136704232));
#35588=CARTESIAN_POINT('Ctrl Pts',(0.0832518913824231,0.15,0.2));
#35589=CARTESIAN_POINT('',(-0.0832518913824231,0.15,0.2));
#35590=CARTESIAN_POINT('Ctrl Pts',(-0.0832518913824231,0.15,0.2));
#35591=CARTESIAN_POINT('Ctrl Pts',(-0.0849191940666509,0.15,0.200490136704231));
#35592=CARTESIAN_POINT('Ctrl Pts',(-0.0866025403784438,0.15,0.201));
#35593=CARTESIAN_POINT('',(-0.0882778648764542,0.147098252850281,0.2));
#35594=CARTESIAN_POINT('Origin',(0.,0.,0.2));
#35595=CARTESIAN_POINT('Ctrl Pts',(-0.0866025403784439,0.15,0.201));
#35596=CARTESIAN_POINT('Ctrl Pts',(-0.0874442135343377,0.148542179330625,
0.200490136704232));
#35597=CARTESIAN_POINT('Ctrl Pts',(-0.0882778648764542,0.147098252850281,
0.2));
#35598=CARTESIAN_POINT('',(-0.171529756258877,0.00290174714971888,0.2));
#35599=CARTESIAN_POINT('Ctrl Pts',(-0.171529756258877,0.00290174714971886,
0.2));
#35600=CARTESIAN_POINT('Ctrl Pts',(-0.172363407600993,0.00145782066937643,
0.200490136704232));
#35601=CARTESIAN_POINT('Ctrl Pts',(-0.173205080756888,1.52655665885959E-16,
0.201));
#35602=CARTESIAN_POINT('Origin',(0.,0.,0.2));
#35603=CARTESIAN_POINT('Origin',(-0.173205080756888,2.77555756156289E-17,
0.4));
#35604=CARTESIAN_POINT('',(-0.0866025403784438,0.15,0.4));
#35605=CARTESIAN_POINT('',(-0.0866025403784438,0.15,0.4));
#35606=CARTESIAN_POINT('',(-0.173205080756888,2.12115047744981E-17,0.4));
#35607=CARTESIAN_POINT('',(-0.151554445662277,0.0375,0.4));
#35608=CARTESIAN_POINT('',(-0.173205080756888,2.12115047744981E-17,0.4));
#35609=CARTESIAN_POINT('Origin',(-0.173205080756888,2.77555756156289E-17,
0.4));
#35610=CARTESIAN_POINT('',(-0.173205080756888,2.77555756156289E-17,0.2));
#35611=CARTESIAN_POINT('',(-0.173205080756888,2.12115047744981E-17,0.4));
#35612=CARTESIAN_POINT('',(-0.0866025403784438,0.15,0.2));
#35613=CARTESIAN_POINT('Origin',(-0.0866025403784438,0.15,0.4));
#35614=CARTESIAN_POINT('',(0.0866025403784439,0.15,0.4));
#35615=CARTESIAN_POINT('',(0.0866025403784439,0.15,0.4));
#35616=CARTESIAN_POINT('',(-0.0433012701892219,0.15,0.4));
#35617=CARTESIAN_POINT('Origin',(-0.0866025403784438,0.15,0.4));
#35618=CARTESIAN_POINT('',(0.0866025403784439,0.15,0.2));
#35619=CARTESIAN_POINT('',(0.0866025403784439,0.15,0.2));
#35620=CARTESIAN_POINT('',(0.0866025403784439,0.15,0.4));
#35621=CARTESIAN_POINT('Origin',(-0.0866025403784438,0.15,0.4));
#35622=CARTESIAN_POINT('',(-0.0866025403784438,0.15,0.2));
#35623=CARTESIAN_POINT('',(-0.0866025403784438,0.15,0.4));
#35624=CARTESIAN_POINT('',(0.0866025403784439,0.15,0.2));
#35625=CARTESIAN_POINT('Origin',(-0.0866025403784439,-0.15,0.4));
#35626=CARTESIAN_POINT('',(-0.0866025403784439,-0.15,0.4));
#35627=CARTESIAN_POINT('',(-0.108253175473055,-0.1125,0.4));
#35628=CARTESIAN_POINT('',(-0.0866025403784439,-0.15,0.4));
#35629=CARTESIAN_POINT('Origin',(-0.0866025403784439,-0.15,0.4));
#35630=CARTESIAN_POINT('',(-0.0866025403784439,-0.15,0.2));
#35631=CARTESIAN_POINT('',(-0.0866025403784439,-0.15,0.4));
#35632=CARTESIAN_POINT('',(-0.173205080756888,2.12115047744981E-17,0.2));
#35633=CARTESIAN_POINT('Origin',(0.0866025403784439,0.15,0.4));
#35634=CARTESIAN_POINT('',(0.173205080756888,0.,0.4));
#35635=CARTESIAN_POINT('',(0.173205080756888,0.,0.4));
#35636=CARTESIAN_POINT('',(0.108253175473055,0.1125,0.4));
#35637=CARTESIAN_POINT('Origin',(0.0866025403784439,0.15,0.4));
#35638=CARTESIAN_POINT('',(0.173205080756888,0.,0.2));
#35639=CARTESIAN_POINT('',(0.173205080756888,0.,0.2));
#35640=CARTESIAN_POINT('',(0.173205080756888,0.,0.4));
#35641=CARTESIAN_POINT('Origin',(0.0866025403784439,0.15,0.4));
#35642=CARTESIAN_POINT('',(0.173205080756888,0.,0.2));
#35643=CARTESIAN_POINT('Origin',(0.,2.77555756156289E-17,0.2));
#35644=CARTESIAN_POINT('',(-0.0866025403784438,0.15,0.2));
#35645=CARTESIAN_POINT('Origin',(0.,2.77555756156289E-17,0.2));
#35646=CARTESIAN_POINT('Origin',(0.,2.77555756156289E-17,0.2));
#35647=CARTESIAN_POINT('',(0.0866025403784439,-0.15,0.2));
#35648=CARTESIAN_POINT('Origin',(0.,2.77555756156289E-17,0.2));
#35649=CARTESIAN_POINT('',(0.0866025403784439,-0.15,0.2));
#35650=CARTESIAN_POINT('',(-0.0866025403784439,-0.15,0.2));
#35651=CARTESIAN_POINT('',(0.0866025403784439,-0.15,0.2));
#35652=CARTESIAN_POINT('Origin',(0.,2.77555756156289E-17,0.2));
#35653=CARTESIAN_POINT('',(-0.0866025403784439,-0.15,0.2));
#35654=CARTESIAN_POINT('Origin',(0.,2.77555756156289E-17,0.2));
#35655=CARTESIAN_POINT('',(-0.173205080756888,2.12115047744981E-17,0.2));
#35656=CARTESIAN_POINT('Origin',(0.173205080756888,0.,0.4));
#35657=CARTESIAN_POINT('',(0.0866025403784439,-0.15,0.4));
#35658=CARTESIAN_POINT('',(0.0866025403784439,-0.15,0.4));
#35659=CARTESIAN_POINT('',(0.151554445662277,-0.0375,0.4));
#35660=CARTESIAN_POINT('Origin',(0.173205080756888,0.,0.4));
#35661=CARTESIAN_POINT('',(0.0866025403784439,-0.15,0.4));
#35662=CARTESIAN_POINT('Origin',(0.173205080756888,0.,0.4));
#35663=CARTESIAN_POINT('Origin',(0.0866025403784439,-0.15,0.4));
#35664=CARTESIAN_POINT('Origin',(0.0866025403784439,-0.15,0.4));
#35665=CARTESIAN_POINT('',(0.0433012701892219,-0.15,0.4));
#35666=CARTESIAN_POINT('Origin',(-0.173205080756888,2.77555756156289E-17,
0.4));
#35667=CARTESIAN_POINT('Origin',(-0.0866025403784439,-0.15,0.4));
#35668=CARTESIAN_POINT('Origin',(0.0866025403784439,-0.15,0.4));
#35669=CARTESIAN_POINT('Origin',(0.317616105825637,-0.115602808444076,0.4));
#35670=CARTESIAN_POINT('',(0.317616105825637,-0.115602808444076,0.372));
#35671=CARTESIAN_POINT('',(0.330485534147499,-0.115235895966675,0.36));
#35672=CARTESIAN_POINT('Ctrl Pts',(0.317616105825637,-0.115602808444076,
0.372));
#35673=CARTESIAN_POINT('Ctrl Pts',(0.32393858660004,-0.115422552023493,
0.366120462798036));
#35674=CARTESIAN_POINT('Ctrl Pts',(0.330485534147499,-0.115235895966675,
0.36));
#35675=CARTESIAN_POINT('',(0.317616105825637,-0.115602808444076,0.4));
#35676=CARTESIAN_POINT('',(0.330485534147499,-0.115235895966675,0.18));
#35677=CARTESIAN_POINT('Origin',(0.358996892846452,-0.152385140110817,0.4));
#35678=CARTESIAN_POINT('',(0.327238813083405,-0.124156188777542,0.36));
#35679=CARTESIAN_POINT('Ctrl Pts',(0.327238813083405,-0.124156188777541,
0.36));
#35680=CARTESIAN_POINT('Ctrl Pts',(0.322343540495881,-0.119804905177671,
0.366120462798032));
#35681=CARTESIAN_POINT('Ctrl Pts',(0.317616105825637,-0.115602808444076,
0.372));
#35682=CARTESIAN_POINT('',(0.327238813083405,-0.124156188777542,0.18));
#35683=CARTESIAN_POINT('Origin',(0.258923021774215,-0.21726221207405,0.4));
#35684=CARTESIAN_POINT('',(0.258923021774215,-0.21726221207405,0.372));
#35685=CARTESIAN_POINT('',(0.27114182006011,-0.221319030845725,0.36));
#35686=CARTESIAN_POINT('Ctrl Pts',(0.258923021774215,-0.21726221207405,
0.372));
#35687=CARTESIAN_POINT('Ctrl Pts',(0.264925861629792,-0.219255242226416,
0.36612046279803));
#35688=CARTESIAN_POINT('Ctrl Pts',(0.27114182006011,-0.221319030845725,
0.36));
#35689=CARTESIAN_POINT('',(0.258923021774215,-0.21726221207405,0.4));
#35690=CARTESIAN_POINT('',(0.27114182006011,-0.221319030845725,0.18));
#35691=CARTESIAN_POINT('Origin',(0.285227943631477,-0.265979360424374,0.4));
#35692=CARTESIAN_POINT('',(0.265039980408751,-0.228590920171666,0.36));
#35693=CARTESIAN_POINT('Ctrl Pts',(0.265039980408751,-0.228590920171666,
0.36));
#35694=CARTESIAN_POINT('Ctrl Pts',(0.261928155521996,-0.222827769249915,
0.366120462798034));
#35695=CARTESIAN_POINT('Ctrl Pts',(0.258923021774215,-0.21726221207405,
0.372));
#35696=CARTESIAN_POINT('',(0.265039980408751,-0.228590920171666,0.18));
#35697=CARTESIAN_POINT('Origin',(0.169,-0.29271658647914,0.4));
#35698=CARTESIAN_POINT('',(0.169,-0.29271658647914,0.372));
#35699=CARTESIAN_POINT('',(0.179094400846393,-0.300707824283758,0.36));
#35700=CARTESIAN_POINT('Ctrl Pts',(0.169,-0.29271658647914,0.372));
#35701=CARTESIAN_POINT('Ctrl Pts',(0.173959167857677,-0.296642514354085,
0.366120462798034));
#35702=CARTESIAN_POINT('Ctrl Pts',(0.179094400846393,-0.300707824283758,
0.36));
#35703=CARTESIAN_POINT('',(0.169,-0.29271658647914,0.4));
#35704=CARTESIAN_POINT('',(0.179094400846393,-0.300707824283758,0.18));
#35705=CARTESIAN_POINT('Origin',(0.177056294898423,-0.347492544433464,0.4));
#35706=CARTESIAN_POINT('',(0.170873414523285,-0.305454212950408,0.36));
#35707=CARTESIAN_POINT('Ctrl Pts',(0.170873414523285,-0.305454212950408,
0.36));
#35708=CARTESIAN_POINT('Ctrl Pts',(0.169920369344289,-0.298974315762995,
0.366120462798031));
#35709=CARTESIAN_POINT('Ctrl Pts',(0.169,-0.29271658647914,0.372));
#35710=CARTESIAN_POINT('',(0.170873414523285,-0.305454212950408,0.18));
#35711=CARTESIAN_POINT('Origin',(0.0586930840514223,-0.332865020518126,
0.4));
#35712=CARTESIAN_POINT('',(0.0586930840514223,-0.332865020518126,0.372));
#35713=CARTESIAN_POINT('',(0.0654455537387477,-0.343826816138341,0.36));
#35714=CARTESIAN_POINT('Ctrl Pts',(0.0586930840514223,-0.332865020518126,
0.372));
#35715=CARTESIAN_POINT('Ctrl Pts',(0.062010431078043,-0.338250321273404,
0.366120462798039));
#35716=CARTESIAN_POINT('Ctrl Pts',(0.0654455537387476,-0.343826816138341,
0.36));
#35717=CARTESIAN_POINT('',(0.0586930840514223,-0.332865020518126,0.4));
#35718=CARTESIAN_POINT('',(0.0654455537387477,-0.343826816138341,0.18));
#35719=CARTESIAN_POINT('Origin',(0.0475290439280076,-0.387092999140116,
0.4));
#35720=CARTESIAN_POINT('',(0.0560969930232948,-0.345475219623267,0.36));
#35721=CARTESIAN_POINT('Ctrl Pts',(0.0560969930232948,-0.345475219623267,
0.36));
#35722=CARTESIAN_POINT('Ctrl Pts',(0.0574176788660909,-0.339060147404089,
0.36612046279803));
#35723=CARTESIAN_POINT('Ctrl Pts',(0.0586930840514223,-0.332865020518126,
0.372));
#35724=CARTESIAN_POINT('',(0.0560969930232948,-0.345475219623267,0.18));
#35725=CARTESIAN_POINT('Origin',(-0.0586930840514224,-0.332865020518126,
0.4));
#35726=CARTESIAN_POINT('',(-0.0586930840514225,-0.332865020518126,0.372));
#35727=CARTESIAN_POINT('',(-0.0560969930232949,-0.345475219623267,0.36));
#35728=CARTESIAN_POINT('Ctrl Pts',(-0.0586930840514225,-0.332865020518126,
0.372));
#35729=CARTESIAN_POINT('Ctrl Pts',(-0.0574176788660934,-0.339060147404077,
0.366120462798041));
#35730=CARTESIAN_POINT('Ctrl Pts',(-0.0560969930232949,-0.345475219623267,
0.36));
#35731=CARTESIAN_POINT('',(-0.0586930840514224,-0.332865020518126,0.4));
#35732=CARTESIAN_POINT('',(-0.0560969930232949,-0.345475219623267,0.18));
#35733=CARTESIAN_POINT('Origin',(-0.0877309111941074,-0.380004325266242,
0.4));
#35734=CARTESIAN_POINT('',(-0.0654455537387478,-0.343826816138341,0.36));
#35735=CARTESIAN_POINT('Ctrl Pts',(-0.0654455537387477,-0.343826816138341,
0.36));
#35736=CARTESIAN_POINT('Ctrl Pts',(-0.062010431078045,-0.338250321273407,
0.366120462798035));
#35737=CARTESIAN_POINT('Ctrl Pts',(-0.0586930840514225,-0.332865020518126,
0.372));
#35738=CARTESIAN_POINT('',(-0.0654455537387478,-0.343826816138341,0.18));
#35739=CARTESIAN_POINT('Origin',(-0.169,-0.29271658647914,0.4));
#35740=CARTESIAN_POINT('',(-0.169,-0.29271658647914,0.372));
#35741=CARTESIAN_POINT('',(-0.170873414523286,-0.305454212950408,0.36));
#35742=CARTESIAN_POINT('Ctrl Pts',(-0.169,-0.29271658647914,0.372));
#35743=CARTESIAN_POINT('Ctrl Pts',(-0.16992036934429,-0.298974315762997,
0.36612046279803));
#35744=CARTESIAN_POINT('Ctrl Pts',(-0.170873414523285,-0.305454212950408,
0.36));
#35745=CARTESIAN_POINT('',(-0.169,-0.29271658647914,0.4));
#35746=CARTESIAN_POINT('',(-0.170873414523286,-0.305454212950408,0.18));
#35747=CARTESIAN_POINT('Origin',(-0.212409223655861,-0.327081521498715,
0.4));
#35748=CARTESIAN_POINT('',(-0.179094400846393,-0.300707824283758,0.36));
#35749=CARTESIAN_POINT('Ctrl Pts',(-0.179094400846393,-0.300707824283758,
0.36));
#35750=CARTESIAN_POINT('Ctrl Pts',(-0.173959167857676,-0.296642514354083,
0.366120462798036));
#35751=CARTESIAN_POINT('Ctrl Pts',(-0.169,-0.29271658647914,0.372));
#35752=CARTESIAN_POINT('',(-0.179094400846393,-0.300707824283758,0.18));
#35753=CARTESIAN_POINT('Origin',(-0.258923021774215,-0.21726221207405,0.4));
#35754=CARTESIAN_POINT('',(-0.258923021774215,-0.21726221207405,0.372));
#35755=CARTESIAN_POINT('',(-0.265039980408751,-0.228590920171666,0.36));
#35756=CARTESIAN_POINT('Ctrl Pts',(-0.258923021774215,-0.21726221207405,
0.372));
#35757=CARTESIAN_POINT('Ctrl Pts',(-0.261928155521997,-0.222827769249916,
0.366120462798033));
#35758=CARTESIAN_POINT('Ctrl Pts',(-0.265039980408751,-0.228590920171666,
0.36));
#35759=CARTESIAN_POINT('',(-0.258923021774215,-0.21726221207405,0.4));
#35760=CARTESIAN_POINT('',(-0.265039980408751,-0.228590920171666,0.18));
#35761=CARTESIAN_POINT('Origin',(-0.311467848918444,-0.234707859029299,
0.4));
#35762=CARTESIAN_POINT('',(-0.27114182006011,-0.221319030845725,0.36));
#35763=CARTESIAN_POINT('Ctrl Pts',(-0.27114182006011,-0.221319030845725,
0.36));
#35764=CARTESIAN_POINT('Ctrl Pts',(-0.264925861629788,-0.219255242226415,
0.366120462798033));
#35765=CARTESIAN_POINT('Ctrl Pts',(-0.258923021774215,-0.21726221207405,
0.372));
#35766=CARTESIAN_POINT('',(-0.27114182006011,-0.221319030845725,0.18));
#35767=CARTESIAN_POINT('Origin',(-0.317616105825637,-0.115602808444076,
0.4));
#35768=CARTESIAN_POINT('',(-0.317616105825637,-0.115602808444076,0.372));
#35769=CARTESIAN_POINT('',(-0.327238813083405,-0.124156188777542,0.36));
#35770=CARTESIAN_POINT('Ctrl Pts',(-0.317616105825637,-0.115602808444076,
0.372));
#35771=CARTESIAN_POINT('Ctrl Pts',(-0.322343540495879,-0.119804905177669,
0.366120462798034));
#35772=CARTESIAN_POINT('Ctrl Pts',(-0.327238813083405,-0.124156188777541,
0.36));
#35773=CARTESIAN_POINT('',(-0.317616105825637,-0.115602808444076,0.4));
#35774=CARTESIAN_POINT('',(-0.327238813083405,-0.124156188777542,0.18));
#35775=CARTESIAN_POINT('Origin',(-0.372958854825584,-0.114024964841867,
0.4));
#35776=CARTESIAN_POINT('',(-0.330485534147499,-0.115235895966675,0.36));
#35777=CARTESIAN_POINT('Ctrl Pts',(-0.330485534147499,-0.115235895966675,
0.36));
#35778=CARTESIAN_POINT('Ctrl Pts',(-0.32393858660004,-0.115422552023493,
0.366120462798036));
#35779=CARTESIAN_POINT('Ctrl Pts',(-0.317616105825637,-0.115602808444076,
0.372));
#35780=CARTESIAN_POINT('',(-0.330485534147499,-0.115235895966675,0.18));
#35781=CARTESIAN_POINT('Origin',(-0.338,4.13930618111805E-17,0.4));
#35782=CARTESIAN_POINT('',(-0.338,4.13930618111805E-17,0.372));
#35783=CARTESIAN_POINT('',(-0.349967815369678,-0.0047463886666502,0.36));
#35784=CARTESIAN_POINT('Ctrl Pts',(-0.338,4.13930618111805E-17,0.372));
#35785=CARTESIAN_POINT('Ctrl Pts',(-0.343879537201965,-0.00233180140890689,
0.366120462798035));
#35786=CARTESIAN_POINT('Ctrl Pts',(-0.349967815369678,-0.00474638866665013,
0.36));
#35787=CARTESIAN_POINT('',(-0.338,4.13930618111805E-17,0.4));
#35788=CARTESIAN_POINT('',(-0.349967815369678,-0.0047463886666502,0.18));
#35789=CARTESIAN_POINT('Origin',(-0.389465518554284,0.0204110229347481,
0.4));
#35790=CARTESIAN_POINT('',(-0.349967815369678,0.00474638866665025,0.36));
#35791=CARTESIAN_POINT('Ctrl Pts',(-0.349967815369678,0.00474638866665024,
0.36));
#35792=CARTESIAN_POINT('Ctrl Pts',(-0.343879537201956,0.00233180140890372,
0.366120462798043));
#35793=CARTESIAN_POINT('Ctrl Pts',(-0.338,4.13930618111805E-17,0.372));
#35794=CARTESIAN_POINT('',(-0.349967815369678,0.00474638866665025,0.18));
#35795=CARTESIAN_POINT('Origin',(-0.332865020518126,0.0586930840514224,
0.4));
#35796=CARTESIAN_POINT('',(-0.332865020518126,0.0586930840514224,0.372));
#35797=CARTESIAN_POINT('',(-0.345475219623267,0.0560969930232949,0.36));
#35798=CARTESIAN_POINT('Ctrl Pts',(-0.332865020518126,0.0586930840514224,
0.372));
#35799=CARTESIAN_POINT('Ctrl Pts',(-0.33906014740408,0.0574176788660928,
0.366120462798038));
#35800=CARTESIAN_POINT('Ctrl Pts',(-0.345475219623267,0.0560969930232949,
0.36));
#35801=CARTESIAN_POINT('',(-0.332865020518126,0.0586930840514224,0.4));
#35802=CARTESIAN_POINT('',(-0.345475219623267,0.0560969930232949,0.18));
#35803=CARTESIAN_POINT('Origin',(-0.380004325266242,0.0877309111941074,
0.4));
#35804=CARTESIAN_POINT('',(-0.343826816138341,0.0654455537387477,0.36));
#35805=CARTESIAN_POINT('Ctrl Pts',(-0.343826816138341,0.0654455537387478,
0.36));
#35806=CARTESIAN_POINT('Ctrl Pts',(-0.338250321273404,0.0620104310780433,
0.366120462798038));
#35807=CARTESIAN_POINT('Ctrl Pts',(-0.332865020518126,0.0586930840514224,
0.372));
#35808=CARTESIAN_POINT('',(-0.343826816138341,0.0654455537387477,0.18));
#35809=CARTESIAN_POINT('Origin',(-0.29271658647914,0.169,0.4));
#35810=CARTESIAN_POINT('',(-0.29271658647914,0.169,0.372));
#35811=CARTESIAN_POINT('',(-0.305454212950408,0.170873414523285,0.36));
#35812=CARTESIAN_POINT('Ctrl Pts',(-0.29271658647914,0.169,0.372));
#35813=CARTESIAN_POINT('Ctrl Pts',(-0.298974315762988,0.169920369344288,
0.366120462798038));
#35814=CARTESIAN_POINT('Ctrl Pts',(-0.305454212950408,0.170873414523285,
0.36));
#35815=CARTESIAN_POINT('',(-0.29271658647914,0.169,0.4));
#35816=CARTESIAN_POINT('',(-0.305454212950408,0.170873414523285,0.18));
#35817=CARTESIAN_POINT('Origin',(-0.327081521498715,0.212409223655861,0.4));
#35818=CARTESIAN_POINT('',(-0.300707824283758,0.179094400846393,0.36));
#35819=CARTESIAN_POINT('Ctrl Pts',(-0.300707824283758,0.179094400846393,
0.36));
#35820=CARTESIAN_POINT('Ctrl Pts',(-0.296642514354079,0.17395916785767,
0.366120462798042));
#35821=CARTESIAN_POINT('Ctrl Pts',(-0.29271658647914,0.169,0.372));
#35822=CARTESIAN_POINT('',(-0.300707824283758,0.179094400846393,0.18));
#35823=CARTESIAN_POINT('Origin',(-0.21726221207405,0.258923021774215,0.4));
#35824=CARTESIAN_POINT('',(-0.21726221207405,0.258923021774215,0.372));
#35825=CARTESIAN_POINT('',(-0.228590920171666,0.265039980408751,0.36));
#35826=CARTESIAN_POINT('Ctrl Pts',(-0.21726221207405,0.258923021774215,
0.372));
#35827=CARTESIAN_POINT('Ctrl Pts',(-0.222827769249908,0.261928155521993,
0.366120462798042));
#35828=CARTESIAN_POINT('Ctrl Pts',(-0.228590920171666,0.265039980408751,
0.36));
#35829=CARTESIAN_POINT('',(-0.21726221207405,0.258923021774215,0.4));
#35830=CARTESIAN_POINT('',(-0.228590920171666,0.265039980408751,0.18));
#35831=CARTESIAN_POINT('Origin',(-0.234707859029299,0.311467848918444,0.4));
#35832=CARTESIAN_POINT('',(-0.221319030845725,0.27114182006011,0.36));
#35833=CARTESIAN_POINT('Ctrl Pts',(-0.221319030845725,0.27114182006011,
0.36));
#35834=CARTESIAN_POINT('Ctrl Pts',(-0.219255242226413,0.264925861629782,
0.366120462798039));
#35835=CARTESIAN_POINT('Ctrl Pts',(-0.21726221207405,0.258923021774215,
0.372));
#35836=CARTESIAN_POINT('',(-0.221319030845725,0.27114182006011,0.18));
#35837=CARTESIAN_POINT('Origin',(-0.115602808444076,0.317616105825637,0.4));
#35838=CARTESIAN_POINT('',(-0.115602808444076,0.317616105825637,0.372));
#35839=CARTESIAN_POINT('',(-0.124156188777542,0.327238813083405,0.36));
#35840=CARTESIAN_POINT('Ctrl Pts',(-0.115602808444076,0.317616105825637,
0.372));
#35841=CARTESIAN_POINT('Ctrl Pts',(-0.119804905177669,0.322343540495879,
0.366120462798034));
#35842=CARTESIAN_POINT('Ctrl Pts',(-0.124156188777542,0.327238813083405,
0.36));
#35843=CARTESIAN_POINT('',(-0.115602808444076,0.317616105825637,0.4));
#35844=CARTESIAN_POINT('',(-0.124156188777542,0.327238813083405,0.18));
#35845=CARTESIAN_POINT('Origin',(-0.114024964841867,0.372958854825584,0.4));
#35846=CARTESIAN_POINT('',(-0.115235895966675,0.330485534147499,0.36));
#35847=CARTESIAN_POINT('Ctrl Pts',(-0.115235895966675,0.330485534147499,
0.36));
#35848=CARTESIAN_POINT('Ctrl Pts',(-0.115422552023493,0.323938586600039,
0.366120462798037));
#35849=CARTESIAN_POINT('Ctrl Pts',(-0.115602808444076,0.317616105825637,
0.372));
#35850=CARTESIAN_POINT('',(-0.115235895966675,0.330485534147499,0.18));
#35851=CARTESIAN_POINT('Origin',(2.06965309055903E-17,0.338,0.4));
#35852=CARTESIAN_POINT('',(2.06965309055903E-17,0.338,0.372));
#35853=CARTESIAN_POINT('',(-0.00474638866665024,0.349967815369678,0.36));
#35854=CARTESIAN_POINT('Ctrl Pts',(2.06965309055903E-17,0.338,0.372));
#35855=CARTESIAN_POINT('Ctrl Pts',(-0.00233180140890855,0.343879537201969,
0.366120462798031));
#35856=CARTESIAN_POINT('Ctrl Pts',(-0.00474638866665021,0.349967815369678,
0.36));
#35857=CARTESIAN_POINT('',(2.06965309055903E-17,0.338,0.4));
#35858=CARTESIAN_POINT('',(-0.00474638866665024,0.349967815369678,0.18));
#35859=CARTESIAN_POINT('Origin',(0.0204110229347481,0.389465518554284,0.4));
#35860=CARTESIAN_POINT('',(0.00474638866665027,0.349967815369678,0.36));
#35861=CARTESIAN_POINT('Ctrl Pts',(0.00474638866665025,0.349967815369678,
0.36));
#35862=CARTESIAN_POINT('Ctrl Pts',(0.00233180140890579,0.343879537201962,
0.366120462798038));
#35863=CARTESIAN_POINT('Ctrl Pts',(2.06965309055903E-17,0.338,0.372));
#35864=CARTESIAN_POINT('',(0.00474638866665027,0.349967815369678,0.18));
#35865=CARTESIAN_POINT('Origin',(0.115602808444076,0.317616105825637,0.4));
#35866=CARTESIAN_POINT('',(0.115602808444076,0.317616105825637,0.372));
#35867=CARTESIAN_POINT('',(0.115235895966675,0.330485534147499,0.36));
#35868=CARTESIAN_POINT('Ctrl Pts',(0.115602808444076,0.317616105825637,
0.372));
#35869=CARTESIAN_POINT('Ctrl Pts',(0.115422552023493,0.323938586600037,
0.366120462798039));
#35870=CARTESIAN_POINT('Ctrl Pts',(0.115235895966675,0.330485534147499,
0.36));
#35871=CARTESIAN_POINT('',(0.115602808444076,0.317616105825637,0.4));
#35872=CARTESIAN_POINT('',(0.115235895966675,0.330485534147499,0.18));
#35873=CARTESIAN_POINT('Origin',(0.152385140110817,0.358996892846452,0.4));
#35874=CARTESIAN_POINT('',(0.124156188777542,0.327238813083405,0.36));
#35875=CARTESIAN_POINT('Ctrl Pts',(0.124156188777542,0.327238813083405,
0.36));
#35876=CARTESIAN_POINT('Ctrl Pts',(0.119804905177668,0.322343540495878,
0.366120462798036));
#35877=CARTESIAN_POINT('Ctrl Pts',(0.115602808444076,0.317616105825637,
0.372));
#35878=CARTESIAN_POINT('',(0.124156188777542,0.327238813083405,0.18));
#35879=CARTESIAN_POINT('Origin',(0.21726221207405,0.258923021774215,0.4));
#35880=CARTESIAN_POINT('',(0.21726221207405,0.258923021774215,0.372));
#35881=CARTESIAN_POINT('',(0.221319030845725,0.27114182006011,0.36));
#35882=CARTESIAN_POINT('Ctrl Pts',(0.21726221207405,0.258923021774215,0.372));
#35883=CARTESIAN_POINT('Ctrl Pts',(0.219255242226414,0.264925861629787,
0.366120462798035));
#35884=CARTESIAN_POINT('Ctrl Pts',(0.221319030845725,0.27114182006011,0.36));
#35885=CARTESIAN_POINT('',(0.21726221207405,0.258923021774215,0.4));
#35886=CARTESIAN_POINT('',(0.221319030845725,0.27114182006011,0.18));
#35887=CARTESIAN_POINT('Origin',(0.265979360424374,0.285227943631476,0.4));
#35888=CARTESIAN_POINT('',(0.228590920171666,0.265039980408751,0.36));
#35889=CARTESIAN_POINT('Ctrl Pts',(0.228590920171666,0.265039980408751,
0.36));
#35890=CARTESIAN_POINT('Ctrl Pts',(0.222827769249913,0.261928155521995,
0.366120462798037));
#35891=CARTESIAN_POINT('Ctrl Pts',(0.21726221207405,0.258923021774215,0.372));
#35892=CARTESIAN_POINT('',(0.228590920171666,0.265039980408751,0.18));
#35893=CARTESIAN_POINT('Origin',(0.29271658647914,0.169,0.4));
#35894=CARTESIAN_POINT('',(0.29271658647914,0.169,0.372));
#35895=CARTESIAN_POINT('',(0.300707824283758,0.179094400846393,0.36));
#35896=CARTESIAN_POINT('Ctrl Pts',(0.29271658647914,0.169,0.372));
#35897=CARTESIAN_POINT('Ctrl Pts',(0.296642514354088,0.173959167857681,
0.366120462798029));
#35898=CARTESIAN_POINT('Ctrl Pts',(0.300707824283758,0.179094400846393,
0.36));
#35899=CARTESIAN_POINT('',(0.29271658647914,0.169,0.4));
#35900=CARTESIAN_POINT('',(0.300707824283758,0.179094400846393,0.18));
#35901=CARTESIAN_POINT('Origin',(0.347492544433463,0.177056294898423,0.4));
#35902=CARTESIAN_POINT('',(0.305454212950408,0.170873414523285,0.36));
#35903=CARTESIAN_POINT('Ctrl Pts',(0.305454212950408,0.170873414523285,
0.36));
#35904=CARTESIAN_POINT('Ctrl Pts',(0.298974315762989,0.169920369344288,
0.366120462798037));
#35905=CARTESIAN_POINT('Ctrl Pts',(0.29271658647914,0.169,0.372));
#35906=CARTESIAN_POINT('',(0.305454212950408,0.170873414523285,0.18));
#35907=CARTESIAN_POINT('Origin',(0.332865020518126,0.0586930840514224,0.4));
#35908=CARTESIAN_POINT('',(0.332865020518126,0.0586930840514225,0.372));
#35909=CARTESIAN_POINT('',(0.343826816138341,0.0654455537387478,0.36));
#35910=CARTESIAN_POINT('Ctrl Pts',(0.332865020518126,0.0586930840514225,
0.372));
#35911=CARTESIAN_POINT('Ctrl Pts',(0.338250321273409,0.0620104310780461,
0.366120462798033));
#35912=CARTESIAN_POINT('Ctrl Pts',(0.343826816138341,0.0654455537387478,
0.36));
#35913=CARTESIAN_POINT('',(0.332865020518126,0.0586930840514224,0.4));
#35914=CARTESIAN_POINT('',(0.343826816138341,0.0654455537387478,0.18));
#35915=CARTESIAN_POINT('Origin',(0.387092999140116,0.0475290439280075,0.4));
#35916=CARTESIAN_POINT('',(0.345475219623267,0.0560969930232949,0.36));
#35917=CARTESIAN_POINT('Ctrl Pts',(0.345475219623267,0.0560969930232949,
0.36));
#35918=CARTESIAN_POINT('Ctrl Pts',(0.339060147404081,0.0574176788660925,
0.366120462798036));
#35919=CARTESIAN_POINT('Ctrl Pts',(0.332865020518126,0.0586930840514225,
0.372));
#35920=CARTESIAN_POINT('',(0.345475219623267,0.0560969930232949,0.18));
#35921=CARTESIAN_POINT('Origin',(0.317616105825637,0.115602808444076,0.4));
#35922=CARTESIAN_POINT('',(0.317616105825637,0.115602808444076,0.372));
#35923=CARTESIAN_POINT('',(0.327238813083405,0.124156188777542,0.36));
#35924=CARTESIAN_POINT('Ctrl Pts',(0.317616105825637,0.115602808444076,
0.372));
#35925=CARTESIAN_POINT('Ctrl Pts',(0.322343540495878,0.119804905177669,
0.366120462798035));
#35926=CARTESIAN_POINT('Ctrl Pts',(0.327238813083405,0.124156188777542,
0.36));
#35927=CARTESIAN_POINT('',(0.317616105825637,0.115602808444076,0.4));
#35928=CARTESIAN_POINT('',(0.327238813083405,0.124156188777542,0.18));
#35929=CARTESIAN_POINT('Origin',(0.372958854825584,0.114024964841867,0.4));
#35930=CARTESIAN_POINT('',(0.330485534147499,0.115235895966675,0.36));
#35931=CARTESIAN_POINT('Ctrl Pts',(0.330485534147499,0.115235895966675,
0.36));
#35932=CARTESIAN_POINT('Ctrl Pts',(0.323938586600038,0.115422552023493,
0.366120462798038));
#35933=CARTESIAN_POINT('Ctrl Pts',(0.317616105825637,0.115602808444076,
0.372));
#35934=CARTESIAN_POINT('',(0.330485534147499,0.115235895966675,0.18));
#35935=CARTESIAN_POINT('Origin',(0.258923021774215,0.21726221207405,0.4));
#35936=CARTESIAN_POINT('',(0.258923021774215,0.21726221207405,0.372));
#35937=CARTESIAN_POINT('',(0.265039980408751,0.228590920171666,0.36));
#35938=CARTESIAN_POINT('Ctrl Pts',(0.258923021774215,0.21726221207405,0.372));
#35939=CARTESIAN_POINT('Ctrl Pts',(0.261928155521996,0.222827769249914,
0.366120462798035));
#35940=CARTESIAN_POINT('Ctrl Pts',(0.265039980408751,0.228590920171666,
0.36));
#35941=CARTESIAN_POINT('',(0.258923021774215,0.21726221207405,0.4));
#35942=CARTESIAN_POINT('',(0.265039980408751,0.228590920171666,0.18));
#35943=CARTESIAN_POINT('Origin',(0.311467848918444,0.234707859029299,0.4));
#35944=CARTESIAN_POINT('',(0.27114182006011,0.221319030845725,0.36));
#35945=CARTESIAN_POINT('Ctrl Pts',(0.27114182006011,0.221319030845725,0.36));
#35946=CARTESIAN_POINT('Ctrl Pts',(0.264925861629781,0.219255242226412,
0.36612046279804));
#35947=CARTESIAN_POINT('Ctrl Pts',(0.258923021774215,0.21726221207405,0.372));
#35948=CARTESIAN_POINT('',(0.27114182006011,0.221319030845725,0.18));
#35949=CARTESIAN_POINT('Origin',(0.169,0.29271658647914,0.4));
#35950=CARTESIAN_POINT('',(0.169,0.29271658647914,0.372));
#35951=CARTESIAN_POINT('',(0.170873414523285,0.305454212950408,0.36));
#35952=CARTESIAN_POINT('Ctrl Pts',(0.169,0.29271658647914,0.372));
#35953=CARTESIAN_POINT('Ctrl Pts',(0.169920369344288,0.298974315762989,
0.366120462798037));
#35954=CARTESIAN_POINT('Ctrl Pts',(0.170873414523285,0.305454212950408,
0.36));
#35955=CARTESIAN_POINT('',(0.169,0.29271658647914,0.4));
#35956=CARTESIAN_POINT('',(0.170873414523285,0.305454212950408,0.18));
#35957=CARTESIAN_POINT('Origin',(0.212409223655861,0.327081521498715,0.4));
#35958=CARTESIAN_POINT('',(0.179094400846393,0.300707824283758,0.36));
#35959=CARTESIAN_POINT('Ctrl Pts',(0.179094400846393,0.300707824283758,
0.36));
#35960=CARTESIAN_POINT('Ctrl Pts',(0.17395916785767,0.296642514354079,0.366120462798043));
#35961=CARTESIAN_POINT('Ctrl Pts',(0.169,0.29271658647914,0.372));
#35962=CARTESIAN_POINT('',(0.179094400846393,0.300707824283758,0.18));
#35963=CARTESIAN_POINT('Origin',(0.0586930840514225,0.332865020518126,0.4));
#35964=CARTESIAN_POINT('',(0.0586930840514225,0.332865020518126,0.372));
#35965=CARTESIAN_POINT('',(0.0560969930232949,0.345475219623267,0.36));
#35966=CARTESIAN_POINT('Ctrl Pts',(0.0586930840514225,0.332865020518126,
0.372));
#35967=CARTESIAN_POINT('Ctrl Pts',(0.0574176788660923,0.339060147404083,
0.366120462798035));
#35968=CARTESIAN_POINT('Ctrl Pts',(0.0560969930232949,0.345475219623267,
0.36));
#35969=CARTESIAN_POINT('',(0.0586930840514225,0.332865020518126,0.4));
#35970=CARTESIAN_POINT('',(0.0560969930232949,0.345475219623267,0.18));
#35971=CARTESIAN_POINT('Origin',(0.0877309111941073,0.380004325266242,0.4));
#35972=CARTESIAN_POINT('',(0.0654455537387478,0.343826816138341,0.36));
#35973=CARTESIAN_POINT('Ctrl Pts',(0.0654455537387477,0.343826816138341,
0.36));
#35974=CARTESIAN_POINT('Ctrl Pts',(0.0620104310780447,0.338250321273407,
0.366120462798036));
#35975=CARTESIAN_POINT('Ctrl Pts',(0.0586930840514225,0.332865020518126,
0.372));
#35976=CARTESIAN_POINT('',(0.0654455537387478,0.343826816138341,0.18));
#35977=CARTESIAN_POINT('Origin',(-0.0586930840514224,0.332865020518126,
0.4));
#35978=CARTESIAN_POINT('',(-0.0586930840514225,0.332865020518126,0.372));
#35979=CARTESIAN_POINT('',(-0.0654455537387477,0.343826816138341,0.36));
#35980=CARTESIAN_POINT('Ctrl Pts',(-0.0586930840514225,0.332865020518126,
0.372));
#35981=CARTESIAN_POINT('Ctrl Pts',(-0.0620104310780444,0.338250321273406,
0.366120462798036));
#35982=CARTESIAN_POINT('Ctrl Pts',(-0.0654455537387477,0.343826816138341,
0.36));
#35983=CARTESIAN_POINT('',(-0.0586930840514224,0.332865020518126,0.4));
#35984=CARTESIAN_POINT('',(-0.0654455537387477,0.343826816138341,0.18));
#35985=CARTESIAN_POINT('Origin',(-0.0475290439280075,0.387092999140116,
0.4));
#35986=CARTESIAN_POINT('',(-0.0560969930232949,0.345475219623267,0.36));
#35987=CARTESIAN_POINT('Ctrl Pts',(-0.0560969930232949,0.345475219623267,
0.36));
#35988=CARTESIAN_POINT('Ctrl Pts',(-0.0574176788660933,0.339060147404078,
0.36612046279804));
#35989=CARTESIAN_POINT('Ctrl Pts',(-0.0586930840514225,0.332865020518126,
0.372));
#35990=CARTESIAN_POINT('',(-0.0560969930232949,0.345475219623267,0.18));
#35991=CARTESIAN_POINT('Origin',(-0.169,0.29271658647914,0.4));
#35992=CARTESIAN_POINT('',(-0.169,0.29271658647914,0.372));
#35993=CARTESIAN_POINT('',(-0.179094400846393,0.300707824283758,0.36));
#35994=CARTESIAN_POINT('Ctrl Pts',(-0.169,0.29271658647914,0.372));
#35995=CARTESIAN_POINT('Ctrl Pts',(-0.173959167857679,0.296642514354086,
0.366120462798031));
#35996=CARTESIAN_POINT('Ctrl Pts',(-0.179094400846393,0.300707824283758,
0.36));
#35997=CARTESIAN_POINT('',(-0.169,0.29271658647914,0.4));
#35998=CARTESIAN_POINT('',(-0.179094400846393,0.300707824283758,0.18));
#35999=CARTESIAN_POINT('Origin',(-0.177056294898423,0.347492544433463,0.4));
#36000=CARTESIAN_POINT('',(-0.170873414523285,0.305454212950408,0.36));
#36001=CARTESIAN_POINT('Ctrl Pts',(-0.170873414523285,0.305454212950408,
0.36));
#36002=CARTESIAN_POINT('Ctrl Pts',(-0.169920369344288,0.29897431576299,
0.366120462798036));
#36003=CARTESIAN_POINT('Ctrl Pts',(-0.169,0.29271658647914,0.372));
#36004=CARTESIAN_POINT('',(-0.170873414523285,0.305454212950408,0.18));
#36005=CARTESIAN_POINT('Origin',(-0.258923021774215,0.21726221207405,0.4));
#36006=CARTESIAN_POINT('',(-0.258923021774215,0.21726221207405,0.372));
#36007=CARTESIAN_POINT('',(-0.27114182006011,0.221319030845725,0.36));
#36008=CARTESIAN_POINT('Ctrl Pts',(-0.258923021774215,0.21726221207405,
0.372));
#36009=CARTESIAN_POINT('Ctrl Pts',(-0.264925861629786,0.219255242226414,
0.366120462798035));
#36010=CARTESIAN_POINT('Ctrl Pts',(-0.27114182006011,0.221319030845725,
0.36));
#36011=CARTESIAN_POINT('',(-0.258923021774215,0.21726221207405,0.4));
#36012=CARTESIAN_POINT('',(-0.27114182006011,0.221319030845725,0.18));
#36013=CARTESIAN_POINT('Origin',(-0.285227943631476,0.265979360424374,0.4));
#36014=CARTESIAN_POINT('',(-0.265039980408751,0.228590920171666,0.36));
#36015=CARTESIAN_POINT('Ctrl Pts',(-0.265039980408751,0.228590920171666,
0.36));
#36016=CARTESIAN_POINT('Ctrl Pts',(-0.261928155521995,0.222827769249914,
0.366120462798036));
#36017=CARTESIAN_POINT('Ctrl Pts',(-0.258923021774215,0.21726221207405,
0.372));
#36018=CARTESIAN_POINT('',(-0.265039980408751,0.228590920171666,0.18));
#36019=CARTESIAN_POINT('Origin',(-0.317616105825637,0.115602808444076,0.4));
#36020=CARTESIAN_POINT('',(-0.317616105825637,0.115602808444076,0.372));
#36021=CARTESIAN_POINT('',(-0.330485534147499,0.115235895966675,0.36));
#36022=CARTESIAN_POINT('Ctrl Pts',(-0.317616105825637,0.115602808444076,
0.372));
#36023=CARTESIAN_POINT('Ctrl Pts',(-0.323938586600037,0.115422552023493,
0.366120462798039));
#36024=CARTESIAN_POINT('Ctrl Pts',(-0.330485534147499,0.115235895966675,
0.36));
#36025=CARTESIAN_POINT('',(-0.317616105825637,0.115602808444076,0.4));
#36026=CARTESIAN_POINT('',(-0.330485534147499,0.115235895966675,0.18));
#36027=CARTESIAN_POINT('Origin',(-0.358996892846452,0.152385140110817,0.4));
#36028=CARTESIAN_POINT('',(-0.327238813083405,0.124156188777542,0.36));
#36029=CARTESIAN_POINT('Ctrl Pts',(-0.327238813083405,0.124156188777542,
0.36));
#36030=CARTESIAN_POINT('Ctrl Pts',(-0.322343540495877,0.119804905177667,
0.366120462798037));
#36031=CARTESIAN_POINT('Ctrl Pts',(-0.317616105825637,0.115602808444076,
0.372));
#36032=CARTESIAN_POINT('',(-0.327238813083405,0.124156188777542,0.18));
#36033=CARTESIAN_POINT('Origin',(0.338,0.,0.4));
#36034=CARTESIAN_POINT('',(0.338,0.,0.372));
#36035=CARTESIAN_POINT('',(0.349967815369678,0.00474638866665024,0.36));
#36036=CARTESIAN_POINT('Ctrl Pts',(0.338,0.,0.372));
#36037=CARTESIAN_POINT('Ctrl Pts',(0.34387953720196,0.00233180140890496,
0.36612046279804));
#36038=CARTESIAN_POINT('Ctrl Pts',(0.349967815369678,0.00474638866665021,
0.36));
#36039=CARTESIAN_POINT('',(0.338,0.,0.4));
#36040=CARTESIAN_POINT('',(0.349967815369678,0.00474638866665024,0.18));
#36041=CARTESIAN_POINT('Origin',(0.389465518554284,-0.0204110229347481,
0.4));
#36042=CARTESIAN_POINT('',(0.349967815369678,-0.00474638866665023,0.36));
#36043=CARTESIAN_POINT('Ctrl Pts',(0.349967815369678,-0.00474638866665021,
0.36));
#36044=CARTESIAN_POINT('Ctrl Pts',(0.343879537201961,-0.00233180140890561,
0.366120462798039));
#36045=CARTESIAN_POINT('Ctrl Pts',(0.338,0.,0.372));
#36046=CARTESIAN_POINT('',(0.349967815369678,-0.00474638866665023,0.18));
#36047=CARTESIAN_POINT('Origin',(-0.332865020518126,-0.0586930840514225,
0.4));
#36048=CARTESIAN_POINT('',(-0.332865020518126,-0.0586930840514225,0.372));
#36049=CARTESIAN_POINT('',(-0.343826816138341,-0.0654455537387478,0.36));
#36050=CARTESIAN_POINT('Ctrl Pts',(-0.332865020518126,-0.0586930840514225,
0.372));
#36051=CARTESIAN_POINT('Ctrl Pts',(-0.338250321273407,-0.062010431078045,
0.366120462798035));
#36052=CARTESIAN_POINT('Ctrl Pts',(-0.343826816138341,-0.0654455537387477,
0.36));
#36053=CARTESIAN_POINT('',(-0.332865020518126,-0.0586930840514225,0.4));
#36054=CARTESIAN_POINT('',(-0.343826816138341,-0.0654455537387478,0.18));
#36055=CARTESIAN_POINT('Origin',(-0.387092999140116,-0.0475290439280074,
0.4));
#36056=CARTESIAN_POINT('',(-0.345475219623267,-0.0560969930232949,0.36));
#36057=CARTESIAN_POINT('Ctrl Pts',(-0.345475219623267,-0.0560969930232949,
0.36));
#36058=CARTESIAN_POINT('Ctrl Pts',(-0.339060147404077,-0.0574176788660935,
0.366120462798041));
#36059=CARTESIAN_POINT('Ctrl Pts',(-0.332865020518126,-0.0586930840514225,
0.372));
#36060=CARTESIAN_POINT('',(-0.345475219623267,-0.0560969930232949,0.18));
#36061=CARTESIAN_POINT('Origin',(-0.29271658647914,-0.169,0.4));
#36062=CARTESIAN_POINT('',(-0.29271658647914,-0.169,0.372));
#36063=CARTESIAN_POINT('',(-0.300707824283758,-0.179094400846393,0.36));
#36064=CARTESIAN_POINT('Ctrl Pts',(-0.29271658647914,-0.169,0.372));
#36065=CARTESIAN_POINT('Ctrl Pts',(-0.296642514354083,-0.173959167857676,
0.366120462798036));
#36066=CARTESIAN_POINT('Ctrl Pts',(-0.300707824283758,-0.179094400846393,
0.36));
#36067=CARTESIAN_POINT('',(-0.29271658647914,-0.169,0.4));
#36068=CARTESIAN_POINT('',(-0.300707824283758,-0.179094400846393,0.18));
#36069=CARTESIAN_POINT('Origin',(-0.347492544433463,-0.177056294898423,
0.4));
#36070=CARTESIAN_POINT('',(-0.305454212950408,-0.170873414523285,0.36));
#36071=CARTESIAN_POINT('Ctrl Pts',(-0.305454212950408,-0.170873414523285,
0.36));
#36072=CARTESIAN_POINT('Ctrl Pts',(-0.298974315762994,-0.169920369344289,
0.366120462798032));
#36073=CARTESIAN_POINT('Ctrl Pts',(-0.29271658647914,-0.169,0.372));
#36074=CARTESIAN_POINT('',(-0.305454212950408,-0.170873414523285,0.18));
#36075=CARTESIAN_POINT('Origin',(-0.21726221207405,-0.258923021774215,0.4));
#36076=CARTESIAN_POINT('',(-0.21726221207405,-0.258923021774215,0.372));
#36077=CARTESIAN_POINT('',(-0.221319030845725,-0.27114182006011,0.36));
#36078=CARTESIAN_POINT('Ctrl Pts',(-0.21726221207405,-0.258923021774215,
0.372));
#36079=CARTESIAN_POINT('Ctrl Pts',(-0.219255242226414,-0.264925861629784,
0.366120462798037));
#36080=CARTESIAN_POINT('Ctrl Pts',(-0.221319030845725,-0.27114182006011,
0.36));
#36081=CARTESIAN_POINT('',(-0.21726221207405,-0.258923021774215,0.4));
#36082=CARTESIAN_POINT('',(-0.221319030845725,-0.27114182006011,0.18));
#36083=CARTESIAN_POINT('Origin',(-0.265979360424374,-0.285227943631476,
0.4));
#36084=CARTESIAN_POINT('',(-0.228590920171666,-0.265039980408751,0.36));
#36085=CARTESIAN_POINT('Ctrl Pts',(-0.228590920171666,-0.265039980408751,
0.36));
#36086=CARTESIAN_POINT('Ctrl Pts',(-0.222827769249914,-0.261928155521995,
0.366120462798036));
#36087=CARTESIAN_POINT('Ctrl Pts',(-0.21726221207405,-0.258923021774215,
0.372));
#36088=CARTESIAN_POINT('',(-0.228590920171666,-0.265039980408751,0.18));
#36089=CARTESIAN_POINT('Origin',(-0.115602808444076,-0.317616105825637,
0.4));
#36090=CARTESIAN_POINT('',(-0.115602808444076,-0.317616105825637,0.372));
#36091=CARTESIAN_POINT('',(-0.115235895966675,-0.330485534147499,0.36));
#36092=CARTESIAN_POINT('Ctrl Pts',(-0.115602808444076,-0.317616105825637,
0.372));
#36093=CARTESIAN_POINT('Ctrl Pts',(-0.115422552023493,-0.323938586600039,
0.366120462798037));
#36094=CARTESIAN_POINT('Ctrl Pts',(-0.115235895966675,-0.330485534147499,
0.36));
#36095=CARTESIAN_POINT('',(-0.115602808444076,-0.317616105825637,0.4));
#36096=CARTESIAN_POINT('',(-0.115235895966675,-0.330485534147499,0.18));
#36097=CARTESIAN_POINT('Origin',(-0.152385140110817,-0.358996892846452,
0.4));
#36098=CARTESIAN_POINT('',(-0.124156188777542,-0.327238813083405,0.36));
#36099=CARTESIAN_POINT('Ctrl Pts',(-0.124156188777541,-0.327238813083405,
0.36));
#36100=CARTESIAN_POINT('Ctrl Pts',(-0.119804905177672,-0.322343540495882,
0.366120462798031));
#36101=CARTESIAN_POINT('Ctrl Pts',(-0.115602808444076,-0.317616105825637,
0.372));
#36102=CARTESIAN_POINT('',(-0.124156188777542,-0.327238813083405,0.18));
#36103=CARTESIAN_POINT('Origin',(-6.20895927167708E-17,-0.338,0.4));
#36104=CARTESIAN_POINT('',(-6.20895927167708E-17,-0.338,0.372));
#36105=CARTESIAN_POINT('',(0.00474638866665021,-0.349967815369678,0.36));
#36106=CARTESIAN_POINT('Ctrl Pts',(-6.20895927167708E-17,-0.338,0.372));
#36107=CARTESIAN_POINT('Ctrl Pts',(0.00233180140890712,-0.343879537201965,
0.366120462798035));
#36108=CARTESIAN_POINT('Ctrl Pts',(0.00474638866665021,-0.349967815369678,
0.36));
#36109=CARTESIAN_POINT('',(-6.20895927167708E-17,-0.338,0.4));
#36110=CARTESIAN_POINT('',(0.00474638866665021,-0.349967815369678,0.18));
#36111=CARTESIAN_POINT('Origin',(-0.0204110229347483,-0.389465518554284,
0.4));
#36112=CARTESIAN_POINT('',(-0.00474638866665032,-0.349967815369678,0.36));
#36113=CARTESIAN_POINT('Ctrl Pts',(-0.00474638866665031,-0.349967815369678,
0.36));
#36114=CARTESIAN_POINT('Ctrl Pts',(-0.00233180140890634,-0.343879537201963,
0.366120462798037));
#36115=CARTESIAN_POINT('Ctrl Pts',(-6.20895927167708E-17,-0.338,0.372));
#36116=CARTESIAN_POINT('',(-0.00474638866665032,-0.349967815369678,0.18));
#36117=CARTESIAN_POINT('Origin',(0.115602808444076,-0.317616105825637,0.4));
#36118=CARTESIAN_POINT('',(0.115602808444076,-0.317616105825637,0.372));
#36119=CARTESIAN_POINT('',(0.124156188777542,-0.327238813083405,0.36));
#36120=CARTESIAN_POINT('Ctrl Pts',(0.115602808444076,-0.317616105825637,
0.372));
#36121=CARTESIAN_POINT('Ctrl Pts',(0.119804905177668,-0.322343540495877,
0.366120462798037));
#36122=CARTESIAN_POINT('Ctrl Pts',(0.124156188777542,-0.327238813083405,
0.36));
#36123=CARTESIAN_POINT('',(0.115602808444076,-0.317616105825637,0.4));
#36124=CARTESIAN_POINT('',(0.124156188777542,-0.327238813083405,0.18));
#36125=CARTESIAN_POINT('Origin',(0.114024964841867,-0.372958854825584,0.4));
#36126=CARTESIAN_POINT('',(0.115235895966675,-0.330485534147499,0.36));
#36127=CARTESIAN_POINT('Ctrl Pts',(0.115235895966675,-0.330485534147499,
0.36));
#36128=CARTESIAN_POINT('Ctrl Pts',(0.115422552023493,-0.323938586600039,
0.366120462798037));
#36129=CARTESIAN_POINT('Ctrl Pts',(0.115602808444076,-0.317616105825637,
0.372));
#36130=CARTESIAN_POINT('',(0.115235895966675,-0.330485534147499,0.18));
#36131=CARTESIAN_POINT('Origin',(0.21726221207405,-0.258923021774215,0.4));
#36132=CARTESIAN_POINT('',(0.21726221207405,-0.258923021774215,0.372));
#36133=CARTESIAN_POINT('',(0.228590920171666,-0.265039980408751,0.36));
#36134=CARTESIAN_POINT('Ctrl Pts',(0.21726221207405,-0.258923021774215,
0.372));
#36135=CARTESIAN_POINT('Ctrl Pts',(0.22282776924991,-0.261928155521994,
0.366120462798039));
#36136=CARTESIAN_POINT('Ctrl Pts',(0.228590920171666,-0.265039980408751,
0.36));
#36137=CARTESIAN_POINT('',(0.21726221207405,-0.258923021774215,0.4));
#36138=CARTESIAN_POINT('',(0.228590920171666,-0.265039980408751,0.18));
#36139=CARTESIAN_POINT('Origin',(0.234707859029299,-0.311467848918444,0.4));
#36140=CARTESIAN_POINT('',(0.221319030845725,-0.27114182006011,0.36));
#36141=CARTESIAN_POINT('Ctrl Pts',(0.221319030845725,-0.27114182006011,
0.36));
#36142=CARTESIAN_POINT('Ctrl Pts',(0.219255242226415,-0.264925861629789,
0.366120462798033));
#36143=CARTESIAN_POINT('Ctrl Pts',(0.21726221207405,-0.258923021774215,
0.372));
#36144=CARTESIAN_POINT('',(0.221319030845725,-0.27114182006011,0.18));
#36145=CARTESIAN_POINT('Origin',(0.29271658647914,-0.169,0.4));
#36146=CARTESIAN_POINT('',(0.29271658647914,-0.169,0.372));
#36147=CARTESIAN_POINT('',(0.305454212950408,-0.170873414523286,0.36));
#36148=CARTESIAN_POINT('Ctrl Pts',(0.29271658647914,-0.169,0.372));
#36149=CARTESIAN_POINT('Ctrl Pts',(0.298974315762989,-0.169920369344288,
0.366120462798037));
#36150=CARTESIAN_POINT('Ctrl Pts',(0.305454212950408,-0.170873414523285,
0.36));
#36151=CARTESIAN_POINT('',(0.29271658647914,-0.169,0.4));
#36152=CARTESIAN_POINT('',(0.305454212950408,-0.170873414523286,0.18));
#36153=CARTESIAN_POINT('Origin',(0.327081521498715,-0.212409223655861,0.4));
#36154=CARTESIAN_POINT('',(0.300707824283758,-0.179094400846393,0.36));
#36155=CARTESIAN_POINT('Ctrl Pts',(0.300707824283758,-0.179094400846393,
0.36));
#36156=CARTESIAN_POINT('Ctrl Pts',(0.296642514354083,-0.173959167857676,
0.366120462798036));
#36157=CARTESIAN_POINT('Ctrl Pts',(0.29271658647914,-0.169,0.372));
#36158=CARTESIAN_POINT('',(0.300707824283758,-0.179094400846393,0.18));
#36159=CARTESIAN_POINT('Origin',(0.332865020518126,-0.0586930840514225,
0.4));
#36160=CARTESIAN_POINT('',(0.332865020518126,-0.0586930840514225,0.372));
#36161=CARTESIAN_POINT('',(0.345475219623267,-0.0560969930232949,0.36));
#36162=CARTESIAN_POINT('Ctrl Pts',(0.332865020518126,-0.0586930840514225,
0.372));
#36163=CARTESIAN_POINT('Ctrl Pts',(0.339060147404081,-0.0574176788660926,
0.366120462798037));
#36164=CARTESIAN_POINT('Ctrl Pts',(0.345475219623267,-0.0560969930232949,
0.36));
#36165=CARTESIAN_POINT('',(0.332865020518126,-0.0586930840514225,0.4));
#36166=CARTESIAN_POINT('',(0.345475219623267,-0.0560969930232949,0.18));
#36167=CARTESIAN_POINT('Origin',(0.380004325266242,-0.0877309111941075,
0.4));
#36168=CARTESIAN_POINT('',(0.343826816138341,-0.0654455537387478,0.36));
#36169=CARTESIAN_POINT('Ctrl Pts',(0.343826816138341,-0.0654455537387478,
0.36));
#36170=CARTESIAN_POINT('Ctrl Pts',(0.338250321273404,-0.062010431078043,
0.366120462798039));
#36171=CARTESIAN_POINT('Ctrl Pts',(0.332865020518126,-0.0586930840514225,
0.372));
#36172=CARTESIAN_POINT('',(0.343826816138341,-0.0654455537387478,0.18));
#36173=CARTESIAN_POINT('Origin',(0.,0.,0.18));
#36174=CARTESIAN_POINT('Origin',(0.,0.,0.36));
#36175=CARTESIAN_POINT('Origin',(0.,0.,0.18));
#36176=CARTESIAN_POINT('Origin',(0.,0.,0.36));
#36177=CARTESIAN_POINT('Origin',(0.,0.,0.18));
#36178=CARTESIAN_POINT('Origin',(0.,0.,0.36));
#36179=CARTESIAN_POINT('Origin',(0.,0.,0.18));
#36180=CARTESIAN_POINT('Origin',(0.,0.,0.36));
#36181=CARTESIAN_POINT('Origin',(0.,0.,0.18));
#36182=CARTESIAN_POINT('Origin',(0.,0.,0.36));
#36183=CARTESIAN_POINT('Origin',(0.,0.,0.18));
#36184=CARTESIAN_POINT('Origin',(0.,0.,0.36));
#36185=CARTESIAN_POINT('Origin',(0.,0.,0.18));
#36186=CARTESIAN_POINT('Origin',(0.,0.,0.36));
#36187=CARTESIAN_POINT('Origin',(0.,0.,0.18));
#36188=CARTESIAN_POINT('Origin',(0.,0.,0.36));
#36189=CARTESIAN_POINT('Origin',(0.,0.,0.18));
#36190=CARTESIAN_POINT('Origin',(0.,0.,0.36));
#36191=CARTESIAN_POINT('Origin',(0.,0.,0.18));
#36192=CARTESIAN_POINT('Origin',(0.,0.,0.36));
#36193=CARTESIAN_POINT('Origin',(0.,0.,0.18));
#36194=CARTESIAN_POINT('Origin',(0.,0.,0.36));
#36195=CARTESIAN_POINT('Origin',(0.,0.,0.18));
#36196=CARTESIAN_POINT('Origin',(0.,0.,0.36));
#36197=CARTESIAN_POINT('Origin',(0.,0.,0.18));
#36198=CARTESIAN_POINT('Origin',(0.,0.,0.36));
#36199=CARTESIAN_POINT('Origin',(0.,0.,0.18));
#36200=CARTESIAN_POINT('Origin',(0.,0.,0.36));
#36201=CARTESIAN_POINT('Origin',(0.,0.,0.18));
#36202=CARTESIAN_POINT('Origin',(0.,0.,0.36));
#36203=CARTESIAN_POINT('Origin',(0.,0.,0.18));
#36204=CARTESIAN_POINT('Origin',(0.,0.,0.36));
#36205=CARTESIAN_POINT('Origin',(0.,0.,0.18));
#36206=CARTESIAN_POINT('Origin',(0.,0.,0.36));
#36207=CARTESIAN_POINT('Origin',(0.,0.,0.18));
#36208=CARTESIAN_POINT('Origin',(0.,0.,0.36));
#36209=CARTESIAN_POINT('Origin',(0.,0.,0.18));
#36210=CARTESIAN_POINT('Origin',(0.,0.,0.36));
#36211=CARTESIAN_POINT('Origin',(0.,0.,0.18));
#36212=CARTESIAN_POINT('Origin',(0.,0.,0.36));
#36213=CARTESIAN_POINT('Origin',(0.,0.,0.18));
#36214=CARTESIAN_POINT('Origin',(0.,0.,0.36));
#36215=CARTESIAN_POINT('Origin',(0.,0.,0.18));
#36216=CARTESIAN_POINT('Origin',(0.,0.,0.36));
#36217=CARTESIAN_POINT('Origin',(0.,0.,0.18));
#36218=CARTESIAN_POINT('Origin',(0.,0.,0.36));
#36219=CARTESIAN_POINT('Origin',(0.,0.,0.18));
#36220=CARTESIAN_POINT('Origin',(0.,0.,0.36));
#36221=CARTESIAN_POINT('Origin',(0.,0.,0.18));
#36222=CARTESIAN_POINT('Origin',(0.,0.,0.36));
#36223=CARTESIAN_POINT('Origin',(0.,0.,0.18));
#36224=CARTESIAN_POINT('Origin',(0.,0.,0.36));
#36225=CARTESIAN_POINT('Origin',(0.,0.,0.18));
#36226=CARTESIAN_POINT('Origin',(0.,0.,0.36));
#36227=CARTESIAN_POINT('Origin',(0.,0.,0.18));
#36228=CARTESIAN_POINT('Origin',(0.,0.,0.36));
#36229=CARTESIAN_POINT('Origin',(0.,0.,0.18));
#36230=CARTESIAN_POINT('Origin',(0.,0.,0.36));
#36231=CARTESIAN_POINT('Origin',(0.,0.,0.18));
#36232=CARTESIAN_POINT('Origin',(0.,0.,0.36));
#36233=CARTESIAN_POINT('Origin',(0.,0.,0.18));
#36234=CARTESIAN_POINT('Origin',(0.,0.,0.36));
#36235=CARTESIAN_POINT('Origin',(0.,0.,0.18));
#36236=CARTESIAN_POINT('Origin',(0.,0.,0.36));
#36237=CARTESIAN_POINT('Origin',(0.,0.,0.18));
#36238=CARTESIAN_POINT('Origin',(0.,0.,0.36));
#36239=CARTESIAN_POINT('Origin',(0.,0.,0.18));
#36240=CARTESIAN_POINT('Origin',(0.,0.,0.36));
#36241=CARTESIAN_POINT('Origin',(0.,0.,0.18));
#36242=CARTESIAN_POINT('Origin',(0.,0.,0.36));
#36243=CARTESIAN_POINT('Origin',(0.,0.,0.18));
#36244=CARTESIAN_POINT('Origin',(0.,0.,0.36));
#36245=CARTESIAN_POINT('Origin',(0.16,0.,-1.6));
#36246=CARTESIAN_POINT('',(-0.16,-1.95943487863577E-17,-1.6));
#36247=CARTESIAN_POINT('Origin',(0.,0.,-1.6));
#36248=CARTESIAN_POINT('Origin',(0.,0.,-1.58));
#36249=CARTESIAN_POINT('',(-0.18,-2.20436423846524E-17,-1.58));
#36250=CARTESIAN_POINT('Origin',(0.,0.,0.38));
#36251=CARTESIAN_POINT('',(-0.31,-3.7964050773568E-17,0.4));
#36252=CARTESIAN_POINT('Origin',(0.,0.,0.4));
#36253=CARTESIAN_POINT('',(-0.33,-4.04133443718627E-17,0.38));
#36254=CARTESIAN_POINT('Origin',(0.,0.,0.4));
#38593=UNCERTAINTY_MEASURE_WITH_UNIT(LENGTH_MEASURE(0.001),#38612,
'DISTANCE_ACCURACY_VALUE',
'Maximum model space distance between geometric entities at asserted c
onnectivities');
#38595=UNCERTAINTY_MEASURE_WITH_UNIT(LENGTH_MEASURE(0.001),#38612,
'DISTANCE_ACCURACY_VALUE',
'Maximum model space distance between geometric entities at asserted c
onnectivities');
#38609=(
GEOMETRIC_REPRESENTATION_CONTEXT(3)
GLOBAL_UNCERTAINTY_ASSIGNED_CONTEXT((#38593))
GLOBAL_UNIT_ASSIGNED_CONTEXT((#38612,#38614,#38615))
REPRESENTATION_CONTEXT('','3D')
);
#38611=(
GEOMETRIC_REPRESENTATION_CONTEXT(3)
GLOBAL_UNCERTAINTY_ASSIGNED_CONTEXT((#38595))
GLOBAL_UNIT_ASSIGNED_CONTEXT((#38612,#38614,#38615))
REPRESENTATION_CONTEXT('','3D')
);
#38612=(
LENGTH_UNIT()
NAMED_UNIT(*)
SI_UNIT(.CENTI.,.METRE.)
);
#38614=(
NAMED_UNIT(*)
PLANE_ANGLE_UNIT()
SI_UNIT($,.RADIAN.)
);
#38615=(
NAMED_UNIT(*)
SI_UNIT($,.STERADIAN.)
SOLID_ANGLE_UNIT()
);
#38629=SHAPE_DEFINITION_REPRESENTATION(#38644,#38680);
#38644=PRODUCT_DEFINITION_SHAPE('',$,#38696);
#38680=SHAPE_REPRESENTATION('',(#17332),#38609);
#38682=PRODUCT_DEFINITION_CONTEXT('part definition',#38729,'design');
#38696=PRODUCT_DEFINITION('2026-10-19-02-31-53-467',
'11_ISO_4762_M4x16_Preload_Screw',#38711,#38682);
#38711=PRODUCT_DEFINITION_FORMATION('',$,#38744);
#38729=APPLICATION_CONTEXT(
'Core Data for Automotive Mechanical Design Process');
#38730=PRODUCT_CONTEXT('part definition',#38729,'mechanical');
#38744=PRODUCT('2026-10-19-02-31-53-467',
'11_ISO_4762_M4x16_Preload_Screw',$,(#38730));
#38879=COLOUR_RGB('Black',0.12,0.14,0.17);
#38880=FILL_AREA_STYLE_COLOUR('',#38879);
#38881=FILL_AREA_STYLE('',(#38880));
#38882=SURFACE_STYLE_FILL_AREA(#38881);
#38883=SURFACE_SIDE_STYLE('',(#38882));
#38884=SURFACE_STYLE_USAGE(.BOTH.,#38883);
#38885=PRESENTATION_STYLE_ASSIGNMENT((#38884));
ENDSEC;
END-ISO-10303-21;
